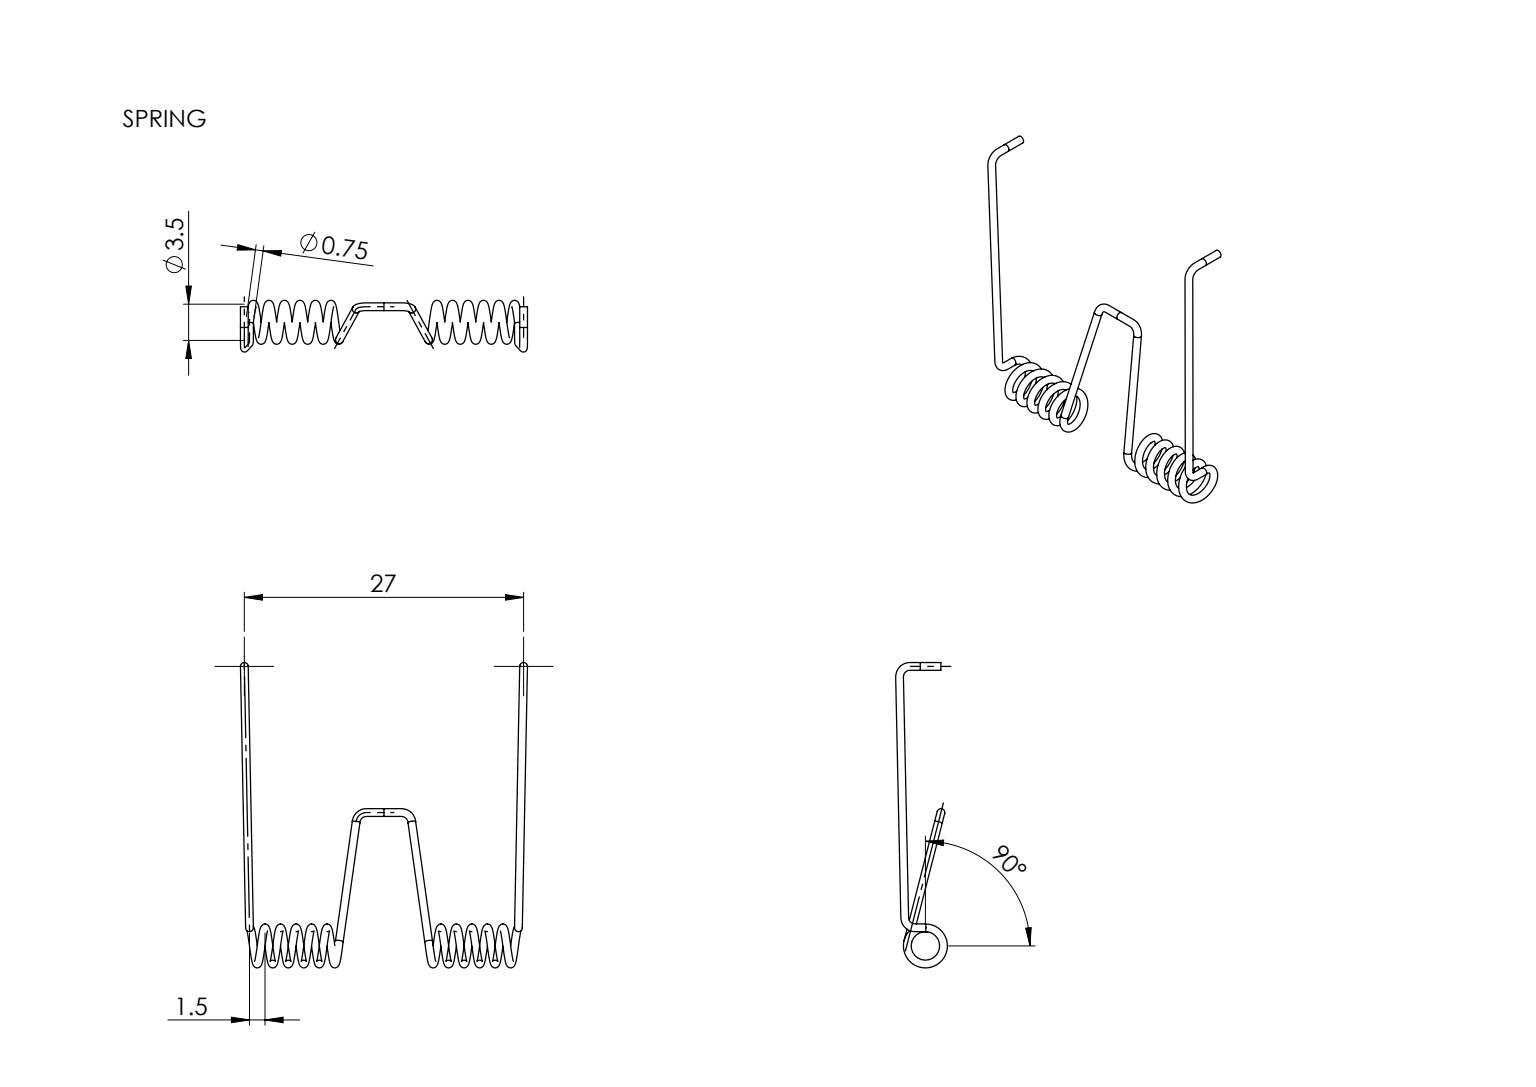
ISO-10303-21;
HEADER;
FILE_DESCRIPTION (('STEP AP214'),
    '1' );
FILE_NAME ('spring.step',
    '2026-10-04T16:38:04',
    ( '' ),
    ( '' ),
    'SwSTEP 2.0',
    'SolidWorks 2026',
    '' );
FILE_SCHEMA (( 'AUTOMOTIVE_DESIGN' ));
ENDSEC;

DATA;
#3=CARTESIAN_POINT ( 'NONE',  ( -13.45643611822145225, -15.38747602984844853, 4.825999963382285429 ) ) ;
#4=CARTESIAN_POINT ( 'NONE',  ( 8.871558582316794173, -20.24999999999999289, 3.449312527122348371 ) ) ;
#5=CARTESIAN_POINT ( 'NONE',  ( -12.62499963760179256, -21.00001830110826972, 4.442557003548452066 ) ) ;
#9=CARTESIAN_POINT ( 'NONE',  ( -8.309058582316795949, -23.80360840875935935, 1.768074502826626260 ) ) ;
#10=CARTESIAN_POINT ( 'NONE',  ( 8.496558582316794173, -22.05068747287764452, 1.749999999999998446 ) ) ;
#11=CARTESIAN_POINT ( 'NONE',  ( 4.097191417683177406, -22.46490103525075810, 4.479004561291653808 ) ) ;
#12=CARTESIAN_POINT ( 'NONE',  ( -6.621558582316794173, -23.74999999999999645, 3.550687472877651629 ) ) ;
#14=CARTESIAN_POINT ( 'NONE',  ( 13.82092246150448211, 3.019084305971233562, 5.221833296715730377 ) ) ;
#25=CARTESIAN_POINT ( 'NONE',  ( -1.548630333695928396, -9.114917468222230923, 2.372643865078341019 ) ) ;
#28=CARTESIAN_POINT ( 'NONE',  ( 2.506848361495492394, -9.459347215042898327, 1.711100304737409150 ) ) ;
#29=CARTESIAN_POINT ( 'NONE',  ( -13.10012427866737639, 3.743776072700027324, 6.001983176248468332 ) ) ;
#30=CARTESIAN_POINT ( 'NONE',  ( 9.715308582316794173, -23.77099543870833998, 2.825813738724734847 ) ) ;
#32=CARTESIAN_POINT ( 'NONE',  ( 13.15498530132288479, 5.764257716805535559, 4.666666666666618113 ) ) ;
#33=CARTESIAN_POINT ( 'NONE',  ( -1.797685059409938280, -9.880079706704160358, 1.626537830816663588 ) ) ;
#37=CARTESIAN_POINT ( 'NONE',  ( -13.85980676119184629, 4.232741440188380722, 5.965367510457697975 ) ) ;
#40=CARTESIAN_POINT ( 'NONE',  ( 5.972191417683178294, -24.47900456129165292, 2.413778621189595963 ) ) ;
#41=CARTESIAN_POINT ( 'NONE',  ( -6.534691417683177406, -20.97900456129164581, 3.136473910504570917 ) ) ;
#44=CARTESIAN_POINT ( 'NONE',  ( 13.90439735423812273, 5.734566389025032684, 4.166666666666765551 ) ) ;
#45=CARTESIAN_POINT ( 'NONE',  ( 13.11017182064853159, 4.251176942750957366, 5.979809059808775196 ) ) ;
#57=CARTESIAN_POINT ( 'NONE',  ( 2.097836924194969033, -11.64739567274323129, 2.830419876579102212 ) ) ;
#64=CARTESIAN_POINT ( 'NONE',  ( 11.77780858231679595, -21.02099543870833998, 3.035098964749253003 ) ) ;
#65=CARTESIAN_POINT ( 'NONE',  ( -13.08799567112409790, 3.881281391764801025, 5.254907606674271037 ) ) ;
#66=CARTESIAN_POINT ( 'NONE',  ( -5.309058582316795949, -22.74294823697954016, 2.828734674606448785 ) ) ;
#67=CARTESIAN_POINT ( 'NONE',  ( -12.25344141768317741, -21.94931252712233061, 1.749999999999998446 ) ) ;
#69=CARTESIAN_POINT ( 'NONE',  ( 13.09358652029869141, 4.163619275088517035, 5.207983256689002083 ) ) ;
#70=SURFACE_STYLE_USAGE ( .BOTH. , #17121 ) ;
#75=CARTESIAN_POINT ( 'NONE',  ( 13.37505392270939986, -20.99727690317663686, 4.612442573673130930 ) ) ;
#79=CARTESIAN_POINT ( 'NONE',  ( 10.19094141768317563, -23.27327832286946219, 4.701595411283453707 ) ) ;
#83=CARTESIAN_POINT ( 'NONE',  ( -2.583953725994688533, -9.847075946378776479, 2.560676788604062004 ) ) ;
#84=CARTESIAN_POINT ( 'NONE',  ( 2.702705060698113115, -10.69015907548275379, 2.777197378435510622 ) ) ;
#85=CARTESIAN_POINT ( 'NONE',  ( -10.65280858231679240, -21.22443879296942626, 5.229004561291660025 ) ) ;
#86=VECTOR ( 'NONE', #19310, 1000.000000000000114 ) ;
#88=CARTESIAN_POINT ( 'NONE',  ( 5.503441417683177406, -22.05068747287766229, 6.000000000000001776 ) ) ;
#90=CARTESIAN_POINT ( 'NONE',  ( -3.974842109207561425, -21.82955800590261575, 5.256404853634145447 ) ) ;
#92=CARTESIAN_POINT ( 'NONE',  ( 13.37155858231679595, -19.49999999999998934, 3.449312527122348371 ) ) ;
#94=CARTESIAN_POINT ( 'NONE',  ( -13.90439735423812273, 5.734566389025032684, 4.791666666666684726 ) ) ;
#97=CARTESIAN_POINT ( 'NONE',  ( 7.465308582316795061, -20.22900456129164937, 4.174186261275266929 ) ) ;
#105=CARTESIAN_POINT ( 'NONE',  ( -12.43405858231679595, -23.73192549717337130, 5.303608408759367343 ) ) ;
#106=CARTESIAN_POINT ( 'NONE',  ( 12.62499979224180180, -20.25001049178813162, 4.458178821399696012 ) ) ;
#108=CARTESIAN_POINT ( 'NONE',  ( 0.5631383031621635116, -9.114917468222230923, 1.622643865078341463 ) ) ;
#109=CARTESIAN_POINT ( 'NONE',  ( 12.62499999999998579, -20.24999999999999289, 3.666666666666653640 ) ) ;
#111=CARTESIAN_POINT ( 'NONE',  ( -13.37499999999998579, -20.24999999999999289, 3.146526952850934755 ) ) ;
#112=CARTESIAN_POINT ( 'NONE',  ( 7.840308582316794173, -22.67418626127525982, 5.270995438708342640 ) ) ;
#113=CARTESIAN_POINT ( 'NONE',  ( -13.89992416064626646, 5.508670112635706495, 5.888743936161951353 ) ) ;
#116=CARTESIAN_POINT ( 'NONE',  ( -10.74655858231679595, -21.94931252712234127, 6.000000000000001776 ) ) ;
#117=CARTESIAN_POINT ( 'NONE',  ( 4.840308582316793284, -22.67418626127525982, 5.270995438708342640 ) ) ;
#119=CARTESIAN_POINT ( 'NONE',  ( 8.503441417683177406, -22.05068747287766229, 4.499999999999999112 ) ) ;
#120=CARTESIAN_POINT ( 'NONE',  ( -9.815941417683177406, -20.79840458871654363, 4.773278322869464851 ) ) ;
#123=CARTESIAN_POINT ( 'NONE',  ( 13.80173896975277437, 2.050317972508536535, 5.200999963382010094 ) ) ;
#125=CARTESIAN_POINT ( 'NONE',  ( 2.693754455098655409, -10.04853567022903782, 2.237415670251142519 ) ) ;
#132=CARTESIAN_POINT ( 'NONE',  ( -2.076833265075072266, -8.407161531158021006, 2.383492984350220389 ) ) ;
#133=CARTESIAN_POINT ( 'NONE',  ( 0.2815691515810352930, -9.114917468222230923, 2.372643865078523984 ) ) ;
#135=CARTESIAN_POINT ( 'NONE',  ( -13.09532840572934376, 3.501584489333809724, 5.996774842915142401 ) ) ;
#138=CARTESIAN_POINT ( 'NONE',  ( 13.12175473207386922, 4.086113969730903683, 6.756475741440692850 ) ) ;
#139=CARTESIAN_POINT ( 'NONE',  ( -1.982945319006538032, -10.83166796549307520, 2.620924705558935308 ) ) ;
#141=CARTESIAN_POINT ( 'NONE',  ( -13.37499999998404299, -20.99999999996810729, 2.793053905886972998 ) ) ;
#143=CARTESIAN_POINT ( 'NONE',  ( 5.878441417683177406, -24.50000000000000000, 3.449312527122335048 ) ) ;
#144=CARTESIAN_POINT ( 'NONE',  ( -6.809058582316796837, -22.74294823697954016, 2.828734674606448785 ) ) ;
#146=CARTESIAN_POINT ( 'NONE',  ( 12.62608183053121458, -20.94536755816881168, 4.949360998036265613 ) ) ;
#147=CARTESIAN_POINT ( 'NONE',  ( 13.10557919622060652, 4.019249409169220577, 6.007898877577752650 ) ) ;
#158=CARTESIAN_POINT ( 'NONE',  ( 0.2815691515810352374, -9.864917468222230923, 1.622643865078524428 ) ) ;
#163=CARTESIAN_POINT ( 'NONE',  ( -11.12155858231679417, -23.74999999999999645, 3.550687472877651629 ) ) ;
#164=CARTESIAN_POINT ( 'NONE',  ( -13.09734501894798342, -20.62502179913553846, 3.486720336327766567 ) ) ;
#165=CARTESIAN_POINT ( 'NONE',  ( -13.08559773465513487, 3.760185600081874746, 5.252303440007609403 ) ) ;
#166=CARTESIAN_POINT ( 'NONE',  ( -10.84030858231679240, -22.67418626127525982, 5.270995438708342640 ) ) ;
#167=CARTESIAN_POINT ( 'NONE',  ( -8.784691417683177406, -23.77099543870834353, 4.174186261275252718 ) ) ;
#169=CARTESIAN_POINT ( 'NONE',  ( 13.37893135632597819, -19.30146650553847465, 4.738802066438188909 ) ) ;
#178=CARTESIAN_POINT ( 'NONE',  ( 9.628441417683177406, -20.24999999999999289, 3.550687472877664952 ) ) ;
#181=CARTESIAN_POINT ( 'NONE',  ( -1.710927537542899612, -9.866086492083725901, 2.372944093759576933 ) ) ;
#182=CARTESIAN_POINT ( 'NONE',  ( 2.659620708751979645, -10.38426118526329489, 2.698636689302993830 ) ) ;
#183=CARTESIAN_POINT ( 'NONE',  ( -11.87155858231679417, -20.24999999999999289, 3.449312527122348371 ) ) ;
#186=CARTESIAN_POINT ( 'NONE',  ( 7.190941417683176518, -23.27327832286946219, 4.701595411283453707 ) ) ;
#188=CARTESIAN_POINT ( 'NONE',  ( -6.253441417683176518, -21.94931252712233061, 1.749999999999998446 ) ) ;
#190=CARTESIAN_POINT ( 'NONE',  ( 11.30905858231679595, -23.80360840875935935, 1.768074502826626260 ) ) ;
#191=CARTESIAN_POINT ( 'NONE',  ( 12.64387510712649565, -19.29680709011273976, 5.506486987317513737 ) ) ;
#192=CARTESIAN_POINT ( 'NONE',  ( -12.62562019941893432, -20.21867992933967173, 4.757612834768309540 ) ) ;
#199=SHAPE_DEFINITION_REPRESENTATION ( #15847, #6045 ) ;
#203=CARTESIAN_POINT ( 'NONE',  ( -7.277808582316794173, -20.27099543870833642, 2.724438792969431589 ) ) ;
#206=CARTESIAN_POINT ( 'NONE',  ( 2.022757268986824730, -10.07035769906783784, 1.675405020440470238 ) ) ;
#207=CARTESIAN_POINT ( 'NONE',  ( 12.65410809543883985, -18.78004118034163739, 5.517608176248461227 ) ) ;
#209=CARTESIAN_POINT ( 'NONE',  ( -13.39169183355864590, -18.65706240528901105, 4.755687463382285429 ) ) ;
#210=CARTESIAN_POINT ( 'NONE',  ( 8.777808582316797725, -19.52099543870833642, 2.413778621189609286 ) ) ;
#211=CARTESIAN_POINT ( 'NONE',  ( -12.62500000000001954, -20.24999999999450040, 3.833333333368183382 ) ) ;
#213=CARTESIAN_POINT ( 'NONE',  ( 5.215308582316793284, -23.77099543870833998, 2.825813738724734847 ) ) ;
#214=CARTESIAN_POINT ( 'NONE',  ( 4.565941417683176518, -22.67126532539353789, 2.757051763020445634 ) ) ;
#215=CARTESIAN_POINT ( 'NONE',  ( -5.409691417683177406, -21.32581373872474373, 5.270995438708348857 ) ) ;
#218=CARTESIAN_POINT ( 'NONE',  ( 13.82811627091129836, 3.382371681020614584, 5.229645796715683304 ) ) ;
#224=CARTESIAN_POINT ( 'NONE',  ( -13.12529397354238192, 5.014845663890295846, 4.833333333333344584 ) ) ;
#225=CARTESIAN_POINT ( 'NONE',  ( -1.513434189748285918, -8.364917468222230923, 1.622643865078341907 ) ) ;
#229=CARTESIAN_POINT ( 'NONE',  ( -12.64323021897839006, -19.32937394158751943, 5.504219675487169283 ) ) ;
#232=CARTESIAN_POINT ( 'NONE',  ( 12.70700162295422864, -16.85891804079483691, 6.308954579156044851 ) ) ;
#233=CARTESIAN_POINT ( 'NONE',  ( -2.097836924194969033, -11.64739567274323129, 2.830419876579102212 ) ) ;
#236=CARTESIAN_POINT ( 'NONE',  ( -13.70116456325478893, -3.778689555664588973, 5.825679699621801433 ) ) ;
#238=CARTESIAN_POINT ( 'NONE',  ( 6.534691417683177406, -19.47900456129164581, 2.515153566944927199 ) ) ;
#239=CARTESIAN_POINT ( 'NONE',  ( -5.027808582316795949, -22.97900456129165647, 3.964901035250747885 ) ) ;
#241=CARTESIAN_POINT ( 'NONE',  ( 13.87372783958217681, 4.185755898898970706, 6.732634959205082481 ) ) ;
#242=CARTESIAN_POINT ( 'NONE',  ( 12.95145221759166354, -3.764163011652346569, 5.840524842913703552 ) ) ;
#249=DIRECTION ( 'NONE',  ( 0.000000000000000000, 0.2487476929738665354, 0.9685683172808094987 ) ) ;
#250=CARTESIAN_POINT ( 'NONE',  ( 1.337453470010121714, -9.864917468222230923, 1.622643865078341907 ) ) ;
#257=CARTESIAN_POINT ( 'NONE',  ( -10.84030858231679240, -22.67418626127525982, 5.270995438708342640 ) ) ;
#258=CARTESIAN_POINT ( 'NONE',  ( -1.548630333695928396, -9.114917468222230923, 2.372643865078341019 ) ) ;
#260=CARTESIAN_POINT ( 'NONE',  ( -12.62837453896009876, -19.32958578251692572, 4.742959489302074338 ) ) ;
#261=CARTESIAN_POINT ( 'NONE',  ( -6.059058582316795949, -21.25705176302045274, 4.171265325393551215 ) ) ;
#262=CARTESIAN_POINT ( 'NONE',  ( -4.284691417683176518, -23.77099543870834353, 4.174186261275252718 ) ) ;
#265=CARTESIAN_POINT ( 'NONE',  ( 13.80173896975277437, 2.050317972508536535, 5.200999963382010094 ) ) ;
#275=CARTESIAN_POINT ( 'NONE',  ( 9.815941417683177406, -20.79840458871654363, 4.773278322869464851 ) ) ;
#277=CARTESIAN_POINT ( 'NONE',  ( -1.853238653218509890, -9.965882697426144077, 2.398573752920997837 ) ) ;
#279=CARTESIAN_POINT ( 'NONE',  ( -9.340308582316794173, -22.67418626127525982, 5.270995438708342640 ) ) ;
#284=CARTESIAN_POINT ( 'NONE',  ( 10.56594141768317741, -23.20159541128344927, 2.226721677130534705 ) ) ;
#286=CARTESIAN_POINT ( 'NONE',  ( -11.59719141768317741, -22.46490103525075810, 4.479004561291653808 ) ) ;
#288=CARTESIAN_POINT ( 'NONE',  ( 11.68405858231679595, -20.26807450282662160, 1.696391591240633101 ) ) ;
#290=CARTESIAN_POINT ( 'NONE',  ( 12.64131715375063258, -19.42598373559290792, 5.491151580003103660 ) ) ;
#291=CARTESIAN_POINT ( 'NONE',  ( -13.15498530132288479, 5.764257716805535559, 4.791666666666684726 ) ) ;
#299=PRESENTATION_STYLE_ASSIGNMENT (( #17872 ) ) ;
#300=ORIENTED_EDGE ( 'NONE', *, *, #6043, .F. ) ;
#303=CARTESIAN_POINT ( 'NONE',  ( 12.87800906051949390, -19.89203723036131066, 3.516308674092069708 ) ) ;
#307=CARTESIAN_POINT ( 'NONE',  ( -6.809058582316794173, -23.27327832286945153, 2.298404588716537411 ) ) ;
#308=CARTESIAN_POINT ( 'NONE',  ( 13.12463908936614132, 4.981774012991869505, 5.264611377988129171 ) ) ;
#311=CARTESIAN_POINT ( 'NONE',  ( 12.62499999999998401, -20.24999999999998934, 2.439580858552613751 ) ) ;
#313=CARTESIAN_POINT ( 'NONE',  ( -13.53317008522746434, -11.51241069598931510, 4.909333296715523431 ) ) ;
#316=CARTESIAN_POINT ( 'NONE',  ( 7.559058582316795949, -20.19639159124062999, 5.231925497173373074 ) ) ;
#317=CARTESIAN_POINT ( 'NONE',  ( -13.15498530132288479, 5.764257716805535559, 3.666666666666500873 ) ) ;
#318=CARTESIAN_POINT ( 'NONE',  ( -10.00344141768317741, -22.05068747287766229, 6.000000000000001776 ) ) ;
#322=CARTESIAN_POINT ( 'NONE',  ( 10.93405858231679595, -22.67126532539354855, 4.242948236979545484 ) ) ;
#323=CARTESIAN_POINT ( 'NONE',  ( -6.722191417683176518, -20.27099543870833998, 4.275561207030583510 ) ) ;
#326=CARTESIAN_POINT ( 'NONE',  ( 13.37883250981221472, -20.05645825448334563, 5.102688967256983510 ) ) ;
#334=CARTESIAN_POINT ( 'NONE',  ( 13.66279757975024722, -5.716222222589476765, 5.784013032957989964 ) ) ;
#341=CARTESIAN_POINT ( 'NONE',  ( -13.10756170493883310, 4.119366099410778581, 6.001761809183453700 ) ) ;
#342=CARTESIAN_POINT ( 'NONE',  ( 5.309058582316794173, -23.27327832286945153, 2.298404588716537411 ) ) ;
#344=CARTESIAN_POINT ( 'NONE',  ( 12.65650603190776025, -18.65894538865861563, 5.520212342915047365 ) ) ;
#345=CARTESIAN_POINT ( 'NONE',  ( -0.2815691515810352374, -9.864917468222230923, 2.372643865078523540 ) ) ;
#347=CARTESIAN_POINT ( 'NONE',  ( -13.39902456816392906, -19.03675930772010361, 5.497554699623231400 ) ) ;
#349=CARTESIAN_POINT ( 'NONE',  ( 10.09719141768317741, -22.77556120703057729, 5.229004561291655584 ) ) ;
#350=CARTESIAN_POINT ( 'NONE',  ( -7.371558582316795949, -20.99999999999999645, 3.449312527122348371 ) ) ;
#352=CARTESIAN_POINT ( 'NONE',  ( 13.87486364728600208, 4.243114187942282456, 6.725269602253773016 ) ) ;
#353=CARTESIAN_POINT ( 'NONE',  ( 12.66849571425264287, -18.05346643024382303, 5.533233176248494978 ) ) ;
#364=CARTESIAN_POINT ( 'NONE',  ( 1.711347482507859397, -9.865394108634699677, 1.622766275858107621 ) ) ;
#371=CARTESIAN_POINT ( 'NONE',  ( -9.059058582316794173, -20.72672167713054137, 4.701595411283463477 ) ) ;
#373=CARTESIAN_POINT ( 'NONE',  ( -0.5631383031621635116, -9.114917468222230923, 2.372643865078341019 ) ) ;
#375=CARTESIAN_POINT ( 'NONE',  ( -12.62499994688180749, -19.50000268246798640, 4.473800639250938183 ) ) ;
#376=CARTESIAN_POINT ( 'NONE',  ( -10.37155858231679417, -20.24999999999999289, 3.449312527122348371 ) ) ;
#377=CARTESIAN_POINT ( 'NONE',  ( -7.284691417683176518, -23.77099543870834353, 4.174186261275252718 ) ) ;
#379=CARTESIAN_POINT ( 'NONE',  ( 13.37930517931174634, -19.28258844475809042, 4.742233558278135419 ) ) ;
#389=CARTESIAN_POINT ( 'NONE',  ( 6.909691417683177406, -21.32581373872474373, 5.270995438708348857 ) ) ;
#391=CARTESIAN_POINT ( 'NONE',  ( -1.707060460004204527, -9.864918773552613374, 2.372644200313257290 ) ) ;
#393=CARTESIAN_POINT ( 'NONE',  ( -7.840308582316794173, -22.67418626127525982, 5.270995438708342640 ) ) ;
#395=CARTESIAN_POINT ( 'NONE',  ( 8.690941417683177406, -23.27327832286946219, 4.701595411283453707 ) ) ;
#397=CARTESIAN_POINT ( 'NONE',  ( -10.47219141768317741, -22.97900456129165292, 3.035098964749240125 ) ) ;
#400=CARTESIAN_POINT ( 'NONE',  ( 9.621558582316795949, -24.50000000000000000, 3.550687472877651629 ) ) ;
#401=CARTESIAN_POINT ( 'NONE',  ( 13.09532840572934376, 3.501584489333809724, 5.996774842915142401 ) ) ;
#402=CARTESIAN_POINT ( 'NONE',  ( -13.15498530132288479, 5.764257716805535559, 4.333333333333380999 ) ) ;
#410=CARTESIAN_POINT ( 'NONE',  ( 13.24164500767265729, -19.96139048183125198, 3.467035629977988975 ) ) ;
#414=CARTESIAN_POINT ( 'NONE',  ( 13.05696142222617695, 1.564051822406025583, 5.955108176248398166 ) ) ;
#418=CARTESIAN_POINT ( 'NONE',  ( 13.15498501280115917, 5.764243146453090105, 5.045733045595949484 ) ) ;
#419=CARTESIAN_POINT ( 'NONE',  ( 4.315753587183824180, -21.65797192216093947, 4.831781436261117335 ) ) ;
#420=CARTESIAN_POINT ( 'NONE',  ( -13.37499979530394967, -20.25001033714808329, 4.458488164327452097 ) ) ;
#421=CARTESIAN_POINT ( 'NONE',  ( 9.715308582316795949, -24.52099543870834708, 2.515153566944913432 ) ) ;
#423=CARTESIAN_POINT ( 'NONE',  ( -13.14123030749026277, 5.069630528265579805, 6.418963484850015000 ) ) ;
#424=CARTESIAN_POINT ( 'NONE',  ( -12.44094141768317741, -20.19639159124061933, 1.768074502826635586 ) ) ;
#426=CARTESIAN_POINT ( 'NONE',  ( 3.944195004867014909, -21.61378581760806128, 5.207602947182413011 ) ) ;
#428=CARTESIAN_POINT ( 'NONE',  ( 10.84030858231679595, -22.36352608949544418, 4.520995438708343528 ) ) ;
#429=CARTESIAN_POINT ( 'NONE',  ( -7.284691417683176518, -23.77099543870834353, 4.174186261275251830 ) ) ;
#432=CARTESIAN_POINT ( 'NONE',  ( 13.84501469867711698, 4.235742283194553259, 4.791666666666684726 ) ) ;
#436=ADVANCED_FACE ( 'NONE', ( #18652 ), #4141, .F. ) ;
#439=CARTESIAN_POINT ( 'NONE',  ( 13.84983662433050178, 3.729249528687784920, 5.987138032956566214 ) ) ;
#441=CARTESIAN_POINT ( 'NONE',  ( 3.767139617958116471, -12.99583330722436791, 3.561955564372631500 ) ) ;
#444=CARTESIAN_POINT ( 'NONE',  ( -12.62746768552656285, -19.37538188090202596, 4.723115281690125400 ) ) ;
#445=CARTESIAN_POINT ( 'NONE',  ( 8.496558582316794173, -22.05068747287764452, 1.749999999999998446 ) ) ;
#447=CARTESIAN_POINT ( 'NONE',  ( 13.08573665985359824, 3.017201322601628100, 5.986358176248492313 ) ) ;
#449=CARTESIAN_POINT ( 'NONE',  ( -2.875042468481914248, -11.91375063635796039, 3.091440134965714126 ) ) ;
#450=CARTESIAN_POINT ( 'NONE',  ( 10.55905858231679595, -21.25705176302045274, 4.171265325393551215 ) ) ;
#451=CARTESIAN_POINT ( 'NONE',  ( 9.628441417683177406, -20.24999999999999289, 3.550687472877664952 ) ) ;
#453=CARTESIAN_POINT ( 'NONE',  ( -7.090308582316795061, -21.63647391050454871, 2.479004561291657804 ) ) ;
#455=CARTESIAN_POINT ( 'NONE',  ( 13.88045627189955233, 4.525541730927888473, 6.662882075361062029 ) ) ;
#456=CARTESIAN_POINT ( 'NONE',  ( 13.10372118337080849, 3.925419760224517329, 6.005889426248455010 ) ) ;
#468=CARTESIAN_POINT ( 'NONE',  ( 0.000000000000000000, -9.114917468222230923, 1.622643865078341019 ) ) ;
#472=CARTESIAN_POINT ( 'NONE',  ( 13.36732475835166234, -20.34061592879088920, 3.450098321863545703 ) ) ;
#473=CARTESIAN_POINT ( 'NONE',  ( -2.436080212393455735, -9.483920418190111334, 2.467411194204634839 ) ) ;
#474=CARTESIAN_POINT ( 'NONE',  ( -8.871558582316794173, -20.24999999999999289, 3.449312527122348371 ) ) ;
#475=CARTESIAN_POINT ( 'NONE',  ( -3.034277558025862298, -9.029550313327863620, 2.543334857076493094 ) ) ;
#477=CARTESIAN_POINT ( 'NONE',  ( -12.62506359033936754, -19.49678868786235597, 4.541393094775662220 ) ) ;
#478=CARTESIAN_POINT ( 'NONE',  ( -5.871558582316794173, -20.24999999999999289, 3.449312527122348371 ) ) ;
#479=CARTESIAN_POINT ( 'NONE',  ( -5.972191417683179182, -23.72900456129165292, 2.724438792969417822 ) ) ;
#481=CARTESIAN_POINT ( 'NONE',  ( 13.84485691484488257, 4.227774199669918964, 5.063753864839139140 ) ) ;
#488=CARTESIAN_POINT ( 'NONE',  ( 5.690941417683176518, -23.27327832286946219, 4.701595411283453707 ) ) ;
#492=EDGE_CURVE ( 'NONE', #1847, #19275, #12685, .T. ) ;
#494=CARTESIAN_POINT ( 'NONE',  ( 11.03469141768318273, -20.22900456129164581, 2.825813738724747726 ) ) ;
#496=CARTESIAN_POINT ( 'NONE',  ( -8.878441417683177406, -22.99999999999999645, 3.449312527122335048 ) ) ;
#497=CARTESIAN_POINT ( 'NONE',  ( -8.965308582316795949, -19.47900456129164937, 4.484846433055089676 ) ) ;
#499=CARTESIAN_POINT ( 'NONE',  ( 12.62499999998404121, -20.24999999996810729, 2.793053905886972998 ) ) ;
#500=CARTESIAN_POINT ( 'NONE',  ( -13.15469878640066526, 5.749788713235649773, 5.232478742873432509 ) ) ;
#507=CARTESIAN_POINT ( 'NONE',  ( 2.592143777221601386, -9.905122062175031772, 2.575584190728205325 ) ) ;
#512=CARTESIAN_POINT ( 'NONE',  ( 13.12529380813666435, 5.014837310896125722, 5.033295791462342628 ) ) ;
#515=CARTESIAN_POINT ( 'NONE',  ( 12.91308523408712183, -5.701695678577235249, 5.798858176249892082 ) ) ;
#517=CARTESIAN_POINT ( 'NONE',  ( 7.184058582316795949, -20.26807450282662160, 1.696391591240633101 ) ) ;
#518=CARTESIAN_POINT ( 'NONE',  ( -13.15498530132288479, 5.764257716805535559, 4.166666666666765551 ) ) ;
#519=CARTESIAN_POINT ( 'NONE',  ( -4.687312169500634340, -21.32903648725300272, 5.908812401261035241 ) ) ;
#524=CARTESIAN_POINT ( 'NONE',  ( 8.309058582316795949, -22.74294823697954016, 2.828734674606448785 ) ) ;
#529=CARTESIAN_POINT ( 'NONE',  ( 13.39542766346049518, -19.21840299524461315, 5.493648449623241170 ) ) ;
#536=CARTESIAN_POINT ( 'NONE',  ( 13.83544900551672185, 3.002674778589386140, 5.971513032956590195 ) ) ;
#539=CARTESIAN_POINT ( 'NONE',  ( 1.797604806073912709, -9.120796646272857799, 2.374153755450133740 ) ) ;
#540=CARTESIAN_POINT ( 'NONE',  ( 1.652577328807104839, -9.114908150887895744, 1.622641472200749835 ) ) ;
#541=CARTESIAN_POINT ( 'NONE',  ( -12.93692567357942202, -3.747753484270499591, 5.090845106672844622 ) ) ;
#542=CARTESIAN_POINT ( 'NONE',  ( 7.840308582316794173, -22.67418626127525982, 5.270995438708342640 ) ) ;
#544=CARTESIAN_POINT ( 'NONE',  ( 13.11514659413808737, 4.502403003978772134, 5.887634658581065494 ) ) ;
#546=CARTESIAN_POINT ( 'NONE',  ( -1.548630333695928396, -9.114917468222230923, 2.372643865078341019 ) ) ;
#547=CARTESIAN_POINT ( 'NONE',  ( 6.902808582316795949, -22.46490103525074034, 2.520995438708341307 ) ) ;
#549=CARTESIAN_POINT ( 'NONE',  ( 8.128441417683175629, -20.24999999999999289, 3.550687472877664952 ) ) ;
#550=CARTESIAN_POINT ( 'NONE',  ( -10.18405858231679595, -21.32873467460644079, 2.757051763020455404 ) ) ;
#552=CARTESIAN_POINT ( 'NONE',  ( 13.11345185444515415, 3.666818649476655700, 6.750360829155977349 ) ) ;
#554=CARTESIAN_POINT ( 'NONE',  ( 13.09123688038123490, 4.044962459253448550, 5.255034774807352704 ) ) ;
#563=CARTESIAN_POINT ( 'NONE',  ( 3.277163086644854229, -14.76879761173520578, 3.824673233536266537 ) ) ;
#564=LINE ( 'NONE', #11752, #7741 ) ;
#569=CARTESIAN_POINT ( 'NONE',  ( -9.246558582316794173, -21.94931252712234482, 5.250000000000000888 ) ) ;
#571=CARTESIAN_POINT ( 'NONE',  ( -3.451187703687236041, -10.75258211228477734, 2.985843844067104680 ) ) ;
#573=CARTESIAN_POINT ( 'NONE',  ( -13.09560269887985307, 4.265436293439658577, 4.973800642626965640 ) ) ;
#575=CARTESIAN_POINT ( 'NONE',  ( -5.409691417683178294, -21.32581373872474373, 5.270995438708348857 ) ) ;
#577=CARTESIAN_POINT ( 'NONE',  ( 13.39169183355864590, -18.65706240528901105, 4.755687463382285429 ) ) ;
#589=CARTESIAN_POINT ( 'NONE',  ( 1.728780693989796724, -8.364929292255887106, 2.372646901726390478 ) ) ;
#590=CARTESIAN_POINT ( 'NONE',  ( -5.965308582316793284, -20.22900456129164937, 4.174186261275266929 ) ) ;
#592=CARTESIAN_POINT ( 'NONE',  ( 12.66863463945108137, -18.79645070772368953, 6.267287912489321045 ) ) ;
#595=CARTESIAN_POINT ( 'NONE',  ( 4.284691417683176518, -23.77099543870834353, 4.174186261275252718 ) ) ;
#597=CARTESIAN_POINT ( 'NONE',  ( -9.628441417683177406, -20.99999999999999645, 3.550687472877664952 ) ) ;
#598=CARTESIAN_POINT ( 'NONE',  ( -6.434058582316796837, -23.73192549717337130, 5.303608408759367343 ) ) ;
#600=CARTESIAN_POINT ( 'NONE',  ( 12.79798428357658047, -11.51429367935891790, 5.673858176248284479 ) ) ;
#601=CARTESIAN_POINT ( 'NONE',  ( -13.11345185444515415, 3.666818649476655700, 6.750360829155977349 ) ) ;
#602=ORIENTED_EDGE ( 'NONE', *, *, #19126, .F. ) ;
#609=CARTESIAN_POINT ( 'NONE',  ( 12.79327455738548203, -19.93647458090189772, 3.527980527292456259 ) ) ;
#612=CARTESIAN_POINT ( 'NONE',  ( 0.000000000000000000, -9.114917468222230923, 1.622643865078341019 ) ) ;
#614=CARTESIAN_POINT ( 'NONE',  ( -1.960495238260606010, -8.383787449798761671, 1.627490053312942164 ) ) ;
#619=CARTESIAN_POINT ( 'NONE',  ( 9.527808582316795949, -24.47900456129166358, 4.586221378810390270 ) ) ;
#620=CARTESIAN_POINT ( 'NONE',  ( -13.12405442816082868, 4.202248622120948518, 6.747400073346936367 ) ) ;
#621=CARTESIAN_POINT ( 'NONE',  ( -7.472191417683177406, -24.47900456129165292, 2.413778621189595963 ) ) ;
#626=CARTESIAN_POINT ( 'NONE',  ( 6.996558582316795949, -22.05068747287764452, 2.499999999999999112 ) ) ;
#631=CARTESIAN_POINT ( 'NONE',  ( 13.49014615398506045, -14.43511922376608680, 5.596513032956658584 ) ) ;
#638=CARTESIAN_POINT ( 'NONE',  ( 13.37515323800563039, -20.24226148071262799, 4.627790572011877934 ) ) ;
#641=CARTESIAN_POINT ( 'NONE',  ( 0.000000000000000000, -8.364917468222230923, 2.372643865078341019 ) ) ;
#644=CARTESIAN_POINT ( 'NONE',  ( -12.62562661273123332, -19.46835605706984040, 4.628101975944573176 ) ) ;
#645=CARTESIAN_POINT ( 'NONE',  ( 4.840308582316793284, -22.67418626127525982, 5.270995438708342640 ) ) ;
#647=CARTESIAN_POINT ( 'NONE',  ( 12.91308523408712183, -5.701695678577235249, 5.798858176249892082 ) ) ;
#648=CARTESIAN_POINT ( 'NONE',  ( -1.668644041176298387, -9.864915931696323526, 2.372643470467795890 ) ) ;
#649=CARTESIAN_POINT ( 'NONE',  ( 10.74655858231679595, -21.94931252712234127, 4.499999999999999112 ) ) ;
#650=CARTESIAN_POINT ( 'NONE',  ( 11.87844141768317563, -23.74999999999999645, 3.449312527122335492 ) ) ;
#651=CARTESIAN_POINT ( 'NONE',  ( -7.934058582316792396, -23.20159541128345992, 4.773278322869455970 ) ) ;
#653=CARTESIAN_POINT ( 'NONE',  ( 13.12175473207386922, 4.086113969730903683, 6.756475741440692850 ) ) ;
#654=CARTESIAN_POINT ( 'NONE',  ( 12.62500797102436678, -19.49959746326937093, 4.516621614626514791 ) ) ;
#666=CARTESIAN_POINT ( 'NONE',  ( 1.772926875221950249, -9.883376166076789815, 2.377384427436886494 ) ) ;
#674=CARTESIAN_POINT ( 'NONE',  ( -6.809058582316794173, -23.27327832286945153, 2.298404588716537411 ) ) ;
#675=CARTESIAN_POINT ( 'NONE',  ( -3.502569552650398155, -9.961070227720959736, 2.032567780072621400 ) ) ;
#678=CARTESIAN_POINT ( 'NONE',  ( -13.37499999999998224, -19.49999999999998934, 4.166666666666637653 ) ) ;
#679=CARTESIAN_POINT ( 'NONE',  ( -4.840308582316793284, -22.67418626127525982, 5.270995438708342640 ) ) ;
#681=CARTESIAN_POINT ( 'NONE',  ( -11.40969141768317918, -21.63647391050456648, 4.520995438708348857 ) ) ;
#683=CARTESIAN_POINT ( 'NONE',  ( 13.39542766346049518, -19.21840299524461315, 5.493648449623241170 ) ) ;
#689=CARTESIAN_POINT ( 'NONE',  ( -13.37499999999998579, -20.24999999999999289, 3.666666666666653640 ) ) ;
#692=ORIENTED_EDGE ( 'NONE', *, *, #16527, .T. ) ;
#698=CARTESIAN_POINT ( 'NONE',  ( 3.173374397671306912, -9.279487642487616483, 2.607523756204581211 ) ) ;
#699=CARTESIAN_POINT ( 'NONE',  ( -7.371558582316794173, -20.24999999999999289, 3.449312527122348371 ) ) ;
#700=CARTESIAN_POINT ( 'NONE',  ( 12.62927505847832776, -20.78410954684871825, 5.373974324164845662 ) ) ;
#701=B_SPLINE_CURVE_WITH_KNOTS ( 'NONE', 3,
 ( #1316, #14061, #7896, #20471, #12592, #14258 ),
 .UNSPECIFIED., .F., .F.,
 ( 4, 2, 4 ),
 ( 0.5000000000000000000, 0.7500000000000000000, 1.000000000000000000 ),
 .UNSPECIFIED. ) ;
#703=CARTESIAN_POINT ( 'NONE',  ( 4.472191417683177406, -23.72900456129165292, 2.724438792969417822 ) ) ;
#705=CARTESIAN_POINT ( 'NONE',  ( -4.472191417683178294, -22.97900456129165292, 3.035098964749240125 ) ) ;
#706=CARTESIAN_POINT ( 'NONE',  ( -5.590308582316795949, -21.01515356694490322, 0.9790045612916562501 ) ) ;
#708=CARTESIAN_POINT ( 'NONE',  ( 12.62499999999998401, -19.49999999999998934, 3.666666666666654084 ) ) ;
#709=CARTESIAN_POINT ( 'NONE',  ( -13.09532840572934376, 3.501584489333809724, 5.996774842915142401 ) ) ;
#723=CARTESIAN_POINT ( 'NONE',  ( 13.08094078691552831, 2.775009739235173356, 5.981149842915306714 ) ) ;
#724=CARTESIAN_POINT ( 'NONE',  ( -3.486710468562268961, -9.848741751643258269, 2.003719583429115492 ) ) ;
#730=CARTESIAN_POINT ( 'NONE',  ( 10.00344141768317741, -22.05068747287766229, 6.000000000000001776 ) ) ;
#731=CARTESIAN_POINT ( 'NONE',  ( -12.63465172146706728, -19.76258806590802664, 5.372658420469845986 ) ) ;
#733=CARTESIAN_POINT ( 'NONE',  ( -5.315941417683176518, -20.26807450282663225, 5.303608408759377113 ) ) ;
#737=CARTESIAN_POINT ( 'NONE',  ( -13.77789853026076550, 0.09637577819625635367, 5.909013032956687006 ) ) ;
#738=CARTESIAN_POINT ( 'NONE',  ( 7.465308582316796837, -20.97900456129165647, 3.863526089495444626 ) ) ;
#742=CARTESIAN_POINT ( 'NONE',  ( 13.87444723674697755, 4.972085455720938185, 5.163895512850782410 ) ) ;
#749=CARTESIAN_POINT ( 'NONE',  ( 13.41820805991576826, -18.06799297425606454, 5.518388032956592859 ) ) ;
#751=CARTESIAN_POINT ( 'NONE',  ( 1.957016269584227031, -9.152392576945766578, 2.382268221639079364 ) ) ;
#753=CARTESIAN_POINT ( 'NONE',  ( -12.62499999999998224, -19.50000000000006040, 4.416666666666682062 ) ) ;
#755=CARTESIAN_POINT ( 'NONE',  ( 12.43405858231679417, -23.20159541128345992, 4.773278322869455970 ) ) ;
#756=CARTESIAN_POINT ( 'NONE',  ( -13.79242507427300879, 0.07996625081441015304, 6.658692769197546824 ) ) ;
#760=CARTESIAN_POINT ( 'NONE',  ( 8.215308582316795949, -23.02099543870833998, 3.136473910504556262 ) ) ;
#761=CARTESIAN_POINT ( 'NONE',  ( 8.878441417683177406, -23.74999999999999645, 3.449312527122335492 ) ) ;
#762=CARTESIAN_POINT ( 'NONE',  ( -11.30905858231679417, -23.27327832286945153, 2.298404588716537411 ) ) ;
#763=ORIENTED_EDGE ( 'NONE', *, *, #6414, .F. ) ;
#764=CARTESIAN_POINT ( 'NONE',  ( 12.66204031416134335, -19.12946413485185104, 6.260126454156002218 ) ) ;
#765=CARTESIAN_POINT ( 'NONE',  ( 13.08799567112409790, 3.881281391764801025, 5.254907606674271037 ) ) ;
#774=CARTESIAN_POINT ( 'NONE',  ( 1.824218240560544047, -9.921717538097572842, 2.387231257717697286 ) ) ;
#779=CARTESIAN_POINT ( 'NONE',  ( -4.934058582316793284, -23.20159541128345992, 4.773278322869455970 ) ) ;
#780=CARTESIAN_POINT ( 'NONE',  ( -0.9854920305337622199, -8.364917468222230923, 2.372643865078341019 ) ) ;
#782=CARTESIAN_POINT ( 'NONE',  ( -13.37500000000002132, -19.49999999999450040, 3.833333333368183382 ) ) ;
#783=CARTESIAN_POINT ( 'NONE',  ( -7.652808582316795061, -21.22443879296942626, 5.229004561291659137 ) ) ;
#785=CARTESIAN_POINT ( 'NONE',  ( 11.40280858231679595, -23.08622137881038938, 1.020995438708339309 ) ) ;
#786=CARTESIAN_POINT ( 'NONE',  ( -9.065941417683177406, -22.67126532539353789, 2.757051763020445634 ) ) ;
#788=CARTESIAN_POINT ( 'NONE',  ( 13.37597619100657198, -20.20070235416671167, 4.815535977982682070 ) ) ;
#802=CARTESIAN_POINT ( 'NONE',  ( 0.2815691515810352374, -8.364917468222230923, 2.372643865078523540 ) ) ;
#803=CARTESIAN_POINT ( 'NONE',  ( -8.496558582316794173, -22.05068747287764452, 1.749999999999998446 ) ) ;
#804=CARTESIAN_POINT ( 'NONE',  ( 12.62672826945118665, -20.91272239271162903, 5.058631648758789900 ) ) ;
#806=CARTESIAN_POINT ( 'NONE',  ( 11.59719141768317741, -22.46490103525075810, 4.479004561291653808 ) ) ;
#808=CARTESIAN_POINT ( 'NONE',  ( -4.097191417683177406, -22.46490103525075810, 4.479004561291653808 ) ) ;
#810=CARTESIAN_POINT ( 'NONE',  ( -4.717959273841179524, -21.63341328858655999, 5.993595146365859883 ) ) ;
#812=CARTESIAN_POINT ( 'NONE',  ( 13.11740841389447709, 4.616624901677048420, 5.813473370769506765 ) ) ;
#813=CARTESIAN_POINT ( 'NONE',  ( -13.08094078691552831, 2.775009739235173356, 5.981149842915306714 ) ) ;
#822=CARTESIAN_POINT ( 'NONE',  ( -2.693754455098655409, -10.04853567022903782, 2.237415670251142519 ) ) ;
#824=CARTESIAN_POINT ( 'NONE',  ( -3.506783328160878010, -9.991161114504492957, 2.040295720924476530 ) ) ;
#828=CARTESIAN_POINT ( 'NONE',  ( 6.340308582316796837, -22.98484643305508612, 6.020995438708344416 ) ) ;
#829=CARTESIAN_POINT ( 'NONE',  ( -13.12512971825177033, 5.006550771716304915, 5.133277049491872468 ) ) ;
#830=CARTESIAN_POINT ( 'NONE',  ( -8.972191417683177406, -24.47900456129165292, 2.413778621189595963 ) ) ;
#834=CARTESIAN_POINT ( 'NONE',  ( 12.80905858231679417, -23.27327832286945153, 2.298404588716537411 ) ) ;
#836=CARTESIAN_POINT ( 'NONE',  ( -13.39782821820594627, -19.84717498059871943, 6.143582220458365661 ) ) ;
#837=CARTESIAN_POINT ( 'NONE',  ( 12.99655858231679417, -22.05068747287764452, 1.749999999999998446 ) ) ;
#841=CARTESIAN_POINT ( 'NONE',  ( 13.77789853026076550, 0.09637577819625635367, 5.909013032956687006 ) ) ;
#851=CARTESIAN_POINT ( 'NONE',  ( 3.636036383999129207, -10.90885478516162976, 2.275977788322152584 ) ) ;
#852=CARTESIAN_POINT ( 'NONE',  ( -13.87470602645761808, 4.985154336109792972, 4.000000000000000000 ) ) ;
#853=CARTESIAN_POINT ( 'NONE',  ( -12.65396917024039958, -18.03705690286155772, 4.783553440007634272 ) ) ;
#857=CARTESIAN_POINT ( 'NONE',  ( -13.87470602645761986, 4.985154336109792972, 3.000000000000000000 ) ) ;
#860=CARTESIAN_POINT ( 'NONE',  ( 13.09030858231679417, -21.32581373872472597, 1.729004561291657582 ) ) ;
#861=CARTESIAN_POINT ( 'NONE',  ( 9.159691417683175629, -22.36352608949543352, 2.479004561291652031 ) ) ;
#862=CARTESIAN_POINT ( 'NONE',  ( -9.621558582316794173, -23.74999999999999645, 3.550687472877651629 ) ) ;
#864=CARTESIAN_POINT ( 'NONE',  ( 12.68302225826488616, -18.06987595762608478, 6.282912912489355683 ) ) ;
#865=CARTESIAN_POINT ( 'NONE',  ( 12.82182472306881671, -9.560351485048736109, 4.965845106672846399 ) ) ;
#875=CARTESIAN_POINT ( 'NONE',  ( 1.126276606324276619, -9.864917468222230923, 2.372643865078341019 ) ) ;
#878=CARTESIAN_POINT ( 'NONE',  ( 4.315753587183822404, -21.47141115243053378, 5.558207674221720573 ) ) ;
#879=CARTESIAN_POINT ( 'NONE',  ( -12.71530858231679417, -24.52099543870834708, 2.515153566944913432 ) ) ;
#880=CARTESIAN_POINT ( 'NONE',  ( -1.639793706121975614, -8.364901960018411131, 1.622639882261793343 ) ) ;
#882=CARTESIAN_POINT ( 'NONE',  ( -13.37523871602689596, -19.48794484064217514, 4.577160611493482634 ) ) ;
#883=CARTESIAN_POINT ( 'NONE',  ( -6.434058582316794173, -23.20159541128345992, 4.773278322869455970 ) ) ;
#884=CARTESIAN_POINT ( 'NONE',  ( 7.465308582316796837, -19.47900456129164937, 4.484846433055089676 ) ) ;
#885=CARTESIAN_POINT ( 'NONE',  ( -12.25344141768317741, -21.94931252712233061, 2.499999999999999112 ) ) ;
#887=CARTESIAN_POINT ( 'NONE',  ( 13.70116456325478893, -3.778689555664588973, 5.825679699621801433 ) ) ;
#899=CARTESIAN_POINT ( 'NONE',  ( 1.743623630681728542, -9.116095536440919744, 2.372946416531167557 ) ) ;
#901=CARTESIAN_POINT ( 'NONE',  ( 13.88684657106908205, 4.848251838987907014, 6.535242036940271504 ) ) ;
#904=CARTESIAN_POINT ( 'NONE',  ( 11.97219141768317918, -22.97900456129165292, 3.035098964749240125 ) ) ;
#905=CARTESIAN_POINT ( 'NONE',  ( -12.62503117662529739, -20.24842558042254836, 4.565011198945062354 ) ) ;
#906=CARTESIAN_POINT ( 'NONE',  ( -6.722191417683176518, -21.02099543870834353, 3.964901035250761208 ) ) ;
#907=CARTESIAN_POINT ( 'NONE',  ( -8.503441417683177406, -22.05068747287766229, 6.000000000000001776 ) ) ;
#909=CARTESIAN_POINT ( 'NONE',  ( 12.62933427970994238, -19.28111887465110996, 4.754790882998214840 ) ) ;
#910=CARTESIAN_POINT ( 'NONE',  ( -13.12500000000000178, 5.000000000000047962, 4.000000000000000000 ) ) ;
#916=ORIENTED_EDGE ( 'NONE', *, *, #5151, .T. ) ;
#921=CARTESIAN_POINT ( 'NONE',  ( -3.187906586576829682, -9.105473976199601083, 1.812833570429532859 ) ) ;
#928=CARTESIAN_POINT ( 'NONE',  ( 10.65969141768317741, -22.98484643305507191, 0.9790045612916508100 ) ) ;
#929=CARTESIAN_POINT ( 'NONE',  ( -13.12529397354238192, 5.014845663890295846, 4.833333333333344584 ) ) ;
#931=CARTESIAN_POINT ( 'NONE',  ( -5.597191417683177406, -23.08622137881040359, 5.979004561291654696 ) ) ;
#933=CARTESIAN_POINT ( 'NONE',  ( 10.74655858231679417, -21.94931252712234482, 5.250000000000000888 ) ) ;
#934=CARTESIAN_POINT ( 'NONE',  ( -13.87500000000000178, 5.000000000000047962, 4.000000000000000000 ) ) ;
#935=CARTESIAN_POINT ( 'NONE',  ( -13.43273460392801155, -18.08440250163749496, 6.268067769197452677 ) ) ;
#937=CARTESIAN_POINT ( 'NONE',  ( 12.62155858231679417, -23.74999999999999645, 3.550687472877651629 ) ) ;
#941=CARTESIAN_POINT ( 'NONE',  ( 13.81626551376501588, 2.033908445126689557, 5.950679699622869911 ) ) ;
#947=CARTESIAN_POINT ( 'NONE',  ( -11.59030858231679417, -21.32581373872472597, 1.729004561291657582 ) ) ;
#951=CARTESIAN_POINT ( 'NONE',  ( 3.002445346198714837, -11.66215945560911749, 2.276826493710632171 ) ) ;
#953=CARTESIAN_POINT ( 'NONE',  ( -13.37499999999998224, -19.49999999999998934, 4.166666666666637653 ) ) ;
#955=CARTESIAN_POINT ( 'NONE',  ( -13.37499999999998401, -20.99999999999998934, 2.439580858552613751 ) ) ;
#958=CARTESIAN_POINT ( 'NONE',  ( 5.684058582316795949, -21.32873467460644079, 2.757051763020455404 ) ) ;
#960=CARTESIAN_POINT ( 'NONE',  ( 11.97219141768317918, -22.97900456129165292, 3.035098964749240125 ) ) ;
#961=CARTESIAN_POINT ( 'NONE',  ( -4.687312169500634340, -21.70215802671379990, 4.455959925339818106 ) ) ;
#963=CARTESIAN_POINT ( 'NONE',  ( 13.09106898171683930, 4.036483576700608644, 5.256123545019964816 ) ) ;
#974=CARTESIAN_POINT ( 'NONE',  ( -2.875042468481914248, -11.91375063635796039, 3.091440134965714126 ) ) ;
#975=CARTESIAN_POINT ( 'NONE',  ( -13.84504075139246915, 3.487057945321567765, 5.981929699623240282 ) ) ;
#977=CARTESIAN_POINT ( 'NONE',  ( 1.513434189748285918, -9.864917468222230923, 2.372643865078341019 ) ) ;
#981=CARTESIAN_POINT ( 'NONE',  ( -8.777808582316797725, -19.52099543870833642, 2.413778621189609286 ) ) ;
#982=CARTESIAN_POINT ( 'NONE',  ( -2.512468814886674284, -13.43512376012158782, 2.539544162874482591 ) ) ;
#985=CARTESIAN_POINT ( 'NONE',  ( -13.37499999999998224, -19.49999999999998934, 4.291666666666699825 ) ) ;
#988=CARTESIAN_POINT ( 'NONE',  ( 10.09719141768317741, -23.08622137881040359, 5.979004561291654696 ) ) ;
#989=CARTESIAN_POINT ( 'NONE',  ( -10.56594141768317741, -22.67126532539353789, 2.757051763020445634 ) ) ;
#992=CARTESIAN_POINT ( 'NONE',  ( 13.40022353639839103, -18.97621141187856608, 5.498856782956575984 ) ) ;
#998=CARTESIAN_POINT ( 'NONE',  ( -13.84983662433050178, 3.729249528687784920, 5.987138032956566214 ) ) ;
#1004=CARTESIAN_POINT ( 'NONE',  ( 2.445888733774860935, -8.532121313016713060, 2.415585152653916712 ) ) ;
#1008=CARTESIAN_POINT ( 'NONE',  ( 12.62499999999998401, -20.99999999999998934, 2.439580858552613751 ) ) ;
#1011=CARTESIAN_POINT ( 'NONE',  ( 13.12529397354238192, 5.014845663890295846, 4.791666666666685614 ) ) ;
#1012=CARTESIAN_POINT ( 'NONE',  ( 11.87844141768317741, -22.99999999999999645, 3.449312527122335048 ) ) ;
#1013=CARTESIAN_POINT ( 'NONE',  ( -12.62562019941893432, -20.21867992933967173, 4.757612834768309540 ) ) ;
#1014=CARTESIAN_POINT ( 'NONE',  ( -11.68405858231679595, -21.32873467460644079, 2.757051763020455404 ) ) ;
#1016=CARTESIAN_POINT ( 'NONE',  ( -10.84719141768317741, -20.91377862118959285, 1.020995438708345082 ) ) ;
#1018=CARTESIAN_POINT ( 'NONE',  ( 12.65396917024039958, -18.03705690286155772, 4.783553440007634272 ) ) ;
#1019=CARTESIAN_POINT ( 'NONE',  ( -13.12529418130016445, 5.014856155665242454, 4.958178834604180629 ) ) ;
#1026=CARTESIAN_POINT ( 'NONE',  ( 2.203959450683124377, -9.262433282444222371, 2.410528873095051594 ) ) ;
#1034=CARTESIAN_POINT ( 'NONE',  ( -1.711347482507859397, -9.865394108634699677, 1.622766275858107621 ) ) ;
#1038=CARTESIAN_POINT ( 'NONE',  ( 11.40969141768317918, -21.01515356694492098, 6.020995438708349745 ) ) ;
#1039=CARTESIAN_POINT ( 'NONE',  ( -13.06655316810189227, 2.048434989138931961, 5.965524842914772030 ) ) ;
#1041=CARTESIAN_POINT ( 'NONE',  ( -3.974842109207560537, -21.73478823434188456, 6.006404853634143670 ) ) ;
#1045=CARTESIAN_POINT ( 'NONE',  ( 10.37155858231679417, -20.24999999999999289, 3.449312527122348371 ) ) ;
#1047=CARTESIAN_POINT ( 'NONE',  ( -13.48548920624593883, -15.42029508461213716, 6.325359435864005064 ) ) ;
#1049=EDGE_CURVE ( 'NONE', #9910, #11689, #11331, .T. ) ;
#1050=CARTESIAN_POINT ( 'NONE',  ( 11.40280858231679417, -22.77556120703056308, 1.770995438708339975 ) ) ;
#1054=CARTESIAN_POINT ( 'NONE',  ( 13.60059015675642513, -9.607697083824668027, 6.450359435862663027 ) ) ;
#1055=CARTESIAN_POINT ( 'NONE',  ( -2.786182376113650605, -10.12667130264514626, 1.882483419865550900 ) ) ;
#1059=EDGE_CURVE ( 'NONE', #17561, #14618, #6947, .T. ) ;
#1066=CARTESIAN_POINT ( 'NONE',  ( 2.589709240944451096, -9.559844081062008669, 1.736909907557668165 ) ) ;
#1068=CARTESIAN_POINT ( 'NONE',  ( -13.09001666039658573, 3.983341349998239966, 5.257104358157307367 ) ) ;
#1069=CARTESIAN_POINT ( 'NONE',  ( 10.27780858231679417, -20.27099543870833642, 2.724438792969431589 ) ) ;
#1070=CARTESIAN_POINT ( 'NONE',  ( -13.37499999999998224, -20.99999999999991829, 4.333333333333343695 ) ) ;
#1072=CARTESIAN_POINT ( 'NONE',  ( 10.18405858231679417, -20.79840458871652942, 2.226721677130544030 ) ) ;
#1075=CARTESIAN_POINT ( 'NONE',  ( 11.12844141768317741, -20.99999999999999645, 3.550687472877664952 ) ) ;
#1076=CARTESIAN_POINT ( 'NONE',  ( -12.05905858231679417, -20.72672167713054137, 4.701595411283463477 ) ) ;
#1077=EDGE_LOOP ( 'NONE', ( #18859, #14241, #20611, #6809, #18260 ) ) ;
#1078=CARTESIAN_POINT ( 'NONE',  ( 13.47561960997282071, -14.41870969638424071, 4.846833296715798767 ) ) ;
#1084=CARTESIAN_POINT ( 'NONE',  ( -12.62499979224180180, -20.25001049178813162, 4.458178821399696012 ) ) ;
#1086=CARTESIAN_POINT ( 'NONE',  ( -13.87367531042247748, 4.933103176334663331, 5.324010972534209074 ) ) ;
#1090=CARTESIAN_POINT ( 'NONE',  ( -12.62500000000001954, -20.25000000000274269, 4.083333333315724012 ) ) ;
#1093=CARTESIAN_POINT ( 'NONE',  ( -1.513434189748285696, -9.114917468222230923, 2.372643865078341019 ) ) ;
#1094=CARTESIAN_POINT ( 'NONE',  ( -11.77780858231679595, -19.52099543870833642, 2.413778621189609286 ) ) ;
#1095=CARTESIAN_POINT ( 'NONE',  ( -2.844469389063872811, -10.54053385813977606, 1.988770633557972012 ) ) ;
#1097=CARTESIAN_POINT ( 'NONE',  ( -13.37500000000002132, -20.25000000000274269, 4.083333333315724012 ) ) ;
#1100=CARTESIAN_POINT ( 'NONE',  ( 5.590308582316795949, -21.01515356694490322, 0.9790045612916562501 ) ) ;
#1101=CARTESIAN_POINT ( 'NONE',  ( -7.659691417683177406, -22.36352608949543352, 2.479004561291652031 ) ) ;
#1104=CARTESIAN_POINT ( 'NONE',  ( 13.54769662923970763, -11.52882022337116119, 5.659013032956382361 ) ) ;
#1112=CARTESIAN_POINT ( 'NONE',  ( -13.75871503850933841, -0.8723905552644914962, 5.888179699623941943 ) ) ;
#1119=CARTESIAN_POINT ( 'NONE',  ( 2.830107938415192148, -10.43856789473369950, 1.962583737180462418 ) ) ;
#1126=CARTESIAN_POINT ( 'NONE',  ( 8.128441417683177406, -20.99999999999999645, 3.550687472877664952 ) ) ;
#1127=CARTESIAN_POINT ( 'NONE',  ( -13.09532840572934376, 3.501584489333809724, 5.996774842915142401 ) ) ;
#1128=CARTESIAN_POINT ( 'NONE',  ( -8.871558582316795949, -20.99999999999999645, 3.449312527122348371 ) ) ;
#1129=CARTESIAN_POINT ( 'NONE',  ( -7.753441417683177406, -21.94931252712233061, 0.9999999999999978906 ) ) ;
#1131=CARTESIAN_POINT ( 'NONE',  ( 12.62506359033936754, -19.49678868786235597, 4.541393094775662220 ) ) ;
#1132=CARTESIAN_POINT ( 'NONE',  ( -12.83635126708105823, -9.576761012430582198, 5.715524842913705328 ) ) ;
#1136=CARTESIAN_POINT ( 'NONE',  ( 1.824218240560544047, -9.921717538097572842, 2.387231257717697286 ) ) ;
#1141=CARTESIAN_POINT ( 'NONE',  ( -2.049450250860079592, -10.15122911285664564, 1.696174415070213382 ) ) ;
#1146=CARTESIAN_POINT ( 'NONE',  ( 10.75344141768317741, -21.94931252712233061, 0.9999999999999978906 ) ) ;
#1147=CARTESIAN_POINT ( 'NONE',  ( -13.12119116326504908, 4.807653744879115010, 5.626470997801169105 ) ) ;
#1148=CARTESIAN_POINT ( 'NONE',  ( -10.65969141768318096, -22.67418626127524917, 1.729004561291651809 ) ) ;
#1150=CARTESIAN_POINT ( 'NONE',  ( 11.02780858231679595, -23.72900456129165647, 4.275561207030568411 ) ) ;
#1152=CARTESIAN_POINT ( 'NONE',  ( -13.87144757537903494, 4.070602556641903291, 6.741633940066556363 ) ) ;
#1153=CARTESIAN_POINT ( 'NONE',  ( 11.02780858231679595, -23.72900456129165647, 4.275561207030568411 ) ) ;
#1157=CARTESIAN_POINT ( 'NONE',  ( 13.44712222274167246, -17.35782775154002522, 6.283692769197384287 ) ) ;
#1163=CARTESIAN_POINT ( 'NONE',  ( 13.87470602645761986, 4.985154336109792972, 4.916666666666650087 ) ) ;
#1165=CARTESIAN_POINT ( 'NONE',  ( 2.532303758294933704, -8.551221675625164664, 1.670490507339845054 ) ) ;
#1168=CARTESIAN_POINT ( 'NONE',  ( -13.37499999999998224, -19.50000000000006040, 4.416666666666682062 ) ) ;
#1170=CARTESIAN_POINT ( 'NONE',  ( -13.37543017851028893, -20.97827598523083026, 4.780017688621249761 ) ) ;
#1173=CARTESIAN_POINT ( 'NONE',  ( 11.96530858231679595, -20.22900456129164937, 4.174186261275266929 ) ) ;
#1175=CARTESIAN_POINT ( 'NONE',  ( 11.31594141768317741, -21.32873467460645145, 4.242948236979555254 ) ) ;
#1176=CARTESIAN_POINT ( 'NONE',  ( -7.090308582316794173, -21.32581373872472597, 1.729004561291657582 ) ) ;
#1178=CARTESIAN_POINT ( 'NONE',  ( 13.38090111944825367, -19.20199346786276351, 4.743968713382380464 ) ) ;
#1183=CARTESIAN_POINT ( 'NONE',  ( -12.64931222250080545, -19.02223276370786209, 5.512399842915133519 ) ) ;
#1186=CARTESIAN_POINT ( 'NONE',  ( -13.86106797245302147, 4.296432608878145487, 5.947261916831099171 ) ) ;
#1187=EDGE_CURVE ( 'NONE', #11689, #18614, #8308, .T. ) ;
#1189=CARTESIAN_POINT ( 'NONE',  ( 2.693754455098655409, -10.14181605509423711, 1.874202551270839123 ) ) ;
#1193=CARTESIAN_POINT ( 'NONE',  ( -8.027808582316795949, -24.47900456129166358, 4.586221378810390270 ) ) ;
#1194=CARTESIAN_POINT ( 'NONE',  ( -0.2815691515810352930, -9.114917468222230923, 1.622643865078524206 ) ) ;
#1198=CARTESIAN_POINT ( 'NONE',  ( -13.84495141469777479, 4.232546442235974204, 5.040078719623224401 ) ) ;
#1201=CARTESIAN_POINT ( 'NONE',  ( 5.965308582316795949, -19.47900456129164937, 4.484846433055089676 ) ) ;
#1202=CARTESIAN_POINT ( 'NONE',  ( -4.659691417683177406, -22.36352608949543352, 2.479004561291652031 ) ) ;
#1204=CARTESIAN_POINT ( 'NONE',  ( 13.87470602645415063, 4.985154336109792972, 3.333333333332063830 ) ) ;
#1211=CARTESIAN_POINT ( 'NONE',  ( -13.85343352903393388, 3.910893216212274925, 5.991044282956552891 ) ) ;
#1216=EDGE_CURVE ( 'NONE', #11536, #7438, #16444, .T. ) ;
#1218=CARTESIAN_POINT ( 'NONE',  ( 3.342893013439646843, -9.383962644129466568, 1.884355023724047173 ) ) ;
#1224=CARTESIAN_POINT ( 'NONE',  ( 7.378441417683177406, -22.99999999999999645, 3.449312527122335048 ) ) ;
#1225=CARTESIAN_POINT ( 'NONE',  ( -13.12512971825177033, 5.006550771716304915, 5.133277049491872468 ) ) ;
#1226=CARTESIAN_POINT ( 'NONE',  ( -9.246558582316795949, -21.94931252712234127, 4.499999999999999112 ) ) ;
#1227=CARTESIAN_POINT ( 'NONE',  ( -10.37844141768317741, -24.50000000000000000, 3.449312527122335048 ) ) ;
#1229=CARTESIAN_POINT ( 'NONE',  ( 13.37499999999998224, -19.49999999999991473, 4.333333333333343695 ) ) ;
#1234=CARTESIAN_POINT ( 'NONE',  ( 1.904508877737772998, -9.138371295333994837, 2.378667276417936627 ) ) ;
#1241=CARTESIAN_POINT ( 'NONE',  ( -2.167793999318431197, -10.98794063836983703, 1.911058649813994315 ) ) ;
#1246=CARTESIAN_POINT ( 'NONE',  ( 5.690941417683177406, -23.80360840875937001, 5.231925497173365081 ) ) ;
#1248=CARTESIAN_POINT ( 'NONE',  ( -11.78469141768317563, -23.77099543870834353, 4.174186261275252718 ) ) ;
#1250=CARTESIAN_POINT ( 'NONE',  ( 9.527808582316792396, -23.72900456129165647, 4.275561207030568411 ) ) ;
#1252=CARTESIAN_POINT ( 'NONE',  ( -13.40787921250184311, -19.33959976865745389, 6.241060671539915283 ) ) ;
#1254=CARTESIAN_POINT ( 'NONE',  ( 5.965308582316795949, -20.97900456129165647, 3.863526089495444626 ) ) ;
#1258=CARTESIAN_POINT ( 'NONE',  ( 13.40653076352726103, -19.40769644187082932, 6.236886054669082746 ) ) ;
#1264=CARTESIAN_POINT ( 'NONE',  ( -9.996558582316794173, -22.05068747287764452, 1.749999999999998446 ) ) ;
#1265=CARTESIAN_POINT ( 'NONE',  ( 13.87470602645761808, 4.985154336109792972, 4.000000000000000000 ) ) ;
#1267=CARTESIAN_POINT ( 'NONE',  ( 1.619022621591187150, -9.114917468222230923, 1.622643865078341463 ) ) ;
#1269=CARTESIAN_POINT ( 'NONE',  ( -13.37514942709654164, -19.49245393162283690, 4.562067678168288509 ) ) ;
#1270=CARTESIAN_POINT ( 'NONE',  ( 7.184058582316794173, -20.79840458871652942, 2.226721677130544030 ) ) ;
#1271=CARTESIAN_POINT ( 'NONE',  ( -12.62499999999998224, -20.99999999999998934, 4.291666666666699825 ) ) ;
#1273=CARTESIAN_POINT ( 'NONE',  ( 5.496558582316795949, -22.05068747287764452, 2.499999999999999112 ) ) ;
#1274=CARTESIAN_POINT ( 'NONE',  ( 10.09719141768317741, -22.46490103525075810, 4.479004561291653808 ) ) ;
#1275=CARTESIAN_POINT ( 'NONE',  ( -12.06594141768317563, -23.20159541128344927, 2.226721677130534705 ) ) ;
#1277=CARTESIAN_POINT ( 'NONE',  ( 13.09556065010287362, 4.263312830196960057, 5.034075356110313315 ) ) ;
#1278=CARTESIAN_POINT ( 'NONE',  ( -2.781778019848414552, -10.09537774617444938, 1.874445651118397560 ) ) ;
#1285=CARTESIAN_POINT ( 'NONE',  ( -13.06655316810189227, 2.048434989138931961, 5.965524842914772030 ) ) ;
#1286=CARTESIAN_POINT ( 'NONE',  ( -1.513434189748285918, -8.364917468222230923, 2.372643865078341019 ) ) ;
#1287=CARTESIAN_POINT ( 'NONE',  ( -13.39107665282975645, -19.43812903209671461, 5.476542851584349947 ) ) ;
#1293=CARTESIAN_POINT ( 'NONE',  ( -13.37155858231679595, -19.49999999999998934, 3.449312527122348371 ) ) ;
#1294=CARTESIAN_POINT ( 'NONE',  ( -1.548630333695928618, -8.364917468222230923, 1.622643865078341907 ) ) ;
#1296=CARTESIAN_POINT ( 'NONE',  ( -13.39296152110871851, -19.34294318400601753, 5.489418334493660012 ) ) ;
#1298=CARTESIAN_POINT ( 'NONE',  ( 4.717959273841179524, -21.63341328858655999, 5.993595146365859883 ) ) ;
#1299=CARTESIAN_POINT ( 'NONE',  ( -12.62155858231679417, -22.99999999999999645, 3.550687472877652073 ) ) ;
#1301=CARTESIAN_POINT ( 'NONE',  ( 13.38172782443493602, -20.66024486603417643, 5.557997437521964734 ) ) ;
#1302=CARTESIAN_POINT ( 'NONE',  ( 12.62499999998404121, -20.24999999996810729, 2.793053905886972998 ) ) ;
#1311=CARTESIAN_POINT ( 'NONE',  ( -13.85723511636018301, 4.102873376188801657, 5.986996695041598926 ) ) ;
#1316=CARTESIAN_POINT ( 'NONE',  ( -3.944195004867014909, -21.61378581760806128, 5.207602947182413011 ) ) ;
#1319=VECTOR ( 'NONE', #14885, 1000.000000000000114 ) ;
#1320=CARTESIAN_POINT ( 'NONE',  ( 2.722060606927515725, -8.660968749821154944, 1.698675748411476283 ) ) ;
#1329=CARTESIAN_POINT ( 'NONE',  ( 6.253441417683175629, -21.94931252712233061, 2.499999999999999112 ) ) ;
#1330=CARTESIAN_POINT ( 'NONE',  ( -13.12463908936614132, 4.981774012991869505, 5.264611377988129171 ) ) ;
#1331=CARTESIAN_POINT ( 'NONE',  ( -11.87155858231679595, -20.99999999999999645, 3.449312527122348371 ) ) ;
#1332=CARTESIAN_POINT ( 'NONE',  ( -11.50344141768317563, -22.05068747287765873, 5.250000000000000888 ) ) ;
#1334=CARTESIAN_POINT ( 'NONE',  ( 13.09560260347216953, 4.265431475339161338, 5.020858537328734883 ) ) ;
#1340=CARTESIAN_POINT ( 'NONE',  ( 3.047379876266447685, -13.13734219723468755, 3.405682891496055742 ) ) ;
#1346=CARTESIAN_POINT ( 'NONE',  ( -1.872293763630120678, -10.04602735435188698, 2.419156501869924369 ) ) ;
#1350=CARTESIAN_POINT ( 'NONE',  ( 8.409691417683177406, -21.01515356694492098, 6.020995438708349745 ) ) ;
#1352=CARTESIAN_POINT ( 'NONE',  ( -8.784691417683177406, -23.77099543870834353, 4.174186261275252718 ) ) ;
#1354=CARTESIAN_POINT ( 'NONE',  ( 9.434058582316794173, -23.20159541128345992, 4.773278322869455970 ) ) ;
#1356=CARTESIAN_POINT ( 'NONE',  ( -12.62500028073152869, -20.99998582305707728, 4.544498183892649479 ) ) ;
#1359=CARTESIAN_POINT ( 'NONE',  ( 8.027808582316792396, -23.72900456129165647, 4.275561207030568411 ) ) ;
#1369=CARTESIAN_POINT ( 'NONE',  ( -9.152808582316794173, -21.22443879296942626, 5.229004561291659137 ) ) ;
#1370=CARTESIAN_POINT ( 'NONE',  ( 12.62562019941893432, -20.21867992933967173, 4.757612834768309540 ) ) ;
#1372=CARTESIAN_POINT ( 'NONE',  ( 2.121089610268797276, -8.411987239090384705, 1.634732322550447758 ) ) ;
#1377=CARTESIAN_POINT ( 'NONE',  ( -13.09080647246885576, 4.023226859705822278, 5.257958009367514229 ) ) ;
#1378=CARTESIAN_POINT ( 'NONE',  ( 9.152808582316794173, -21.22443879296942626, 5.229004561291659137 ) ) ;
#1379=CARTESIAN_POINT ( 'NONE',  ( -13.90411326029870409, 5.720219645086723759, 5.230514352905474063 ) ) ;
#1380=CARTESIAN_POINT ( 'NONE',  ( 3.944195004867014909, -21.61378581760806128, 5.207602947182413011 ) ) ;
#1381=CARTESIAN_POINT ( 'NONE',  ( 8.684058582316794173, -20.79840458871652942, 2.226721677130544030 ) ) ;
#1382=CARTESIAN_POINT ( 'NONE',  ( 12.80905858231679417, -22.74294823697954016, 2.828734674606448785 ) ) ;
#1383=CARTESIAN_POINT ( 'NONE',  ( -5.777808582316794173, -20.27099543870833642, 2.724438792969431589 ) ) ;
#1385=CARTESIAN_POINT ( 'NONE',  ( 13.45643611822145225, -15.38747602984844853, 4.825999963382285429 ) ) ;
#1386=CARTESIAN_POINT ( 'NONE',  ( -2.195822829018478473, -9.226849102155203042, 1.651390144731336163 ) ) ;
#1392=CARTESIAN_POINT ( 'NONE',  ( -0.2815691515810352930, -9.114917468222230923, 2.372643865078523984 ) ) ;
#1393=CARTESIAN_POINT ( 'NONE',  ( -13.38238173943565990, -19.87722215849730034, 5.285856107751903288 ) ) ;
#1397=CARTESIAN_POINT ( 'NONE',  ( 10.65280858231679240, -21.22443879296942626, 5.229004561291660025 ) ) ;
#1399=CARTESIAN_POINT ( 'NONE',  ( 13.10985494974158705, 3.485174961951963191, 6.746454579156001330 ) ) ;
#1401=CARTESIAN_POINT ( 'NONE',  ( -12.25344141768317741, -21.94931252712233061, 0.9999999999999978906 ) ) ;
#1402=CARTESIAN_POINT ( 'NONE',  ( -1.939860967060266672, -10.52577007527361808, 2.542364016426418516 ) ) ;
#1404=CARTESIAN_POINT ( 'NONE',  ( -13.84311479963346869, 4.139797381492562600, 5.195993353439945395 ) ) ;
#1406=CARTESIAN_POINT ( 'NONE',  ( 8.690941417683177406, -23.80360840875937001, 5.231925497173365081 ) ) ;
#1407=CARTESIAN_POINT ( 'NONE',  ( -6.065941417683177406, -22.67126532539353789, 2.757051763020445634 ) ) ;
#1410=CARTESIAN_POINT ( 'NONE',  ( 13.37526900345969771, -20.98641532528209908, 4.724331462949078464 ) ) ;
#1411=CARTESIAN_POINT ( 'NONE',  ( 12.62745083560477966, -20.12623280195927933, 5.001038150054709419 ) ) ;
#1415=CARTESIAN_POINT ( 'NONE',  ( -13.87066368810231154, 4.781016249162736820, 5.617237349937618696 ) ) ;
#1422=CARTESIAN_POINT ( 'NONE',  ( 3.502569552650398155, -9.961070227720959736, 2.032567780072621400 ) ) ;
#1428=CARTESIAN_POINT ( 'NONE',  ( -13.33466323279248122, -20.44601834413422026, 3.454345736197117045 ) ) ;
#1429=CARTESIAN_POINT ( 'NONE',  ( 7.565941417683177406, -22.67126532539353789, 2.757051763020445634 ) ) ;
#1430=CARTESIAN_POINT ( 'NONE',  ( -12.91308523408712183, -5.701695678577235249, 5.798858176249892082 ) ) ;
#1431=CARTESIAN_POINT ( 'NONE',  ( -7.559058582316795949, -21.25705176302045274, 4.171265325393551215 ) ) ;
#1433=CARTESIAN_POINT ( 'NONE',  ( -10.56594141768317741, -23.20159541128344927, 2.226721677130534705 ) ) ;
#1436=CARTESIAN_POINT ( 'NONE',  ( 13.37505992445764136, -19.49697381488866554, 4.539006848837218833 ) ) ;
#1439=EDGE_CURVE ( 'NONE', #13028, #8942, #18411, .T. ) ;
#1440=CARTESIAN_POINT ( 'NONE',  ( 12.62672070884157804, -20.24999999999983658, 3.550922209436377042 ) ) ;
#1442=CARTESIAN_POINT ( 'NONE',  ( 1.707060460004204527, -9.864918773552613374, 2.372644200313257290 ) ) ;
#1444=CARTESIAN_POINT ( 'NONE',  ( 9.722191417683177406, -20.27099543870833998, 4.275561207030583510 ) ) ;
#1447=CARTESIAN_POINT ( 'NONE',  ( -1.896776615114361908, -10.21987218505477024, 2.463803327293850209 ) ) ;
#1452=CARTESIAN_POINT ( 'NONE',  ( 5.315941417683176518, -20.26807450282663225, 5.303608408759377113 ) ) ;
#1453=CARTESIAN_POINT ( 'NONE',  ( -7.847191417683176518, -21.22443879296941915, 1.770995438708345748 ) ) ;
#1455=CARTESIAN_POINT ( 'NONE',  ( 8.871558582316794173, -20.24999999999999289, 3.449312527122348371 ) ) ;
#1457=CARTESIAN_POINT ( 'NONE',  ( -12.62500000000002132, -20.99999999999450395, 3.833333333368183382 ) ) ;
#1459=CARTESIAN_POINT ( 'NONE',  ( 6.340308582316793284, -22.67418626127525982, 5.270995438708342640 ) ) ;
#1464=ADVANCED_FACE ( 'NONE', ( #12881 ), #14233, .T. ) ;
#1467=CARTESIAN_POINT ( 'NONE',  ( -6.246558582316794173, -21.94931252712234482, 5.250000000000000888 ) ) ;
#1470=CARTESIAN_POINT ( 'NONE',  ( 1.407845757905374695, -9.864917468222230923, 1.622643865078341907 ) ) ;
#1474=CARTESIAN_POINT ( 'NONE',  ( -13.74418849449709512, -0.8559810278826442964, 5.138499963383082125 ) ) ;
#1476=CARTESIAN_POINT ( 'NONE',  ( 4.717959273841178636, -21.72818306014730183, 5.243595146365860771 ) ) ;
#1477=CARTESIAN_POINT ( 'NONE',  ( -13.90434039801927568, 5.731690099970989216, 5.115558489342345361 ) ) ;
#1478=CARTESIAN_POINT ( 'NONE',  ( 7.746558582316794173, -21.94931252712234482, 5.250000000000000888 ) ) ;
#1479=CARTESIAN_POINT ( 'NONE',  ( 5.503441417683177406, -22.05068747287766229, 4.499999999999999112 ) ) ;
#1480=CARTESIAN_POINT ( 'NONE',  ( -12.34719141768317741, -21.22443879296941915, 1.770995438708345748 ) ) ;
#1481=B_SPLINE_CURVE_WITH_KNOTS ( 'NONE', 3,
 ( #3169, #1591, #1494, #12672, #18967, #4623, #11016, #14344, #7874, #4731, #28, #6415, #12780, #17808, #14766, #6919, #5352, #10263, #5459, #540, #8399, #19494, #9951, #16336, #19804, #2010, #11831, #5243, #10065, #11523 ),
 .UNSPECIFIED., .F., .F.,
 ( 4, 2, 2, 2, 2, 2, 2, 2, 2, 2, 2, 2, 2, 2, 4 ),
 ( 0.6080100341812841869, 0.6200887121040892236, 0.6309950902025724950, 0.6419014683010558775, 0.6637142244980225314, 0.7073397368919559502, 0.7509652492858893691, 0.7727780054828560230, 0.7836843835813394055, 0.7945907616798226769, 0.8074288390748337596, 0.8202669164698448423, 0.8459430712598670077, 0.8972953808399113385, 1.000000000000000000 ),
 .UNSPECIFIED. ) ;
#1483=CARTESIAN_POINT ( 'NONE',  ( 13.38569699238614952, -18.95980188449660986, 4.749177046715717054 ) ) ;
#1484=CARTESIAN_POINT ( 'NONE',  ( -1.126276606324276619, -9.114917468222230923, 1.622643865078341463 ) ) ;
#1490=CARTESIAN_POINT ( 'NONE',  ( -4.066879903460562495, -13.96783368734915776, 3.061584679647603391 ) ) ;
#1494=CARTESIAN_POINT ( 'NONE',  ( 2.777355782919915139, -10.06396397089670458, 1.866377966073868411 ) ) ;
#1497=CARTESIAN_POINT ( 'NONE',  ( 12.62500016093973620, -20.24999187254239175, 4.532396751752561848 ) ) ;
#1498=CARTESIAN_POINT ( 'NONE',  ( -11.40969141768317918, -21.01515356694492098, 6.020995438708349745 ) ) ;
#1499=CARTESIAN_POINT ( 'NONE',  ( -1.707060460004204527, -9.864918773552613374, 2.372644200313257290 ) ) ;
#1501=CARTESIAN_POINT ( 'NONE',  ( -13.82092246150448211, 3.019084305971233562, 5.221833296715730377 ) ) ;
#1503=CARTESIAN_POINT ( 'NONE',  ( 4.847191417683177406, -20.91377862118959285, 1.020995438708345082 ) ) ;
#1504=CARTESIAN_POINT ( 'NONE',  ( -10.93405858231679595, -22.67126532539354855, 4.242948236979545484 ) ) ;
#1506=CARTESIAN_POINT ( 'NONE',  ( 13.87470602645761986, 4.985154336109792972, 4.583333333333296622 ) ) ;
#1507=CARTESIAN_POINT ( 'NONE',  ( 12.64131715375063258, -19.42598373559290792, 5.491151580003103660 ) ) ;
#1519=CARTESIAN_POINT ( 'NONE',  ( 0.2815691515810352374, -8.364917468222230923, 1.622643865078524428 ) ) ;
#1522=CARTESIAN_POINT ( 'NONE',  ( 2.693754455098655409, -10.04853567022903782, 2.237415670251142519 ) ) ;
#1524=CARTESIAN_POINT ( 'NONE',  ( -13.09030858231679417, -21.32581373872472597, 1.729004561291657582 ) ) ;
#1525=CARTESIAN_POINT ( 'NONE',  ( -2.367358971471363649, -9.400572650371021410, 2.446005822389718087 ) ) ;
#1527=CARTESIAN_POINT ( 'NONE',  ( 8.972191417683177406, -22.97900456129165292, 3.035098964749240125 ) ) ;
#1528=CARTESIAN_POINT ( 'NONE',  ( -13.12529397354238192, 5.014845663890295846, 4.333333333333382775 ) ) ;
#1529=CARTESIAN_POINT ( 'NONE',  ( -12.71530858231679240, -23.77099543870833998, 2.825813738724734847 ) ) ;
#1530=CARTESIAN_POINT ( 'NONE',  ( -5.503441417683177406, -22.05068747287766229, 6.000000000000001776 ) ) ;
#1532=CARTESIAN_POINT ( 'NONE',  ( 12.89855869007488209, -5.685286151195387383, 5.049178440009032265 ) ) ;
#1543=CARTESIAN_POINT ( 'NONE',  ( 0.000000000000000000, -9.864917468222230923, 2.372643865078341019 ) ) ;
#1545=CARTESIAN_POINT ( 'NONE',  ( -10.09030858231679417, -21.32581373872472952, 1.729004561291657138 ) ) ;
#1546=CARTESIAN_POINT ( 'NONE',  ( 7.565941417683177406, -23.73192549717336064, 1.696391591240623331 ) ) ;
#1548=CARTESIAN_POINT ( 'NONE',  ( -11.31594141768317741, -20.79840458871654363, 4.773278322869464851 ) ) ;
#1550=CARTESIAN_POINT ( 'NONE',  ( 5.402808582316794173, -22.77556120703056308, 1.770995438708339975 ) ) ;
#1552=CARTESIAN_POINT ( 'NONE',  ( -13.04271272860988340, 0.09449279482665236263, 6.673537912489449830 ) ) ;
#1555=CARTESIAN_POINT ( 'NONE',  ( 8.496558582316794173, -22.05068747287764452, 1.749999999999998446 ) ) ;
#1556=CARTESIAN_POINT ( 'NONE',  ( 13.12500000000000000, 5.004982103124741677, 3.999999999999983569 ) ) ;
#1561=B_SPLINE_CURVE_WITH_KNOTS ( 'NONE', 3,
 ( #16574, #2154, #15119, #689, #16679, #8536, #8748, #2251, #13441, #7179, #13640, #19945, #14907, #8850, #5602, #8638, #15009, #11974, #19845, #18264, #5497, #4033, #15218, #10419, #13232, #16378, #10310, #8443, #19630, #9357, #9254, #18475, #15525, #4453, #14058, #5813, #4549, #2877, #15624, #16991, #5712, #6125, #16889, #12391, #7488, #1112, #13850, #20049, #2669, #12083, #4136, #10728, #15734, #20153, #998, #10518, #7388, #1211, #10837, #17201, #7690, #1311, #9056, #10932, #20466, #2559, #8945, #1415, #7797, #15318, #9157, #12494, #13751, #5911, #7586, #12183, #18573, #4236, #10617, #15427, #2780, #20252, #18888, #12282 ),
 .UNSPECIFIED., .F., .F.,
 ( 4, 2, 2, 2, 2, 2, 2, 2, 2, 2, 2, 2, 2, 2, 2, 2, 2, 2, 2, 2, 2, 2, 2, 2, 2, 2, 2, 2, 2, 2, 2, 2, 2, 2, 2, 2, 2, 2, 2, 2, 2, 4 ),
 ( 0.03313147696908362583, 0.03481082764294501225, 0.05122453910963482154, 0.05943139484297972619, 0.06353482270965217504, 0.06763825057632462390, 0.07081696859385247511, 0.07399568661138032633, 0.08035312264643602875, 0.09306799471654744749, 0.1057828667866588385, 0.1121403028217145548, 0.1153190208392423921, 0.1184977388567702433, 0.1214804596100246686, 0.1244631803632790662, 0.1304286218697878474, 0.1423595048828054654, 0.1662212709088405904, 0.2139448029609110069, 0.3093918670650517844, 0.5002859952733332838, 0.6911801234816148387, 0.7866271875857555607, 0.8343507196378260327, 0.8582124856638612131, 0.8701433686768788034, 0.8761088101833875985, 0.8790915309366421626, 0.8820742516898965047, 0.8853411830926055659, 0.8886081144953145161, 0.8951419773007326386, 0.9082097029115688835, 0.9212774285224051285, 0.9278112913278232510, 0.9310782227305320902, 0.9343451541332412624, 0.9384485819999136558, 0.9425520098665861601, 0.9507588655999309468, 0.9671725770666207422 ),
 .UNSPECIFIED. ) ;
#1564=CARTESIAN_POINT ( 'NONE',  ( -13.09030858231679417, -21.01515356694490322, 0.9790045612916562501 ) ) ;
#1568=CARTESIAN_POINT ( 'NONE',  ( 2.110348196723525138, -10.58007678474401914, 1.806311064303893099 ) ) ;
#1572=CARTESIAN_POINT ( 'NONE',  ( -13.84500676459759383, 4.235341612176667603, 5.016097456370799179 ) ) ;
#1573=CARTESIAN_POINT ( 'NONE',  ( 7.934058582316792396, -23.20159541128345992, 4.773278322869455970 ) ) ;
#1574=CARTESIAN_POINT ( 'NONE',  ( -12.62499999999998224, -20.99999999999991829, 4.333333333333343695 ) ) ;
#1576=CARTESIAN_POINT ( 'NONE',  ( -6.996558582316795949, -22.05068747287764452, 0.9999999999999978906 ) ) ;
#1577=CARTESIAN_POINT ( 'NONE',  ( 9.152808582316794173, -21.22443879296942626, 5.229004561291659137 ) ) ;
#1578=CARTESIAN_POINT ( 'NONE',  ( 6.815941417683177406, -21.32873467460645145, 4.242948236979555254 ) ) ;
#1579=CARTESIAN_POINT ( 'NONE',  ( -6.434058582316794173, -23.20159541128345992, 4.773278322869455970 ) ) ;
#1581=CARTESIAN_POINT ( 'NONE',  ( 13.84074239313819277, 4.019990853478630832, 5.241358430878110930 ) ) ;
#1588=CARTESIAN_POINT ( 'NONE',  ( -13.11017182064853159, 4.251176942750957366, 5.979809059808775196 ) ) ;
#1589=CARTESIAN_POINT ( 'NONE',  ( -3.528325504133930313, -10.14411005961392398, 2.079576065490765124 ) ) ;
#1591=CARTESIAN_POINT ( 'NONE',  ( 2.781778019848414552, -10.09537774617444938, 1.874445651118397560 ) ) ;
#1592=CARTESIAN_POINT ( 'NONE',  ( -12.64691428603184242, -19.14332855539073464, 5.509795676248469221 ) ) ;
#1593=CARTESIAN_POINT ( 'NONE',  ( 10.46530858231679417, -20.22900456129164937, 4.174186261275266929 ) ) ;
#1595=CARTESIAN_POINT ( 'NONE',  ( 13.08107971211413378, 2.032025461757085427, 6.715204579155630960 ) ) ;
#1597=CARTESIAN_POINT ( 'NONE',  ( -1.407845757905374695, -9.864917468222230923, 1.622643865078341907 ) ) ;
#1599=CARTESIAN_POINT ( 'NONE',  ( -13.40022353639839103, -18.97621141187856608, 5.498856782956575984 ) ) ;
#1602=CARTESIAN_POINT ( 'NONE',  ( 7.940941417683175629, -20.19639159124061933, 1.768074502826635586 ) ) ;
#1603=CARTESIAN_POINT ( 'NONE',  ( -4.565941417683176518, -22.67126532539353789, 2.757051763020445634 ) ) ;
#1605=CARTESIAN_POINT ( 'NONE',  ( 13.87144757537903494, 4.070602556641903291, 6.741633940066556363 ) ) ;
#1606=CARTESIAN_POINT ( 'NONE',  ( 12.64323021897839006, -19.32937394158751943, 5.504219675487169283 ) ) ;
#1611=EDGE_CURVE ( 'NONE', #1939, #8942, #1481, .T. ) ;
#1617=CARTESIAN_POINT ( 'NONE',  ( 2.513306525444908512, -9.622685169956881168, 2.503048754562789746 ) ) ;
#1619=CARTESIAN_POINT ( 'NONE',  ( 0.000000000000000000, -9.864917468222230923, 1.622643865078341241 ) ) ;
#1625=CARTESIAN_POINT ( 'NONE',  ( -11.59030858231679417, -21.32581373872472597, 1.729004561291657582 ) ) ;
#1626=CARTESIAN_POINT ( 'NONE',  ( -2.875042468481914248, -11.91375063635796039, 3.091440134965714126 ) ) ;
#1628=CARTESIAN_POINT ( 'NONE',  ( 10.37155858231679595, -20.99999999999999645, 3.449312527122348371 ) ) ;
#1629=CARTESIAN_POINT ( 'NONE',  ( -12.63238774201960268, -19.12691902800888499, 4.760115940007608515 ) ) ;
#1630=CARTESIAN_POINT ( 'NONE',  ( -7.090308582316795061, -21.63647391050454871, 2.479004561291657804 ) ) ;
#1631=CARTESIAN_POINT ( 'NONE',  ( -5.128441417683177406, -19.49999999999998934, 3.550687472877664952 ) ) ;
#1634=CARTESIAN_POINT ( 'NONE',  ( 13.09560264575884503, 4.265433610975056133, 3.333333333333364568 ) ) ;
#1640=CARTESIAN_POINT ( 'NONE',  ( 13.41175265982446696, -19.14399067886409256, 6.245281310864100988 ) ) ;
#1643=B_SPLINE_CURVE_WITH_KNOTS ( 'NONE', 3,
 ( #10027, #11390, #5213, #8561, #19460, #1975, #11797, #5010, #14929, #11691, #8360, #18088, #410, #3850, #6996, #18186, #10230, #303, #16596, #609, #17974, #6793, #16406, #17776, #2081, #2274, #3443, #9822, #8466, #16207, #6690, #1873 ),
 .UNSPECIFIED., .F., .F.,
 ( 4, 2, 2, 2, 1, 2, 2, 2, 2, 2, 2, 2, 1, 2, 2, 2, 4 ),
 ( 0.5000677049534336671, 0.5625592418342705292, 0.5938050102746865733, 0.6094278944948945398, 0.6172393366049978569, 0.6211450576600495710, 0.6250507787151011740, 0.6875423155959299315, 0.7500338524767586890, 0.8125253893575872244, 0.8437711577980016031, 0.8593940420182086815, 0.8672054841283111104, 0.8711112051833602710, 0.8750169262384093205, 0.9375084631192046603, 1.000000000000000000 ),
 .UNSPECIFIED. ) ;
#1644=AXIS2_PLACEMENT_3D ( 'NONE', #12595, #17830, #249 ) ;
#1646=CARTESIAN_POINT ( 'NONE',  ( 10.94094141768317741, -20.72672167713052715, 2.298404588716546293 ) ) ;
#1648=AXIS2_PLACEMENT_3D ( 'NONE', #20610, #9197, #5956 ) ;
#1649=CARTESIAN_POINT ( 'NONE',  ( -2.875042468481914248, -11.91375063635796039, 3.091440134965714126 ) ) ;
#1651=CARTESIAN_POINT ( 'NONE',  ( -11.21530858231679417, -23.77099543870833998, 2.825813738724734847 ) ) ;
#1653=CARTESIAN_POINT ( 'NONE',  ( 6.159691417683175629, -22.98484643305507191, 0.9790045612916508100 ) ) ;
#1655=CARTESIAN_POINT ( 'NONE',  ( -4.190941417683176518, -23.27327832286946219, 4.701595411283453707 ) ) ;
#1657=CARTESIAN_POINT ( 'NONE',  ( 7.184058582316794173, -20.79840458871652942, 2.226721677130544030 ) ) ;
#1659=CARTESIAN_POINT ( 'NONE',  ( -13.07148796623841847, 1.547642295024179493, 6.704787912489258872 ) ) ;
#1661=CARTESIAN_POINT ( 'NONE',  ( 6.621558582316794173, -23.74999999999999645, 3.550687472877651629 ) ) ;
#1665=PRODUCT ( 'spring', 'spring', '', ( #14521 ) ) ;
#1668=ORIENTED_EDGE ( 'NONE', *, *, #11266, .F. ) ;
#1671=CARTESIAN_POINT ( 'NONE',  ( -12.62155858231679417, -24.50000000000000000, 3.550687472877651629 ) ) ;
#1674=CARTESIAN_POINT ( 'NONE',  ( 2.327620134574780231, -13.27885108724501251, 3.249410218619480872 ) ) ;
#1677=CARTESIAN_POINT ( 'NONE',  ( -13.37499999998404121, -20.24999999996810729, 2.793053905886972998 ) ) ;
#1678=CARTESIAN_POINT ( 'NONE',  ( 8.402808582316794173, -22.77556120703056308, 1.770995438708339975 ) ) ;
#1679=CARTESIAN_POINT ( 'NONE',  ( -12.69740987707854707, -17.34330120752609616, 6.298537912489285517 ) ) ;
#1680=STYLED_ITEM ( 'NONE', ( #6457 ), #11472 ) ;
#1683=CARTESIAN_POINT ( 'NONE',  ( 4.068047865639286442, -21.69070144236915354, 4.840187030888444042 ) ) ;
#1684=CARTESIAN_POINT ( 'NONE',  ( -10.37155858231679595, -19.49999999999998934, 3.449312527122348371 ) ) ;
#1685=CARTESIAN_POINT ( 'NONE',  ( 6.715308582316794173, -23.77099543870833998, 2.825813738724734847 ) ) ;
#1686=CARTESIAN_POINT ( 'NONE',  ( 5.409691417683178294, -21.63647391050456648, 4.520995438708348857 ) ) ;
#1687=CARTESIAN_POINT ( 'NONE',  ( -6.815941417683176518, -20.79840458871654363, 4.773278322869464851 ) ) ;
#1691=CARTESIAN_POINT ( 'NONE',  ( 13.37499999999998224, -20.24999999999991829, 4.333333333333343695 ) ) ;
#1702=CARTESIAN_POINT ( 'NONE',  ( -1.743623630681728542, -9.116095536440919744, 2.372946416531167557 ) ) ;
#1705=CARTESIAN_POINT ( 'NONE',  ( -12.62515553039088090, -20.24214571525854467, 4.629702272822510345 ) ) ;
#1708=CARTESIAN_POINT ( 'NONE',  ( 12.62499999999998579, -20.24999999999999289, 3.146526952850934755 ) ) ;
#1710=CARTESIAN_POINT ( 'NONE',  ( -1.772926875221950249, -9.883376166076789815, 2.377384427436886494 ) ) ;
#1712=CARTESIAN_POINT ( 'NONE',  ( -13.85788212999909419, 4.135547564954428879, 5.982801014393342776 ) ) ;
#1715=CARTESIAN_POINT ( 'NONE',  ( 5.315941417683176518, -20.26807450282663225, 5.303608408759377113 ) ) ;
#1716=CARTESIAN_POINT ( 'NONE',  ( -10.46530858231679595, -20.97900456129165647, 3.863526089495444626 ) ) ;
#1719=CARTESIAN_POINT ( 'NONE',  ( 13.86316420010827777, 3.652292105464413297, 6.735515685864076119 ) ) ;
#1720=CARTESIAN_POINT ( 'NONE',  ( 12.79798428357658047, -11.51429367935891790, 5.673858176248284479 ) ) ;
#1729=CARTESIAN_POINT ( 'NONE',  ( 2.011668220304084542, -11.03559989230542193, 2.673298498313999794 ) ) ;
#1735=CARTESIAN_POINT ( 'NONE',  ( -2.693754455098655409, -9.955255285363838524, 2.600628789231445470 ) ) ;
#1737=CARTESIAN_POINT ( 'NONE',  ( -2.817596665886821672, -11.50588678273290988, 2.986692549455723267 ) ) ;
#1738=CARTESIAN_POINT ( 'NONE',  ( 9.527808582316795949, -22.97900456129165647, 3.964901035250747885 ) ) ;
#1739=CARTESIAN_POINT ( 'NONE',  ( -13.09173631808601002, 4.070184063342107805, 5.250510817581989009 ) ) ;
#1740=CARTESIAN_POINT ( 'NONE',  ( -12.90280858231679773, -22.77556120703056308, 1.770995438708339975 ) ) ;
#1741=CARTESIAN_POINT ( 'NONE',  ( -10.28469141768318096, -23.77099543870834353, 4.174186261275252718 ) ) ;
#1743=CARTESIAN_POINT ( 'NONE',  ( 13.84439157666246878, 4.204274621457510186, 5.123803251657143676 ) ) ;
#1753=CARTESIAN_POINT ( 'NONE',  ( 8.690941417683177406, -23.27327832286946219, 4.701595411283453707 ) ) ;
#1755=CARTESIAN_POINT ( 'NONE',  ( -1.407845757905374695, -9.864917468222230923, 2.372643865078341019 ) ) ;
#1757=CARTESIAN_POINT ( 'NONE',  ( -12.62155858231679417, -23.74999999999999645, 3.550687472877651629 ) ) ;
#1759=CARTESIAN_POINT ( 'NONE',  ( 6.347191417683176518, -21.22443879296941915, 1.770995438708345748 ) ) ;
#1761=CARTESIAN_POINT ( 'NONE',  ( -11.40969141768317918, -21.63647391050456648, 4.520995438708348857 ) ) ;
#1763=CARTESIAN_POINT ( 'NONE',  ( 11.12155858231679595, -24.50000000000000000, 3.550687472877651629 ) ) ;
#1764=CARTESIAN_POINT ( 'NONE',  ( 12.62524871736568954, -20.23743977303344010, 4.661898514667671023 ) ) ;
#1765=CARTESIAN_POINT ( 'NONE',  ( -13.14782865898149034, 5.402847278557675104, 6.092770214907355708 ) ) ;
#1775=CARTESIAN_POINT ( 'NONE',  ( -5.402808582316794173, -22.77556120703056308, 1.770995438708339975 ) ) ;
#1778=CARTESIAN_POINT ( 'NONE',  ( 2.124709647372160060, -10.68204274815009924, 1.832497960681391147 ) ) ;
#1779=CARTESIAN_POINT ( 'NONE',  ( 12.62500000000001954, -20.24999999999450040, 3.833333333368183382 ) ) ;
#1781=CARTESIAN_POINT ( 'NONE',  ( -13.84501474873290938, 4.235744811019327649, 4.974109985360144037 ) ) ;
#1782=CARTESIAN_POINT ( 'NONE',  ( 9.434058582316795949, -23.73192549717337130, 5.303608408759367343 ) ) ;
#1783=CARTESIAN_POINT ( 'NONE',  ( -13.15469878640066526, 5.749788713235649773, 5.232478742873432509 ) ) ;
#1786=CARTESIAN_POINT ( 'NONE',  ( 6.902808582316793284, -22.77556120703056308, 1.770995438708339975 ) ) ;
#1787=CARTESIAN_POINT ( 'NONE',  ( 8.972191417683177406, -22.97900456129165292, 3.035098964749240125 ) ) ;
#1788=CARTESIAN_POINT ( 'NONE',  ( -4.753441417683176518, -21.94931252712233061, 1.749999999999998446 ) ) ;
#1791=CARTESIAN_POINT ( 'NONE',  ( 13.37499979530394967, -20.25001033714808329, 4.458488164327452097 ) ) ;
#1793=CARTESIAN_POINT ( 'NONE',  ( 0.000000000000000000, 0.000000000000000000, 0.000000000000000000 ) ) ;
#1800=CARTESIAN_POINT ( 'NONE',  ( -0.5631383031621635116, -8.364917468222230923, 1.622643865078341907 ) ) ;
#1804=CARTESIAN_POINT ( 'NONE',  ( -12.64751377014909828, -19.11305460747000495, 5.510446717915143289 ) ) ;
#1808=CARTESIAN_POINT ( 'NONE',  ( 13.15498530132288479, 5.764257716805535559, 4.791666666666684726 ) ) ;
#1809=CARTESIAN_POINT ( 'NONE',  ( -2.041623931606483033, -10.12028065167953272, 1.688226231982305370 ) ) ;
#1811=CARTESIAN_POINT ( 'NONE',  ( -13.49014615398506045, -14.43511922376608680, 5.596513032956658584 ) ) ;
#1813=CARTESIAN_POINT ( 'NONE',  ( 7.659691417683177406, -22.98484643305507191, 0.9790045612916508100 ) ) ;
#1814=CARTESIAN_POINT ( 'NONE',  ( -5.684058582316795949, -21.32873467460644079, 2.757051763020455404 ) ) ;
#1816=CARTESIAN_POINT ( 'NONE',  ( 13.90439735423812273, 5.734566389025032684, 2.999999999999999556 ) ) ;
#1817=CARTESIAN_POINT ( 'NONE',  ( 13.10431844137356627, 3.955581289335645234, 6.006545679920360925 ) ) ;
#1827=CARTESIAN_POINT ( 'NONE',  ( 1.982945319006538032, -10.83166796549307520, 2.620924705558935308 ) ) ;
#1833=CARTESIAN_POINT ( 'NONE',  ( -10.93405858231679417, -23.20159541128345992, 4.773278322869455970 ) ) ;
#1834=CARTESIAN_POINT ( 'NONE',  ( -12.62672070884157804, -20.24999999999991473, 3.550922209436377042 ) ) ;
#1837=CARTESIAN_POINT ( 'NONE',  ( -12.62599452815238443, -19.44977632830967806, 4.656396506304353977 ) ) ;
#1838=CARTESIAN_POINT ( 'NONE',  ( -11.96530858231679595, -20.22900456129164937, 4.174186261275266929 ) ) ;
#1839=CARTESIAN_POINT ( 'NONE',  ( -8.222191417683175629, -20.27099543870833998, 4.275561207030583510 ) ) ;
#1841=CARTESIAN_POINT ( 'NONE',  ( 13.79214722387705905, 1.565934805775630601, 5.190583296715636230 ) ) ;
#1847=VERTEX_POINT ( 'NONE', #852 ) ;
#1852=CARTESIAN_POINT ( 'NONE',  ( 11.59719141768317563, -22.77556120703057729, 5.229004561291656472 ) ) ;
#1854=CARTESIAN_POINT ( 'NONE',  ( -3.047379876266447685, -13.13734219723468755, 3.405682891496055742 ) ) ;
#1855=CARTESIAN_POINT ( 'NONE',  ( 2.436080212393455735, -9.483920418190111334, 2.467411194204634839 ) ) ;
#1856=CARTESIAN_POINT ( 'NONE',  ( -11.68405858231679417, -20.79840458871652942, 2.226721677130544030 ) ) ;
#1858=CARTESIAN_POINT ( 'NONE',  ( 8.222191417683175629, -20.27099543870833998, 4.275561207030583510 ) ) ;
#1861=CARTESIAN_POINT ( 'NONE',  ( -10.28469141768317741, -23.02099543870834353, 3.863526089495429972 ) ) ;
#1862=ORIENTED_EDGE ( 'NONE', *, *, #19649, .F. ) ;
#1863=CARTESIAN_POINT ( 'NONE',  ( 8.871558582316795949, -19.49999999999998934, 3.449312527122348371 ) ) ;
#1864=CARTESIAN_POINT ( 'NONE',  ( 12.62500000000001954, -20.24999999999450040, 3.833333333368183382 ) ) ;
#1865=CARTESIAN_POINT ( 'NONE',  ( -13.15498530132288479, 5.764257716805535559, 4.166666666666765551 ) ) ;
#1873=CARTESIAN_POINT ( 'NONE',  ( 12.62672070884157804, -20.24999999999983658, 3.550922209436377042 ) ) ;
#1876=CARTESIAN_POINT ( 'NONE',  ( -11.68405858231679595, -20.26807450282662160, 1.696391591240633101 ) ) ;
#1877=CARTESIAN_POINT ( 'NONE',  ( 13.09892531043291086, 3.683228176858501790, 6.000681092915118420 ) ) ;
#1881=CARTESIAN_POINT ( 'NONE',  ( 12.64571531779736979, -19.20387645123237164, 5.508493592915143289 ) ) ;
#1883=CARTESIAN_POINT ( 'NONE',  ( -13.40368151590352497, -18.05158344687463412, 4.768708296715732153 ) ) ;
#1884=CARTESIAN_POINT ( 'NONE',  ( 7.746558582316795949, -21.94931252712234127, 6.000000000000001776 ) ) ;
#1885=CARTESIAN_POINT ( 'NONE',  ( -13.15498501280115917, 5.764243146453090105, 5.045733045595949484 ) ) ;
#1887=CARTESIAN_POINT ( 'NONE',  ( -10.19094141768317741, -23.80360840875937001, 5.231925497173365081 ) ) ;
#1890=CARTESIAN_POINT ( 'NONE',  ( 10.55905858231679595, -21.25705176302045274, 4.171265325393551215 ) ) ;
#1891=CARTESIAN_POINT ( 'NONE',  ( -7.847191417683176518, -21.22443879296941915, 1.770995438708345748 ) ) ;
#1894=CARTESIAN_POINT ( 'NONE',  ( 13.37499999998404121, -20.24999999996810729, 2.793053905886972998 ) ) ;
#1903=CARTESIAN_POINT ( 'NONE',  ( -12.79798428357658047, -11.51429367935891790, 5.673858176248284479 ) ) ;
#1904=CARTESIAN_POINT ( 'NONE',  ( 9.059058582316794173, -20.72672167713054137, 4.701595411283463477 ) ) ;
#1906=CARTESIAN_POINT ( 'NONE',  ( 12.62745083560477966, -20.12623280195927933, 5.001038150054709419 ) ) ;
#1911=CARTESIAN_POINT ( 'NONE',  ( -13.86693669322925260, 4.592803008081209448, 5.801483467520450077 ) ) ;
#1914=CARTESIAN_POINT ( 'NONE',  ( 9.253441417683177406, -21.94931252712233061, 1.749999999999998446 ) ) ;
#1915=CARTESIAN_POINT ( 'NONE',  ( -8.965308582316795949, -20.97900456129165647, 3.863526089495444626 ) ) ;
#1917=CARTESIAN_POINT ( 'NONE',  ( 13.90439735423812273, 5.734566389025032684, 4.916666666666649199 ) ) ;
#1918=CARTESIAN_POINT ( 'NONE',  ( 13.12503131243110843, 5.001581277770153378, 5.166347330538456184 ) ) ;
#1919=CARTESIAN_POINT ( 'NONE',  ( -13.19540963423371949, -19.91531415481216882, 3.473342506385693085 ) ) ;
#1920=EDGE_LOOP ( 'NONE', ( #602, #17525, #19374, #11232, #9716 ) ) ;
#1921=ORIENTED_EDGE ( 'NONE', *, *, #12222, .T. ) ;
#1926=CARTESIAN_POINT ( 'NONE',  ( 1.862510824048270619, -9.990417728039201251, 2.404874838918925395 ) ) ;
#1932=CARTESIAN_POINT ( 'NONE',  ( -13.37155858231679417, -20.24999999999999289, 3.449312527122348371 ) ) ;
#1933=CARTESIAN_POINT ( 'NONE',  ( -3.379380450443691952, -10.24275229525297348, 2.854909362179569587 ) ) ;
#1935=CARTESIAN_POINT ( 'NONE',  ( -12.62966097655984754, -19.26462068372267566, 4.756751955311774083 ) ) ;
#1936=CARTESIAN_POINT ( 'NONE',  ( -6.527808582316795949, -22.97900456129165647, 3.964901035250747885 ) ) ;
#1938=CARTESIAN_POINT ( 'NONE',  ( -8.597191417683177406, -22.77556120703057729, 5.229004561291655584 ) ) ;
#1939=VERTEX_POINT ( 'NONE', #10579 ) ;
#1940=CARTESIAN_POINT ( 'NONE',  ( 13.84501469867711698, 4.235742283194553259, 4.791666666666684726 ) ) ;
#1944=PLANE ( 'NONE',  #19092 ) ;
#1952=CARTESIAN_POINT ( 'NONE',  ( 6.159691417683176518, -22.67418626127524917, 1.729004561291651587 ) ) ;
#1954=CARTESIAN_POINT ( 'NONE',  ( -2.534747216115884161, -9.671180236796224960, 2.515503256513427210 ) ) ;
#1955=CARTESIAN_POINT ( 'NONE',  ( 1.904508877737772998, -9.138371295333994837, 2.378667276417936627 ) ) ;
#1956=CARTESIAN_POINT ( 'NONE',  ( -5.684058582316794173, -20.79840458871652942, 2.226721677130544030 ) ) ;
#1959=CARTESIAN_POINT ( 'NONE',  ( 6.253441417683176518, -21.94931252712233061, 1.749999999999998446 ) ) ;
#1961=CARTESIAN_POINT ( 'NONE',  ( -10.65969141768317741, -22.36352608949543352, 2.479004561291652031 ) ) ;
#1964=CARTESIAN_POINT ( 'NONE',  ( 9.527808582316795949, -24.47900456129166358, 4.586221378810390270 ) ) ;
#1965=CARTESIAN_POINT ( 'NONE',  ( 13.06655316810189227, 2.048434989138931961, 5.965524842914772030 ) ) ;
#1966=CARTESIAN_POINT ( 'NONE',  ( -13.11824772738305356, 3.909010232842670796, 6.755569162489314827 ) ) ;
#1975=CARTESIAN_POINT ( 'NONE',  ( 13.30678549240874275, -20.03395411350983935, 3.458247869257524254 ) ) ;
#1981=CARTESIAN_POINT ( 'NONE',  ( 12.62500000000001954, -20.25000000000274269, 4.083333333315724012 ) ) ;
#1983=CARTESIAN_POINT ( 'NONE',  ( -13.37515323800563039, -20.24226148071262799, 4.627790572011877934 ) ) ;
#1985=CARTESIAN_POINT ( 'NONE',  ( 11.40280858231679595, -23.08622137881038938, 1.020995438708339309 ) ) ;
#1986=CARTESIAN_POINT ( 'NONE',  ( -12.92761177809936513, -5.718105205959081339, 6.548537912490751900 ) ) ;
#1987=CARTESIAN_POINT ( 'NONE',  ( -4.840308582316795061, -22.98484643305508612, 6.020995438708344416 ) ) ;
#1993=CARTESIAN_POINT ( 'NONE',  ( 9.434058582316795949, -22.67126532539354855, 4.242948236979545484 ) ) ;
#1994=CARTESIAN_POINT ( 'NONE',  ( -9.253441417683177406, -21.94931252712233061, 1.749999999999998446 ) ) ;
#1997=CARTESIAN_POINT ( 'NONE',  ( 13.38800411018677572, -19.59329243556743805, 5.436267741224407146 ) ) ;
#2004=CARTESIAN_POINT ( 'NONE',  ( 13.84264281492353987, 3.365962153638767607, 5.979325532956542233 ) ) ;
#2008=CARTESIAN_POINT ( 'NONE',  ( 1.337453470010121714, -8.364917468222230923, 2.372643865078341019 ) ) ;
#2010=CARTESIAN_POINT ( 'NONE',  ( 1.126276606324276619, -9.114917468222230923, 1.622643865078341463 ) ) ;
#2011=CARTESIAN_POINT ( 'NONE',  ( -13.10431844137356627, 3.955581289335645234, 6.006545679920360925 ) ) ;
#2012=CARTESIAN_POINT ( 'NONE',  ( 8.309058582316792396, -23.27327832286945153, 2.298404588716537411 ) ) ;
#2014=CARTESIAN_POINT ( 'NONE',  ( 12.63249216759192350, -19.87164553660301536, 5.297612231341934041 ) ) ;
#2015=CARTESIAN_POINT ( 'NONE',  ( -2.602174906157317835, -9.976397331638239052, 2.593889103792902606 ) ) ;
#2018=CARTESIAN_POINT ( 'NONE',  ( 7.753441417683176518, -21.94931252712233061, 1.749999999999998446 ) ) ;
#2019=CARTESIAN_POINT ( 'NONE',  ( -8.590308582316797725, -21.63647391050454871, 2.479004561291657804 ) ) ;
#2021=CARTESIAN_POINT ( 'NONE',  ( 13.90439735423812273, 5.734566389025032684, 4.833333333333343695 ) ) ;
#2022=CARTESIAN_POINT ( 'NONE',  ( 12.65051119073526564, -18.96168486786632457, 5.513701926248478102 ) ) ;
#2032=CARTESIAN_POINT ( 'NONE',  ( 2.340131407102140848, -12.21153219924485889, 2.225301406344140531 ) ) ;
#2036=( GEOMETRIC_REPRESENTATION_CONTEXT ( 3 ) GLOBAL_UNCERTAINTY_ASSIGNED_CONTEXT ( ( #2529 ) ) GLOBAL_UNIT_ASSIGNED_CONTEXT ( ( #17942, #5282, #9892 ) ) REPRESENTATION_CONTEXT ( 'NONE', 'WORKASPACE' ) );
#2038=CARTESIAN_POINT ( 'NONE',  ( 13.25854700851012424, -20.52162993467030461, 3.464734827531053440 ) ) ;
#2039=CARTESIAN_POINT ( 'NONE',  ( -2.534747216115884161, -9.671180236796224960, 2.515503256513427210 ) ) ;
#2040=CARTESIAN_POINT ( 'NONE',  ( -7.277808582316794173, -20.27099543870833642, 2.724438792969431589 ) ) ;
#2043=CARTESIAN_POINT ( 'NONE',  ( 0.000000000000000000, -8.364917468222230923, 2.372643865078341019 ) ) ;
#2046=CARTESIAN_POINT ( 'NONE',  ( -12.62500797102436678, -19.49959746326937093, 4.516621614626514791 ) ) ;
#2047=CARTESIAN_POINT ( 'NONE',  ( -6.809058582316794173, -23.27327832286945153, 2.298404588716537411 ) ) ;
#2048=CARTESIAN_POINT ( 'NONE',  ( -6.815941417683176518, -20.79840458871654363, 4.773278322869464851 ) ) ;
#2050=CARTESIAN_POINT ( 'NONE',  ( 13.39888564296547635, -18.29377503024027263, 4.763499963382565205 ) ) ;
#2059=CARTESIAN_POINT ( 'NONE',  ( 5.878441417683177406, -23.74999999999999645, 3.449312527122335492 ) ) ;
#2067=CARTESIAN_POINT ( 'NONE',  ( 11.87844141768317563, -23.74999999999999645, 3.449312527122335492 ) ) ;
#2069=CARTESIAN_POINT ( 'NONE',  ( -5.690941417683176518, -23.27327832286946219, 4.701595411283453707 ) ) ;
#2071=CARTESIAN_POINT ( 'NONE',  ( -7.371558582316795949, -19.49999999999998934, 3.449312527122348371 ) ) ;
#2073=CARTESIAN_POINT ( 'NONE',  ( 12.63249216759192350, -19.87164553660301536, 5.297612231341934041 ) ) ;
#2074=CARTESIAN_POINT ( 'NONE',  ( -12.62500000000001954, -20.25000000000274269, 4.083333333315724012 ) ) ;
#2081=CARTESIAN_POINT ( 'NONE',  ( 12.74155597218489078, -19.97827208673946231, 3.535251045670558145 ) ) ;
#2088=CARTESIAN_POINT ( 'NONE',  ( 12.62745083560477966, -20.12623280195927933, 5.001038150054709419 ) ) ;
#2090=CARTESIAN_POINT ( 'NONE',  ( 7.277808582316795061, -19.52099543870833642, 2.413778621189609286 ) ) ;
#2092=CARTESIAN_POINT ( 'NONE',  ( -13.10026320386584153, 3.000791795219782454, 6.736037912489353019 ) ) ;
#2093=CARTESIAN_POINT ( 'NONE',  ( -10.47219141768317741, -24.47900456129165292, 2.413778621189595963 ) ) ;
#2097=CARTESIAN_POINT ( 'NONE',  ( 9.621558582316795949, -22.99999999999999645, 3.550687472877652073 ) ) ;
#2098=CARTESIAN_POINT ( 'NONE',  ( -4.003441417683176518, -22.05068747287765873, 5.250000000000000888 ) ) ;
#2101=CARTESIAN_POINT ( 'NONE',  ( 13.39359219590679295, -19.31109410670777038, 5.491647114909025795 ) ) ;
#2107=CARTESIAN_POINT ( 'NONE',  ( 13.38921792038197900, -19.53199502070850357, 5.456033026503027017 ) ) ;
#2111=CARTESIAN_POINT ( 'NONE',  ( 2.910499702382182807, -8.879427762644468203, 2.504780387061739333 ) ) ;
#2114=CARTESIAN_POINT ( 'NONE',  ( -12.82182472306881671, -9.560351485048736109, 4.965845106672846399 ) ) ;
#2115=CARTESIAN_POINT ( 'NONE',  ( 6.246558582316794173, -21.94931252712234482, 5.250000000000000888 ) ) ;
#2117=CARTESIAN_POINT ( 'NONE',  ( 13.10756170493883310, 4.119366099410778581, 6.001761809183453700 ) ) ;
#2118=CARTESIAN_POINT ( 'NONE',  ( -2.559937518207947793, -9.746075135043517079, 2.534737762559237773 ) ) ;
#2119=CARTESIAN_POINT ( 'NONE',  ( 7.090308582316795061, -21.63647391050454871, 2.479004561291657804 ) ) ;
#2120=CARTESIAN_POINT ( 'NONE',  ( 12.06594141768317563, -23.20159541128344927, 2.226721677130534705 ) ) ;
#2122=CARTESIAN_POINT ( 'NONE',  ( -6.246558582316795949, -21.94931252712234127, 4.499999999999999112 ) ) ;
#2124=CARTESIAN_POINT ( 'NONE',  ( 13.10026320386584153, 3.000791795219782454, 6.736037912489353019 ) ) ;
#2125=CARTESIAN_POINT ( 'NONE',  ( 12.62515856830665584, -19.49199230051052822, 4.565864671500353467 ) ) ;
#2126=CARTESIAN_POINT ( 'NONE',  ( -12.66618699081223198, -20.05307589586896455, 3.545538277555074114 ) ) ;
#2128=ORIENTED_EDGE ( 'NONE', *, *, #1216, .F. ) ;
#2135=CARTESIAN_POINT ( 'NONE',  ( 1.707060460004204527, -9.864918773552613374, 2.372644200313257290 ) ) ;
#2140=CARTESIAN_POINT ( 'NONE',  ( -8.027808582316792396, -23.72900456129165647, 4.275561207030568411 ) ) ;
#2141=CARTESIAN_POINT ( 'NONE',  ( -2.445888733774860935, -8.532121313016713060, 2.415585152653916712 ) ) ;
#2143=CARTESIAN_POINT ( 'NONE',  ( -13.38090111944825367, -19.20199346786276351, 4.743968713382380464 ) ) ;
#2144=CARTESIAN_POINT ( 'NONE',  ( -5.215308582316793284, -23.77099543870833998, 2.825813738724734847 ) ) ;
#2146=CARTESIAN_POINT ( 'NONE',  ( -10.09719141768317741, -22.77556120703057729, 5.229004561291655584 ) ) ;
#2148=CARTESIAN_POINT ( 'NONE',  ( 13.84501469867711698, 4.235742283194553259, 4.166666666666765551 ) ) ;
#2154=CARTESIAN_POINT ( 'NONE',  ( -13.37499999999995026, -20.24999999999991829, 3.465895369911768054 ) ) ;
#2156=CARTESIAN_POINT ( 'NONE',  ( 3.974842109207561425, -21.82955800590261930, 5.256404853634145447 ) ) ;
#2159=CARTESIAN_POINT ( 'NONE',  ( 2.817596665886821672, -11.50588678273290988, 2.986692549455723267 ) ) ;
#2161=CARTESIAN_POINT ( 'NONE',  ( 12.62500028073152869, -20.99998582305707728, 4.544498183892649479 ) ) ;
#2163=CARTESIAN_POINT ( 'NONE',  ( 10.65969141768318096, -22.67418626127524917, 1.729004561291651809 ) ) ;
#2165=CARTESIAN_POINT ( 'NONE',  ( -5.315941417683176518, -21.32873467460645145, 4.242948236979555254 ) ) ;
#2166=CARTESIAN_POINT ( 'NONE',  ( -11.12155858231679595, -24.50000000000000000, 3.550687472877651629 ) ) ;
#2168=CARTESIAN_POINT ( 'NONE',  ( 12.62500000000001954, -20.25000000000274269, 4.083333333315724012 ) ) ;
#2169=CARTESIAN_POINT ( 'NONE',  ( -13.11465082267961968, 3.727366545318180791, 6.751662912489328150 ) ) ;
#2177=AXIS2_PLACEMENT_3D ( 'NONE', #14012, #18844, #20307 ) ;
#2181=CARTESIAN_POINT ( 'NONE',  ( 13.11740841389447709, 4.616624901677048420, 5.813473370769506765 ) ) ;
#2182=CARTESIAN_POINT ( 'NONE',  ( -1.126276606324276619, -8.364917468222230923, 1.622643865078341907 ) ) ;
#2185=CARTESIAN_POINT ( 'NONE',  ( 12.72125031657057015, -15.38935901321805133, 5.590524842915047365 ) ) ;
#2187=CARTESIAN_POINT ( 'NONE',  ( 11.12155858231679595, -24.50000000000000000, 3.550687472877651629 ) ) ;
#2188=CARTESIAN_POINT ( 'NONE',  ( -12.96597876160390683, -3.780572539034193102, 6.590204579154564257 ) ) ;
#2189=CARTESIAN_POINT ( 'NONE',  ( -4.472191417683178294, -24.47900456129165292, 2.413778621189595963 ) ) ;
#2194=CARTESIAN_POINT ( 'NONE',  ( 6.809058582316796837, -22.74294823697954016, 2.828734674606448785 ) ) ;
#2198=CARTESIAN_POINT ( 'NONE',  ( 13.85980676119184629, 4.232741440188380722, 5.965367510457697975 ) ) ;
#2207=CARTESIAN_POINT ( 'NONE',  ( 13.38450946332969771, -19.76977210184853462, 5.359796180098093998 ) ) ;
#2209=CARTESIAN_POINT ( 'NONE',  ( 0.5631383031621635116, -8.364917468222230923, 2.372643865078341019 ) ) ;
#2211=CARTESIAN_POINT ( 'NONE',  ( -13.12529380813666435, 5.014837310896125722, 5.033295791462342628 ) ) ;
#2212=CARTESIAN_POINT ( 'NONE',  ( 6.621558582316794173, -23.74999999999999645, 3.550687472877651629 ) ) ;
#2214=CARTESIAN_POINT ( 'NONE',  ( 12.63465172146706728, -19.76258806590802664, 5.372658420469845986 ) ) ;
#2215=CARTESIAN_POINT ( 'NONE',  ( -3.162271481458107658, -13.95306990448253437, 3.615178062515473911 ) ) ;
#2216=CARTESIAN_POINT ( 'NONE',  ( 11.30905858231679595, -22.74294823697954016, 2.828734674606448785 ) ) ;
#2218=CARTESIAN_POINT ( 'NONE',  ( 9.440941417683177406, -20.72672167713052715, 2.298404588716546293 ) ) ;
#2219=CARTESIAN_POINT ( 'NONE',  ( -11.12155858231679417, -23.74999999999999645, 3.550687472877651629 ) ) ;
#2221=CARTESIAN_POINT ( 'NONE',  ( 12.65346245025441263, -19.56264626215117275, 6.228892365149262922 ) ) ;
#2222=CARTESIAN_POINT ( 'NONE',  ( 12.62499999999998224, -19.49999999999991473, 4.333333333333343695 ) ) ;
#2225=EDGE_LOOP ( 'NONE', ( #1668, #20220, #7372, #9771, #20404 ) ) ;
#2231=CARTESIAN_POINT ( 'NONE',  ( 2.583953725994688533, -9.847075946378776479, 2.560676788604062004 ) ) ;
#2236=CARTESIAN_POINT ( 'NONE',  ( -6.621558582316794173, -23.74999999999999645, 3.550687472877651629 ) ) ;
#2237=CARTESIAN_POINT ( 'NONE',  ( -2.910499702382182807, -8.879427762644468203, 2.504780387061739333 ) ) ;
#2239=CARTESIAN_POINT ( 'NONE',  ( -13.09556065010287362, 4.263312830196960057, 5.034075356110313315 ) ) ;
#2240=CARTESIAN_POINT ( 'NONE',  ( -9.340308582316794173, -22.67418626127525982, 5.270995438708342640 ) ) ;
#2242=CARTESIAN_POINT ( 'NONE',  ( -8.034691417683175629, -20.22900456129164581, 2.825813738724747726 ) ) ;
#2245=CARTESIAN_POINT ( 'NONE',  ( 13.75871503850933841, -0.8723905552644914962, 5.888179699623941943 ) ) ;
#2246=FACE_OUTER_BOUND ( 'NONE', #1920, .T. ) ;
#2251=CARTESIAN_POINT ( 'NONE',  ( -13.37499999999998224, -20.24999999999998934, 4.291666666666698937 ) ) ;
#2253=CARTESIAN_POINT ( 'NONE',  ( 7.378441417683176518, -23.74999999999999645, 3.449312527122335492 ) ) ;
#2257=CARTESIAN_POINT ( 'NONE',  ( 3.549867680106858714, -10.29705900472337632, 2.118856410057032402 ) ) ;
#2258=CARTESIAN_POINT ( 'NONE',  ( -8.402808582316792396, -22.77556120703056308, 1.770995438708340197 ) ) ;
#2259=CARTESIAN_POINT ( 'NONE',  ( 13.90439706815434739, 5.734551941788608609, 5.045486763335835789 ) ) ;
#2261=CARTESIAN_POINT ( 'NONE',  ( 5.784691417683179182, -23.77099543870834353, 4.174186261275252718 ) ) ;
#2262=CARTESIAN_POINT ( 'NONE',  ( -12.64571531779736979, -19.20387645123237164, 5.508493592915143289 ) ) ;
#2263=CARTESIAN_POINT ( 'NONE',  ( -6.159691417683175629, -22.36352608949543352, 2.479004561291652031 ) ) ;
#2264=CARTESIAN_POINT ( 'NONE',  ( -8.684058582316795949, -20.26807450282662160, 1.696391591240633101 ) ) ;
#2266=CARTESIAN_POINT ( 'NONE',  ( 13.12424783836753228, 4.962015837561366993, 5.328858059679200565 ) ) ;
#2267=CARTESIAN_POINT ( 'NONE',  ( -12.64387510712649565, -19.29680709011273976, 5.506486987317513737 ) ) ;
#2274=CARTESIAN_POINT ( 'NONE',  ( 12.73854111515253607, -19.98117175391610090, 3.535666685490541639 ) ) ;
#2276=FACE_OUTER_BOUND ( 'NONE', #13922, .T. ) ;
#2278=CARTESIAN_POINT ( 'NONE',  ( 12.95145221759166354, -3.764163011652346569, 5.840524842913703552 ) ) ;
#2280=CARTESIAN_POINT ( 'NONE',  ( -2.916276642307554123, -11.05036367517186058, 2.119705115445599475 ) ) ;
#2285=CARTESIAN_POINT ( 'NONE',  ( 11.31594141768317741, -20.26807450282663225, 5.303608408759377113 ) ) ;
#2286=CARTESIAN_POINT ( 'NONE',  ( -13.12526104302547836, 5.013182672784613381, 5.066812735559260261 ) ) ;
#2287=CARTESIAN_POINT ( 'NONE',  ( -7.003441417683177406, -22.05068747287766229, 6.000000000000001776 ) ) ;
#2288=VERTEX_POINT ( 'NONE', #6896 ) ;
#2289=CARTESIAN_POINT ( 'NONE',  ( 10.84030858231679240, -22.67418626127525982, 5.270995438708342640 ) ) ;
#2291=CARTESIAN_POINT ( 'NONE',  ( -13.87470602645761986, 4.985154336109792972, 4.666666666666619889 ) ) ;
#2293=CARTESIAN_POINT ( 'NONE',  ( 8.121558582316795949, -22.99999999999999645, 3.550687472877652073 ) ) ;
#2298=CARTESIAN_POINT ( 'NONE',  ( 13.86470821076586368, 4.480264643675554659, 5.874551681240599343 ) ) ;
#2304=CARTESIAN_POINT ( 'NONE',  ( 13.37561105820882013, -20.21914156045197686, 4.753815841436231260 ) ) ;
#2308=CARTESIAN_POINT ( 'NONE',  ( 3.379380450443691952, -10.24275229525297348, 2.854909362179569587 ) ) ;
#2312=CARTESIAN_POINT ( 'NONE',  ( -12.62500004114794372, -19.49999792202770621, 4.520295319612473328 ) ) ;
#2314=CARTESIAN_POINT ( 'NONE',  ( 13.10624331898488037, 4.052787608736739600, 6.006964772046813117 ) ) ;
#2315=CARTESIAN_POINT ( 'NONE',  ( -2.513306525444908512, -9.622685169956881168, 2.503048754562789746 ) ) ;
#2317=CARTESIAN_POINT ( 'NONE',  ( 8.777808582316797725, -21.02099543870833998, 3.035098964749253003 ) ) ;
#2319=CARTESIAN_POINT ( 'NONE',  ( 7.565941417683176518, -23.20159541128344927, 2.226721677130534705 ) ) ;
#2320=CARTESIAN_POINT ( 'NONE',  ( -7.840308582316794173, -22.67418626127525982, 5.270995438708342640 ) ) ;
#2322=CARTESIAN_POINT ( 'NONE',  ( 12.69740987707854707, -17.34330120752609616, 6.298537912489285517 ) ) ;
#2323=CARTESIAN_POINT ( 'NONE',  ( 12.99447614883396973, -0.8414544838704021146, 5.153345106674984244 ) ) ;
#2326=UNCERTAINTY_MEASURE_WITH_UNIT (LENGTH_MEASURE( 1.000000000000000082E-05 ), #12848, 'distance_accuracy_value', 'NONE');
#2335=CARTESIAN_POINT ( 'NONE',  ( 2.602174906157317835, -9.976397331638239052, 2.593889103792902606 ) ) ;
#2340=CARTESIAN_POINT ( 'NONE',  ( -5.309058582316794173, -23.27327832286945153, 2.298404588716537411 ) ) ;
#2341=CARTESIAN_POINT ( 'NONE',  ( -3.882031223148668886, -13.81156101447257889, 3.771450735391772557 ) ) ;
#2343=CARTESIAN_POINT ( 'NONE',  ( -13.37559048950600626, -19.47018027994350220, 4.620717101209816491 ) ) ;
#2344=CARTESIAN_POINT ( 'NONE',  ( -9.809058582316794173, -23.27327832286945153, 2.298404588716537411 ) ) ;
#2346=CARTESIAN_POINT ( 'NONE',  ( 8.027808582316795949, -24.47900456129166358, 4.586221378810390270 ) ) ;
#2347=CARTESIAN_POINT ( 'NONE',  ( -8.503441417683177406, -22.05068747287766229, 4.499999999999999112 ) ) ;
#2349=CARTESIAN_POINT ( 'NONE',  ( 13.83544900551672185, 3.002674778589386140, 5.971513032956590195 ) ) ;
#2350=DIRECTION ( 'NONE',  ( 1.000000000000000000, 0.000000000000000000, 0.000000000000000000 ) ) ;
#2360=DIRECTION ( 'NONE',  ( 0.000000000000000000, 0.2487476929738665354, 0.9685683172808094987 ) ) ;
#2366=CARTESIAN_POINT ( 'NONE',  ( 1.884282074604925583, -8.375506800461993251, 2.375363417140690547 ) ) ;
#2369=CARTESIAN_POINT ( 'NONE',  ( 12.62499999999998401, -20.99999999999999645, 3.146526952850934755 ) ) ;
#2371=CARTESIAN_POINT ( 'NONE',  ( 5.409691417683178294, -21.32581373872474373, 5.270995438708348857 ) ) ;
#2373=CARTESIAN_POINT ( 'NONE',  ( -7.847191417683175629, -21.53509896474923835, 2.520995438708346192 ) ) ;
#2374=CARTESIAN_POINT ( 'NONE',  ( -12.15969141768317918, -22.98484643305507191, 0.9790045612916508100 ) ) ;
#2376=CARTESIAN_POINT ( 'NONE',  ( 12.63478567848856571, -19.00582323632600890, 4.762720106674273701 ) ) ;
#2377=CARTESIAN_POINT ( 'NONE',  ( -13.10821839766814279, 4.152529082241303904, 5.997503362667785609 ) ) ;
#2382=B_SPLINE_CURVE_WITH_KNOTS ( 'NONE', 3,
 ( #3343, #3238, #8058, #9312, #12753, #11095, #3041, #19356, #106, #6492, #10988, #4596, #17780, #1370, #3142, #9722, #15887, #7942, #18941, #7751, #20522, #9419, #6175, #14312, #19156, #4811, #11190, #17565, #9610, #3447, #16599, #5527, #18092, #7000, #14738, #19464, #11800, #16210, #3649, #8669, #3854, #13261, #2278, #8469, #5216, #414, #13063, #723, #19770, #5119, #9825, #1877, #10135, #19657, #6892, #15039, #3757, #11898, #14838, #16507, #17978, #8260, #14625, #10031, #2181, #13367, #5429, #6796, #308, #17879, #18189, #5322, #512, #11694, #10233, #7107, #13164, #19563, #6693, #11499, #8564, #13471 ),
 .UNSPECIFIED., .F., .F.,
 ( 4, 2, 2, 2, 2, 2, 2, 2, 2, 2, 2, 2, 2, 2, 2, 2, 2, 2, 2, 2, 2, 2, 2, 2, 2, 2, 2, 2, 2, 2, 2, 2, 2, 2, 2, 2, 2, 2, 2, 2, 4 ),
 ( 0.03648247254878290990, 0.05122453910963482848, 0.05943139484297973313, 0.06353482270965218892, 0.06763825057632463778, 0.07081696859385248899, 0.07399568661138034020, 0.08035312264643605651, 0.09306799471654747524, 0.1057828667866588801, 0.1121403028217145964, 0.1153190208392424337, 0.1184977388567702850, 0.1214804596100246964, 0.1244631803632790940, 0.1304286218697879030, 0.1423595048828055210, 0.1662212709088407014, 0.2139448029609111179, 0.3093918670650518954, 0.5002859952733336169, 0.6911801234816151718, 0.7866271875857560048, 0.8343507196378263657, 0.8582124856638615462, 0.8701433686768791365, 0.8761088101833880426, 0.8790915309366424957, 0.8820742516898969487, 0.8853411830926060100, 0.8886081144953148492, 0.8951419773007329717, 0.9082097029115692166, 0.9212774285224054616, 0.9278112913278236951, 0.9310782227305326453, 0.9343451541332417065, 0.9384485819999140999, 0.9425520098665866042, 0.9507588655999313909, 0.9671725770666211863 ),
 .UNSPECIFIED. ) ;
#2389=CARTESIAN_POINT ( 'NONE',  ( -2.808565762442263303, -10.28561894962424716, 1.923303392614186924 ) ) ;
#2395=CARTESIAN_POINT ( 'NONE',  ( 4.840308582316795061, -22.98484643305508612, 6.020995438708344416 ) ) ;
#2396=CARTESIAN_POINT ( 'NONE',  ( -13.05696142222617695, 1.564051822406025583, 5.955108176248398166 ) ) ;
#2397=CARTESIAN_POINT ( 'NONE',  ( -7.284691417683176518, -24.52099543870834708, 4.484846433055073689 ) ) ;
#2399=CARTESIAN_POINT ( 'NONE',  ( 10.55905858231679595, -20.72672167713054137, 4.701595411283463477 ) ) ;
#2401=CARTESIAN_POINT ( 'NONE',  ( -13.40322194933353828, -19.57479155865495457, 6.214283636730510096 ) ) ;
#2402=EDGE_CURVE ( 'NONE', #19322, #8256, #5179, .T. ) ;
#2403=CARTESIAN_POINT ( 'NONE',  ( 5.684058582316795949, -21.32873467460644079, 2.757051763020455404 ) ) ;
#2407=CARTESIAN_POINT ( 'NONE',  ( 13.40022353639839103, -18.97621141187856608, 5.498856782956575984 ) ) ;
#2414=CARTESIAN_POINT ( 'NONE',  ( 13.37500015856764435, -20.24999199233421265, 4.532157119432948633 ) ) ;
#2416=CARTESIAN_POINT ( 'NONE',  ( 1.407845757905374695, -8.364917468222230923, 2.372643865078341019 ) ) ;
#2418=CARTESIAN_POINT ( 'NONE',  ( -12.62506359033936754, -19.49678868786235597, 4.541393094775662220 ) ) ;
#2420=CARTESIAN_POINT ( 'NONE',  ( 11.40280858231679417, -22.77556120703056308, 1.770995438708339975 ) ) ;
#2421=CARTESIAN_POINT ( 'NONE',  ( -13.38172782443493602, -20.66024486603417643, 5.557997437521964734 ) ) ;
#2424=CARTESIAN_POINT ( 'NONE',  ( 4.717959273841179524, -21.82295283170803302, 4.493595146365858994 ) ) ;
#2425=CARTESIAN_POINT ( 'NONE',  ( 11.03469141768317741, -20.97900456129164581, 3.136473910504570917 ) ) ;
#2426=CARTESIAN_POINT ( 'NONE',  ( -13.37155858231679417, -20.24999999999999289, 3.449312527122348371 ) ) ;
#2428=CARTESIAN_POINT ( 'NONE',  ( 12.73577686058281344, -15.40576854059989920, 6.340204579155907183 ) ) ;
#2429=CARTESIAN_POINT ( 'NONE',  ( 12.62500000000002132, -19.49999999999450040, 3.833333333368183382 ) ) ;
#2439=CARTESIAN_POINT ( 'NONE',  ( 1.957016269584227031, -9.152392576945766578, 2.382268221639079364 ) ) ;
#2443=CARTESIAN_POINT ( 'NONE',  ( -7.652808582316795061, -21.22443879296942626, 5.229004561291659137 ) ) ;
#2444=CARTESIAN_POINT ( 'NONE',  ( -1.513434189748285918, -8.364917468222230923, 1.622643865078341907 ) ) ;
#2446=CARTESIAN_POINT ( 'NONE',  ( -13.37499999999998401, -19.49999999999998934, 3.666666666666654084 ) ) ;
#2447=CARTESIAN_POINT ( 'NONE',  ( -5.402808582316794173, -22.77556120703056308, 1.770995438708339975 ) ) ;
#2448=CARTESIAN_POINT ( 'NONE',  ( 8.402808582316797725, -23.08622137881038938, 1.020995438708339309 ) ) ;
#2449=CARTESIAN_POINT ( 'NONE',  ( -10.28469141768317741, -23.02099543870834353, 3.863526089495429972 ) ) ;
#2451=CARTESIAN_POINT ( 'NONE',  ( 13.85788212999909419, 4.135547564954428879, 5.982801014393342776 ) ) ;
#2465=CARTESIAN_POINT ( 'NONE',  ( 3.636036383999129207, -10.90885478516162976, 2.275977788322152584 ) ) ;
#2468=CARTESIAN_POINT ( 'NONE',  ( 13.90434039801927568, 5.731690099970989216, 5.115558489342345361 ) ) ;
#2470=CARTESIAN_POINT ( 'NONE',  ( 11.03469141768317741, -20.97900456129164581, 3.136473910504570917 ) ) ;
#2472=CARTESIAN_POINT ( 'NONE',  ( -7.753441417683177406, -21.94931252712233061, 2.499999999999999112 ) ) ;
#2473=CARTESIAN_POINT ( 'NONE',  ( -8.597191417683177406, -23.08622137881040359, 5.979004561291654696 ) ) ;
#2475=CARTESIAN_POINT ( 'NONE',  ( 13.12529397354238192, 5.014845663890295846, 4.666666666666619889 ) ) ;
#2476=CARTESIAN_POINT ( 'NONE',  ( -12.74043380832193684, -14.42059267975384529, 5.611358176248560703 ) ) ;
#2486=CARTESIAN_POINT ( 'NONE',  ( -2.747777887823422471, -9.906471667804277459, 1.825930796414880763 ) ) ;
#2489=DIRECTION ( 'NONE',  ( -1.000000000000000000, 0.000000000000000000, 0.000000000000000000 ) ) ;
#2490=CARTESIAN_POINT ( 'NONE',  ( 5.215308582316795949, -24.52099543870834708, 2.515153566944913432 ) ) ;
#2491=CARTESIAN_POINT ( 'NONE',  ( -13.08573665985359824, 3.017201322601628100, 5.986358176248492313 ) ) ;
#2492=CARTESIAN_POINT ( 'NONE',  ( -4.284691417683177406, -24.52099543870834708, 4.484846433055073689 ) ) ;
#2496=CARTESIAN_POINT ( 'NONE',  ( -13.89730118381875279, 5.376209782841177898, 6.083536567043803522 ) ) ;
#2497=CARTESIAN_POINT ( 'NONE',  ( 5.871558582316795949, -20.99999999999999645, 3.449312527122348371 ) ) ;
#2503=CARTESIAN_POINT ( 'NONE',  ( 13.87467358130843387, 4.983515856073828409, 5.065827972856573602 ) ) ;
#2511=CARTESIAN_POINT ( 'NONE',  ( 13.86470821076586368, 4.480264643675554659, 5.874551681240599343 ) ) ;
#2514=CARTESIAN_POINT ( 'NONE',  ( 3.347120161770001268, -14.10934257735911146, 2.905312006771028077 ) ) ;
#2517=CARTESIAN_POINT ( 'NONE',  ( -12.62499999999998401, -19.49999999999998934, 3.666666666666654084 ) ) ;
#2519=CARTESIAN_POINT ( 'NONE',  ( -13.41355111217617413, -19.05316883510194614, 6.247234435864091218 ) ) ;
#2521=CARTESIAN_POINT ( 'NONE',  ( 12.05905858231679417, -20.72672167713054137, 4.701595411283463477 ) ) ;
#2522=CARTESIAN_POINT ( 'NONE',  ( 4.097191417683176518, -22.77556120703057729, 5.229004561291655584 ) ) ;
#2523=CARTESIAN_POINT ( 'NONE',  ( -10.55905858231679595, -20.72672167713054137, 4.701595411283463477 ) ) ;
#2525=CARTESIAN_POINT ( 'NONE',  ( 13.04271272860988340, 0.09449279482665236263, 6.673537912489449830 ) ) ;
#2526=CARTESIAN_POINT ( 'NONE',  ( 13.09001666039658573, 3.983341349998239966, 5.257104358157307367 ) ) ;
#2529=UNCERTAINTY_MEASURE_WITH_UNIT (LENGTH_MEASURE( 1.000000000000000082E-05 ), #17942, 'distance_accuracy_value', 'NONE');
#2530=ORIENTED_EDGE ( 'NONE', *, *, #20355, .F. ) ;
#2533=CARTESIAN_POINT ( 'NONE',  ( -12.74043380832193684, -14.42059267975384529, 5.611358176248560703 ) ) ;
#2535=CARTESIAN_POINT ( 'NONE',  ( -13.41341218697771609, -18.31018455762212227, 5.513179699623425023 ) ) ;
#2538=CARTESIAN_POINT ( 'NONE',  ( 2.579281110863027582, -9.822567596814183233, 2.554382554832406615 ) ) ;
#2541=( BOUNDED_CURVE ( )  B_SPLINE_CURVE ( 3, ( #18318, #3674, #14860, #5346 ),
 .UNSPECIFIED., .F., .F. ) 
 B_SPLINE_CURVE_WITH_KNOTS ( ( 4, 4 ),
 ( 1.468430546537837468E-05, 0.001172421487176120289 ),
 .UNSPECIFIED. ) 
 CURVE ( )  GEOMETRIC_REPRESENTATION_ITEM ( )  RATIONAL_B_SPLINE_CURVE ( ( 0.9619191252709937690, 0.3335846922424353656, 0.3462783171521043313, 1.000000000000000222 ) ) 
 REPRESENTATION_ITEM ( '' )  );
#2542=CARTESIAN_POINT ( 'NONE',  ( -1.337453470010121714, -9.114917468222230923, 2.372643865078341019 ) ) ;
#2543=CARTESIAN_POINT ( 'NONE',  ( -9.434058582316795949, -23.73192549717337130, 5.303608408759367343 ) ) ;
#2544=CARTESIAN_POINT ( 'NONE',  ( -2.708677329869237482, -9.785633270066144362, 1.794897081886200230 ) ) ;
#2547=CARTESIAN_POINT ( 'NONE',  ( -13.37593719518949698, -19.45267164293252193, 4.647380496992003174 ) ) ;
#2549=CARTESIAN_POINT ( 'NONE',  ( 12.53469141768317741, -19.47900456129164581, 2.515153566944927199 ) ) ;
#2550=CARTESIAN_POINT ( 'NONE',  ( -10.37844141768317741, -22.99999999999999645, 3.449312527122335048 ) ) ;
#2553=CARTESIAN_POINT ( 'NONE',  ( 13.37499999998404121, -20.24999999996810729, 2.793053905886972998 ) ) ;
#2559=CARTESIAN_POINT ( 'NONE',  ( -13.86470821076586368, 4.480264643675554659, 5.874551681240599343 ) ) ;
#2565=CARTESIAN_POINT ( 'NONE',  ( 0.5631383031621635116, -8.364917468222230923, 2.372643865078341019 ) ) ;
#2568=CARTESIAN_POINT ( 'NONE',  ( 13.89992416064626646, 5.508670112635706495, 5.888743936161951353 ) ) ;
#2571=CARTESIAN_POINT ( 'NONE',  ( 13.12529397354238192, 5.014845663890295846, 4.833333333333344584 ) ) ;
#2572=CARTESIAN_POINT ( 'NONE',  ( 9.440941417683177406, -21.25705176302044208, 2.828734674606458555 ) ) ;
#2574=CARTESIAN_POINT ( 'NONE',  ( -7.659691417683177406, -22.36352608949543352, 2.479004561291652031 ) ) ;
#2575=CARTESIAN_POINT ( 'NONE',  ( -4.746558582316795061, -21.94931252712234127, 6.000000000000001776 ) ) ;
#2578=CARTESIAN_POINT ( 'NONE',  ( 12.62525331949183105, -19.48720736566255951, 4.581880915780448760 ) ) ;
#2579=CARTESIAN_POINT ( 'NONE',  ( -12.64571531779736979, -19.20387645123237164, 5.508493592915143289 ) ) ;
#2582=ADVANCED_FACE ( 'NONE', ( #5637 ), #18295, .T. ) ;
#2586=CARTESIAN_POINT ( 'NONE',  ( 2.534747216115884161, -9.671180236796224960, 2.515503256513427210 ) ) ;
#2591=CARTESIAN_POINT ( 'NONE',  ( -1.859341899742023463, -9.902476528685241419, 1.632289782122827271 ) ) ;
#2597=CARTESIAN_POINT ( 'NONE',  ( 5.402808582316795949, -23.08622137881038938, 1.020995438708339309 ) ) ;
#2598=CARTESIAN_POINT ( 'NONE',  ( -12.79798428357658047, -11.51429367935891790, 5.673858176248284479 ) ) ;
#2599=CARTESIAN_POINT ( 'NONE',  ( -5.222191417683177406, -19.52099543870834353, 4.586221378810406257 ) ) ;
#2601=CARTESIAN_POINT ( 'NONE',  ( 11.40280858231679417, -22.77556120703056308, 1.770995438708339975 ) ) ;
#2603=CARTESIAN_POINT ( 'NONE',  ( -13.41115317570721110, -19.17426462678482579, 6.244630269197427808 ) ) ;
#2604=CARTESIAN_POINT ( 'NONE',  ( 5.590308582316795949, -21.63647391050454871, 2.479004561291657804 ) ) ;
#2608=CARTESIAN_POINT ( 'NONE',  ( 13.50467269799730374, -14.45152875114793467, 6.346192769197517514 ) ) ;
#2615=CARTESIAN_POINT ( 'NONE',  ( -12.62155858231679417, -23.74999999999999645, 3.550687472877651629 ) ) ;
#2618=CARTESIAN_POINT ( 'NONE',  ( 2.739050625766161762, -9.875938058683834342, 1.818089155622620412 ) ) ;
#2622=CARTESIAN_POINT ( 'NONE',  ( -13.37505992445764136, -19.49697381488866554, 4.539006848837218833 ) ) ;
#2626=CARTESIAN_POINT ( 'NONE',  ( -13.37505392270939986, -20.99727690317663686, 4.612442573673130930 ) ) ;
#2630=CARTESIAN_POINT ( 'NONE',  ( 10.27780858231679417, -20.27099543870833642, 2.724438792969431589 ) ) ;
#2632=CARTESIAN_POINT ( 'NONE',  ( 11.50344141768317741, -22.05068747287766229, 4.499999999999999112 ) ) ;
#2633=CARTESIAN_POINT ( 'NONE',  ( -8.684058582316794173, -20.79840458871652942, 2.226721677130544030 ) ) ;
#2635=CARTESIAN_POINT ( 'NONE',  ( 13.37499999999998401, -19.49999999999998934, 3.146526952850934755 ) ) ;
#2642=CARTESIAN_POINT ( 'NONE',  ( -13.08094078691552831, 2.775009739235173356, 5.981149842915306714 ) ) ;
#2644=CARTESIAN_POINT ( 'NONE',  ( -2.616536356806028696, -10.07836329504444706, 2.620076000170431296 ) ) ;
#2645=CARTESIAN_POINT ( 'NONE',  ( -13.39482594849551944, -19.24878960097397140, 5.493002502378098839 ) ) ;
#2646=DIRECTION ( 'NONE',  ( 0.000000000000000000, 0.000000000000000000, 1.000000000000000000 ) ) ;
#2651=CARTESIAN_POINT ( 'NONE',  ( -4.746558582316793284, -21.94931252712234482, 5.250000000000000888 ) ) ;
#2653=CARTESIAN_POINT ( 'NONE',  ( -3.059891148793807414, -12.07002330923453570, 2.381574079220715401 ) ) ;
#2655=CARTESIAN_POINT ( 'NONE',  ( -13.84501469867711698, 4.235742283194553259, 4.833333333333343695 ) ) ;
#2657=CARTESIAN_POINT ( 'NONE',  ( 6.809058582316796837, -23.80360840875935935, 1.768074502826626260 ) ) ;
#2658=CARTESIAN_POINT ( 'NONE',  ( -10.09719141768317741, -22.46490103525075810, 4.479004561291653808 ) ) ;
#2661=CARTESIAN_POINT ( 'NONE',  ( 13.37499999999998401, -20.24999999999998934, 2.439580858552613751 ) ) ;
#2662=CYLINDRICAL_SURFACE ( 'NONE', #12380, 0.3750000000000003331 ) ;
#2669=CARTESIAN_POINT ( 'NONE',  ( -13.81626551376501588, 2.033908445126689557, 5.950679699622869911 ) ) ;
#2675=( BOUNDED_CURVE ( )  B_SPLINE_CURVE ( 3, ( #14300, #12944, #1556, #11588 ),
 .UNSPECIFIED., .F., .F. ) 
 B_SPLINE_CURVE_WITH_KNOTS ( ( 4, 4 ),
 ( 0.000000000000000000, 1.468430546537837468E-05 ),
 .UNSPECIFIED. ) 
 CURVE ( )  GEOMETRIC_REPRESENTATION_ITEM ( )  RATIONAL_B_SPLINE_CURVE ( ( 1.000000000000000000, 0.9870550161812301493, 0.9743613912715626268, 0.9619191252709974327 ) ) 
 REPRESENTATION_ITEM ( '' )  );
#2677=CARTESIAN_POINT ( 'NONE',  ( 2.787023586469211001, -10.13267000451481614, 1.884023048047904103 ) ) ;
#2683=CARTESIAN_POINT ( 'NONE',  ( 13.12529397354238192, 5.014845663890295846, 4.333333333333382775 ) ) ;
#2684=CARTESIAN_POINT ( 'NONE',  ( 12.06594141768317741, -22.67126532539353789, 2.757051763020445634 ) ) ;
#2685=CARTESIAN_POINT ( 'NONE',  ( -12.63465172146706728, -19.76258806590802664, 5.372658420469845986 ) ) ;
#2686=CARTESIAN_POINT ( 'NONE',  ( -11.59030858231679595, -21.63647391050454871, 2.479004561291657804 ) ) ;
#2687=CARTESIAN_POINT ( 'NONE',  ( -4.934058582316795061, -23.73192549717337130, 5.303608408759367343 ) ) ;
#2689=CARTESIAN_POINT ( 'NONE',  ( 13.12529397353891270, 5.014845663890295846, 3.333333333333220239 ) ) ;
#2690=CARTESIAN_POINT ( 'NONE',  ( -13.12529397354238192, 5.014845663890295846, 3.000000000000000000 ) ) ;
#2696=CARTESIAN_POINT ( 'NONE',  ( 2.731427961995660958, -10.89409100229510052, 2.829571171190552015 ) ) ;
#2699=EDGE_CURVE ( 'NONE', #8463, #13542, #4343, .T. ) ;
#2704=CARTESIAN_POINT ( 'NONE',  ( -2.442511739767545098, -14.09457879449248807, 3.458905389639174821 ) ) ;
#2709=CARTESIAN_POINT ( 'NONE',  ( 4.687312169500634340, -21.32903648725300272, 5.908812401261035241 ) ) ;
#2710=CARTESIAN_POINT ( 'NONE',  ( -12.63943061533661982, -19.52125392549825733, 5.470334935344855154 ) ) ;
#2711=CARTESIAN_POINT ( 'NONE',  ( -3.944195004867014909, -21.42722504787766624, 5.934029185143018914 ) ) ;
#2717=CARTESIAN_POINT ( 'NONE',  ( -13.40957725085194241, -19.25384883197511243, 6.242932005802575901 ) ) ;
#2718=CARTESIAN_POINT ( 'NONE',  ( 13.18405858231679417, -20.79840458871652942, 2.226721677130544030 ) ) ;
#2722=CARTESIAN_POINT ( 'NONE',  ( 13.39169349927020569, -20.15697828685464188, 6.009339318877812808 ) ) ;
#2726=CARTESIAN_POINT ( 'NONE',  ( -4.315753587183824180, -21.56469153729574018, 5.194994555241421175 ) ) ;
#2728=CARTESIAN_POINT ( 'NONE',  ( -11.68405858231679417, -20.79840458871652942, 2.226721677130544030 ) ) ;
#2734=CARTESIAN_POINT ( 'NONE',  ( 2.309828811027716977, -9.292785183284841821, 1.668323847571005603 ) ) ;
#2737=CARTESIAN_POINT ( 'NONE',  ( -13.37559048950600626, -19.47018027994350220, 4.620717101209816491 ) ) ;
#2739=CARTESIAN_POINT ( 'NONE',  ( -13.37500027835944039, -20.99998594284889464, 4.544258551573043370 ) ) ;
#2741=CARTESIAN_POINT ( 'NONE',  ( 6.621558582316796837, -22.99999999999999645, 3.550687472877652073 ) ) ;
#2743=CARTESIAN_POINT ( 'NONE',  ( 11.40969141768317918, -21.63647391050456648, 4.520995438708348857 ) ) ;
#2744=CARTESIAN_POINT ( 'NONE',  ( -11.59719141768317563, -22.77556120703057729, 5.229004561291656472 ) ) ;
#2746=CARTESIAN_POINT ( 'NONE',  ( 13.37499994994395891, -19.50000252782794519, 4.474109982178703149 ) ) ;
#2750=VERTEX_POINT ( 'NONE', #11345 ) ;
#2754=CARTESIAN_POINT ( 'NONE',  ( -12.62888984277510218, -20.05356293986039873, 5.111704976569332537 ) ) ;
#2756=CARTESIAN_POINT ( 'NONE',  ( -13.85723511636018301, 4.102873376188801657, 5.986996695041598926 ) ) ;
#2763=CARTESIAN_POINT ( 'NONE',  ( -13.18405858231679595, -20.26807450282662160, 1.696391591240633101 ) ) ;
#2764=CARTESIAN_POINT ( 'NONE',  ( -1.126276606324276619, -9.114917468222230923, 1.622643865078341463 ) ) ;
#2766=CARTESIAN_POINT ( 'NONE',  ( -13.39107665282975645, -19.43812903209671461, 5.476542851584349947 ) ) ;
#2768=CARTESIAN_POINT ( 'NONE',  ( 6.715308582316796837, -24.52099543870834708, 2.515153566944913432 ) ) ;
#2769=CARTESIAN_POINT ( 'NONE',  ( -3.974842109207561425, -21.82955800590261575, 5.256404853634145447 ) ) ;
#2771=CARTESIAN_POINT ( 'NONE',  ( 13.50467269799730374, -14.45152875114793467, 6.346192769197517514 ) ) ;
#2772=CARTESIAN_POINT ( 'NONE',  ( 12.62499979224180180, -20.25001049178813162, 4.458178821399696012 ) ) ;
#2780=CARTESIAN_POINT ( 'NONE',  ( -13.87470602645761986, 4.985154336109792972, 4.583333333333296622 ) ) ;
#2787=CARTESIAN_POINT ( 'NONE',  ( 3.002445346198714837, -11.66215945560911749, 2.276826493710632171 ) ) ;
#2790=AXIS2_PLACEMENT_3D ( 'NONE', #2726, #15374, #10785 ) ;
#2791=EDGE_CURVE ( 'NONE', #4418, #11657, #15708, .T. ) ;
#2795=CARTESIAN_POINT ( 'NONE',  ( 5.878441417683177406, -22.99999999999999645, 3.449312527122335048 ) ) ;
#2796=CARTESIAN_POINT ( 'NONE',  ( -13.05696142222617695, 1.564051822406025583, 5.955108176248398166 ) ) ;
#2797=CARTESIAN_POINT ( 'NONE',  ( -9.621558582316795949, -22.99999999999999645, 3.550687472877652073 ) ) ;
#2798=CARTESIAN_POINT ( 'NONE',  ( -10.09719141768317741, -23.08622137881040359, 5.979004561291654696 ) ) ;
#2800=CARTESIAN_POINT ( 'NONE',  ( 13.09533517714100093, 4.251926445620864747, 5.084080158857392284 ) ) ;
#2804=ORIENTED_EDGE ( 'NONE', *, *, #20615, .F. ) ;
#2805=CARTESIAN_POINT ( 'NONE',  ( 1.882415164465650825, -10.11790622164856224, 2.437616430916333510 ) ) ;
#2809=CARTESIAN_POINT ( 'NONE',  ( -2.011668220304084542, -11.03559989230542193, 2.673298498313999794 ) ) ;
#2814=CARTESIAN_POINT ( 'NONE',  ( 8.878441417683177406, -24.50000000000000000, 3.449312527122335048 ) ) ;
#2816=CARTESIAN_POINT ( 'NONE',  ( -10.19094141768317563, -23.27327832286946219, 4.701595411283453707 ) ) ;
#2819=CARTESIAN_POINT ( 'NONE',  ( 5.684058582316794173, -20.79840458871652942, 2.226721677130544030 ) ) ;
#2821=CARTESIAN_POINT ( 'NONE',  ( -13.41175265982446696, -19.14399067886409256, 6.245281310864100988 ) ) ;
#2823=CARTESIAN_POINT ( 'NONE',  ( 9.621558582316794173, -23.74999999999999645, 3.550687472877651629 ) ) ;
#2827=CARTESIAN_POINT ( 'NONE',  ( 13.37500000000002132, -20.99999999999450395, 3.833333333368183382 ) ) ;
#2833=CARTESIAN_POINT ( 'NONE',  ( -10.55905858231679595, -20.72672167713054137, 4.701595411283463477 ) ) ;
#2836=CARTESIAN_POINT ( 'NONE',  ( 2.747777887823422471, -9.906471667804277459, 1.825930796414880763 ) ) ;
#2838=CARTESIAN_POINT ( 'NONE',  ( -13.09559422631463654, 4.265008428887424152, 5.017082219073495608 ) ) ;
#2839=CARTESIAN_POINT ( 'NONE',  ( -13.40432071140796744, -19.51930407389869515, 6.223619713037471968 ) ) ;
#2842=CARTESIAN_POINT ( 'NONE',  ( 5.965308582316795949, -20.97900456129165647, 3.863526089495444626 ) ) ;
#2844=CARTESIAN_POINT ( 'NONE',  ( 5.597191417683179182, -22.77556120703057729, 5.229004561291655584 ) ) ;
#2845=CARTESIAN_POINT ( 'NONE',  ( -10.47219141768317741, -23.72900456129164937, 2.724438792969417378 ) ) ;
#2848=CARTESIAN_POINT ( 'NONE',  ( 13.37500000000002132, -19.50000000000273559, 4.083333333315724012 ) ) ;
#2850=CARTESIAN_POINT ( 'NONE',  ( -1.720709671993384093, -9.114925383610804843, 1.622645897908254753 ) ) ;
#2854=CARTESIAN_POINT ( 'NONE',  ( -12.62599079447150885, -20.19996487918709249, 4.820256282269618886 ) ) ;
#2856=CARTESIAN_POINT ( 'NONE',  ( -13.87444723674697755, 4.972085455720938185, 5.163895512850782410 ) ) ;
#2857=DIRECTION ( 'NONE',  ( -1.000000000000000000, -0.000000000000000000, -0.000000000000000000 ) ) ;
#2863=CARTESIAN_POINT ( 'NONE',  ( -10.27780858231679595, -19.52099543870833642, 2.413778621189609286 ) ) ;
#2864=CARTESIAN_POINT ( 'NONE',  ( -2.808565762442263303, -10.28561894962424716, 1.923303392614186924 ) ) ;
#2866=CARTESIAN_POINT ( 'NONE',  ( -13.83770801678722329, 3.866754847752558621, 5.240062463382368030 ) ) ;
#2868=CARTESIAN_POINT ( 'NONE',  ( 11.31594141768317741, -20.26807450282663225, 5.303608408759377113 ) ) ;
#2869=CARTESIAN_POINT ( 'NONE',  ( -6.628441417683177406, -20.99999999999999645, 3.550687472877664952 ) ) ;
#2871=CARTESIAN_POINT ( 'NONE',  ( 13.87470602645761986, 4.985154336109792972, 3.000000000000000000 ) ) ;
#2873=ORIENTED_EDGE ( 'NONE', *, *, #6043, .T. ) ;
#2877=CARTESIAN_POINT ( 'NONE',  ( -13.43259567872942917, -17.34141822415733714, 5.534013032956523581 ) ) ;
#2882=CARTESIAN_POINT ( 'NONE',  ( 2.702705060698113115, -10.69015907548275379, 2.777197378435510622 ) ) ;
#2884=CARTESIAN_POINT ( 'NONE',  ( 3.347120161770001268, -14.10934257735911146, 2.905312006771028077 ) ) ;
#2886=CARTESIAN_POINT ( 'NONE',  ( 13.12512971825177033, 5.006550771716304915, 5.133277049491872468 ) ) ;
#2892=CARTESIAN_POINT ( 'NONE',  ( 8.690941417683177406, -22.74294823697955081, 4.171265325393542334 ) ) ;
#2893=CARTESIAN_POINT ( 'NONE',  ( -12.64931222250080545, -19.02223276370786209, 5.512399842915133519 ) ) ;
#2894=CARTESIAN_POINT ( 'NONE',  ( -11.49655858231679595, -22.05068747287764452, 2.499999999999999112 ) ) ;
#2895=CARTESIAN_POINT ( 'NONE',  ( -12.06594141768317563, -23.20159541128344927, 2.226721677130534705 ) ) ;
#2898=CARTESIAN_POINT ( 'NONE',  ( 13.37593719518949698, -19.45267164293252193, 4.647380496992003174 ) ) ;
#2903=CARTESIAN_POINT ( 'NONE',  ( 1.797604806073912709, -9.120796646272857799, 2.374153755450133740 ) ) ;
#2910=CARTESIAN_POINT ( 'NONE',  ( -1.882415164465650825, -10.11790622164856224, 2.437616430916333510 ) ) ;
#2914=CARTESIAN_POINT ( 'NONE',  ( 4.659691417683177406, -22.98484643305507191, 0.9790045612916508100 ) ) ;
#2916=CARTESIAN_POINT ( 'NONE',  ( -10.75344141768317741, -21.94931252712233061, 1.749999999999998446 ) ) ;
#2918=CARTESIAN_POINT ( 'NONE',  ( 6.902808582316793284, -22.77556120703056308, 1.770995438708339975 ) ) ;
#2920=CARTESIAN_POINT ( 'NONE',  ( -12.65346245025441263, -19.56264626215117275, 6.228892365149262922 ) ) ;
#2922=CARTESIAN_POINT ( 'NONE',  ( 7.559058582316794173, -20.72672167713054137, 4.701595411283463477 ) ) ;
#2925=CARTESIAN_POINT ( 'NONE',  ( 13.85956729540471066, 3.470648417939721231, 6.731609435864099211 ) ) ;
#2931=CARTESIAN_POINT ( 'NONE',  ( -9.809058582316794173, -23.27327832286945153, 2.298404588716537411 ) ) ;
#2932=CARTESIAN_POINT ( 'NONE',  ( 13.87406079471522347, 4.952570133121557028, 5.260711232101737522 ) ) ;
#2934=CARTESIAN_POINT ( 'NONE',  ( 3.521144778809589315, -10.09312707791070096, 2.066482617302010105 ) ) ;
#2936=CARTESIAN_POINT ( 'NONE',  ( -13.37893135632597819, -19.30146650553847465, 4.738802066438188909 ) ) ;
#2937=CARTESIAN_POINT ( 'NONE',  ( 9.059058582316794173, -20.72672167713054137, 4.701595411283463477 ) ) ;
#2938=CARTESIAN_POINT ( 'NONE',  ( -13.90439735423812273, 5.734566389025032684, 3.666666666666500873 ) ) ;
#2940=CARTESIAN_POINT ( 'NONE',  ( 9.527808582316792396, -23.72900456129165647, 4.275561207030568411 ) ) ;
#2941=CARTESIAN_POINT ( 'NONE',  ( 6.628441417683177406, -20.99999999999999645, 3.550687472877664952 ) ) ;
#2942=CARTESIAN_POINT ( 'NONE',  ( -7.184058582316794173, -20.79840458871652942, 2.226721677130544030 ) ) ;
#2945=CARTESIAN_POINT ( 'NONE',  ( 13.09560264576187905, 4.265433610975056133, 4.583333333333295734 ) ) ;
#2951=EDGE_CURVE ( 'NONE', #13563, #8562, #3701, .T. ) ;
#2952=CARTESIAN_POINT ( 'NONE',  ( -12.63465172146706728, -19.76258806590802664, 5.372658420469845986 ) ) ;
#2954=CARTESIAN_POINT ( 'NONE',  ( -3.302240162463773832, -9.695145533921818881, 2.714273006325518711 ) ) ;
#2955=CARTESIAN_POINT ( 'NONE',  ( -13.85223456079946303, 3.850345320370711644, 5.989742199623227847 ) ) ;
#2963=CARTESIAN_POINT ( 'NONE',  ( 12.62499999999998224, -20.25000000000006395, 4.416666666666681174 ) ) ;
#2965=CARTESIAN_POINT ( 'NONE',  ( -6.059058582316795949, -20.19639159124062999, 5.231925497173373074 ) ) ;
#2966=CARTESIAN_POINT ( 'NONE',  ( -0.2815691515810352374, -9.864917468222230923, 1.622643865078524428 ) ) ;
#2968=CARTESIAN_POINT ( 'NONE',  ( -13.37499999999998401, -20.24999999999998934, 2.439580858552613751 ) ) ;
#2970=CARTESIAN_POINT ( 'NONE',  ( 5.496558582316795949, -22.05068747287764452, 0.9999999999999978906 ) ) ;
#2971=CARTESIAN_POINT ( 'NONE',  ( -4.378441417683176518, -22.99999999999999645, 3.449312527122335048 ) ) ;
#2973=CARTESIAN_POINT ( 'NONE',  ( 13.41475008041063433, -18.99262093926051520, 6.248536519197435801 ) ) ;
#2984=CARTESIAN_POINT ( 'NONE',  ( 0.5631383031621635116, -9.114917468222230923, 2.372643865078341019 ) ) ;
#2987=CARTESIAN_POINT ( 'NONE',  ( 2.616536356806028696, -10.07836329504444706, 2.620076000170431296 ) ) ;
#2990=CARTESIAN_POINT ( 'NONE',  ( 1.337453470010121714, -8.364917468222230923, 1.622643865078341907 ) ) ;
#2997=CARTESIAN_POINT ( 'NONE',  ( 4.753441417683176518, -21.94931252712233061, 2.499999999999999112 ) ) ;
#2998=CARTESIAN_POINT ( 'NONE',  ( -13.08573665985359824, 3.017201322601628100, 5.986358176248492313 ) ) ;
#3000=CARTESIAN_POINT ( 'NONE',  ( -10.37155858231679595, -20.99999999999999645, 3.449312527122348371 ) ) ;
#3001=CARTESIAN_POINT ( 'NONE',  ( -12.62844141768317741, -20.24999999999999289, 3.550687472877664952 ) ) ;
#3003=CARTESIAN_POINT ( 'NONE',  ( 13.09494140422671471, 4.232040913449062636, 5.131376921800749003 ) ) ;
#3006=CARTESIAN_POINT ( 'NONE',  ( 2.601332995093193379, -9.970398767539743190, 2.592349323443654097 ) ) ;
#3008=CARTESIAN_POINT ( 'NONE',  ( 2.702705060698113115, -10.69015907548275379, 2.777197378435510622 ) ) ;
#3014=CARTESIAN_POINT ( 'NONE',  ( 8.128441417683175629, -20.24999999999999289, 3.550687472877664952 ) ) ;
#3017=CARTESIAN_POINT ( 'NONE',  ( -1.865667289525601680, -9.999006358835732300, 2.407080570882605297 ) ) ;
#3022=CARTESIAN_POINT ( 'NONE',  ( 9.253441417683177406, -21.94931252712233061, 0.9999999999999978906 ) ) ;
#3024=CARTESIAN_POINT ( 'NONE',  ( -10.84719141768317563, -21.22443879296941915, 1.770995438708345748 ) ) ;
#3026=CARTESIAN_POINT ( 'NONE',  ( 9.809058582316794173, -23.27327832286945153, 2.298404588716537411 ) ) ;
#3028=CARTESIAN_POINT ( 'NONE',  ( -13.90439706815434739, 5.734551941788608609, 5.045486763335835789 ) ) ;
#3031=CARTESIAN_POINT ( 'NONE',  ( 6.434058582316794173, -23.20159541128345992, 4.773278322869455970 ) ) ;
#3036=B_SPLINE_CURVE_WITH_KNOTS ( 'NONE', 3,
 ( #1834, #9477, #15746, #13019, #4968, #164, #20675, #1428, #6547, #4865 ),
 .UNSPECIFIED., .F., .F.,
 ( 4, 2, 2, 2, 4 ),
 ( 0.000000000000000000, 0.0002944886444448786226, 0.0005889772888897572452, 0.0008834659333346358678, 0.001177954577779514490 ),
 .UNSPECIFIED. ) ;
#3040=CARTESIAN_POINT ( 'NONE',  ( -8.684058582316794173, -20.79840458871652942, 2.226721677130544030 ) ) ;
#3041=CARTESIAN_POINT ( 'NONE',  ( 12.62499999999998224, -20.24999999999991829, 4.333333333333343695 ) ) ;
#3042=( GEOMETRIC_REPRESENTATION_CONTEXT ( 3 ) GLOBAL_UNCERTAINTY_ASSIGNED_CONTEXT ( ( #2326 ) ) GLOBAL_UNIT_ASSIGNED_CONTEXT ( ( #12848, #16301, #17560 ) ) REPRESENTATION_CONTEXT ( 'NONE', 'WORKASPACE' ) );
#3045=CARTESIAN_POINT ( 'NONE',  ( 0.9854920305337622199, -9.864917468222230923, 1.622643865078341907 ) ) ;
#3050=CARTESIAN_POINT ( 'NONE',  ( -13.84051394328565365, 4.008454135954084840, 5.243107695145536873 ) ) ;
#3051=CARTESIAN_POINT ( 'NONE',  ( 5.121558582316794173, -23.74999999999999645, 3.550687472877651629 ) ) ;
#3052=CARTESIAN_POINT ( 'NONE',  ( -12.62499999999998401, -20.99999999999999645, 3.146526952850934755 ) ) ;
#3056=CARTESIAN_POINT ( 'NONE',  ( 4.659691417683177406, -22.36352608949543352, 2.479004561291652031 ) ) ;
#3057=CARTESIAN_POINT ( 'NONE',  ( -7.371558582316794173, -20.24999999999999289, 3.449312527122348371 ) ) ;
#3059=CARTESIAN_POINT ( 'NONE',  ( 13.37930517931174634, -19.28258844475809042, 4.742233558278135419 ) ) ;
#3060=CARTESIAN_POINT ( 'NONE',  ( -1.652577328807104839, -9.114908150887895744, 1.622641472200749835 ) ) ;
#3066=CARTESIAN_POINT ( 'NONE',  ( -1.787053415088318609, -8.367039355952382351, 2.373188808236395886 ) ) ;
#3070=CARTESIAN_POINT ( 'NONE',  ( 10.37155858231679417, -20.24999999999999289, 3.449312527122348371 ) ) ;
#3072=CARTESIAN_POINT ( 'NONE',  ( 12.68302225826488616, -18.06987595762608478, 6.282912912489355683 ) ) ;
#3074=CARTESIAN_POINT ( 'NONE',  ( -4.717959273841179524, -21.63341328858655999, 5.993595146365859883 ) ) ;
#3075=CARTESIAN_POINT ( 'NONE',  ( -1.710927537542899612, -9.866086492083725901, 2.372944093759576933 ) ) ;
#3077=CARTESIAN_POINT ( 'NONE',  ( -13.84439157666246878, 4.204274621457510186, 5.123803251657143676 ) ) ;
#3080=CARTESIAN_POINT ( 'NONE',  ( 3.944195004867014909, -21.42722504787766624, 5.934029185143018914 ) ) ;
#3081=CARTESIAN_POINT ( 'NONE',  ( -11.40280858231679595, -22.46490103525074034, 2.520995438708341307 ) ) ;
#3083=CARTESIAN_POINT ( 'NONE',  ( 13.87444723674697755, 4.972085455720938185, 5.163895512850782410 ) ) ;
#3084=CARTESIAN_POINT ( 'NONE',  ( 12.63819864697926754, -19.58346832754827105, 5.450273968536036406 ) ) ;
#3095=CARTESIAN_POINT ( 'NONE',  ( 1.513434189748285918, -8.364917468222230923, 1.622643865078341907 ) ) ;
#3101=CARTESIAN_POINT ( 'NONE',  ( 6.065941417683177406, -22.67126532539353789, 2.757051763020445634 ) ) ;
#3102=CARTESIAN_POINT ( 'NONE',  ( -13.10557919622060652, 4.019249409169220577, 6.007898877577752650 ) ) ;
#3103=CARTESIAN_POINT ( 'NONE',  ( -9.996558582316795949, -22.05068747287764452, 2.499999999999999112 ) ) ;
#3106=CARTESIAN_POINT ( 'NONE',  ( -10.47219141768317563, -23.72900456129165292, 2.724438792969417822 ) ) ;
#3108=CARTESIAN_POINT ( 'NONE',  ( 13.09206359972826661, 4.086711786274932479, 5.245812454509717782 ) ) ;
#3117=CARTESIAN_POINT ( 'NONE',  ( 8.972191417683177406, -23.72900456129164937, 2.724438792969417378 ) ) ;
#3120=CARTESIAN_POINT ( 'NONE',  ( -2.436080212393455735, -9.483920418190111334, 2.467411194204634839 ) ) ;
#3124=CARTESIAN_POINT ( 'NONE',  ( 7.378441417683177406, -24.50000000000000000, 3.449312527122335048 ) ) ;
#3126=CARTESIAN_POINT ( 'NONE',  ( -8.503441417683177406, -22.05068747287765873, 5.250000000000000888 ) ) ;
#3129=CARTESIAN_POINT ( 'NONE',  ( 5.496558582316794173, -22.05068747287764452, 1.749999999999998446 ) ) ;
#3130=CARTESIAN_POINT ( 'NONE',  ( -13.90326467458556969, 5.677366066573198644, 5.457668599364335904 ) ) ;
#3132=CARTESIAN_POINT ( 'NONE',  ( 4.717959273841178636, -21.72818306014730183, 5.243595146365860771 ) ) ;
#3136=SURFACE_STYLE_FILL_AREA ( #11087 ) ;
#3141=CARTESIAN_POINT ( 'NONE',  ( -5.777808582316794173, -20.27099543870833642, 2.724438792969431589 ) ) ;
#3142=CARTESIAN_POINT ( 'NONE',  ( 12.62599079447150885, -20.19996487918709249, 4.820256282269618886 ) ) ;
#3145=CARTESIAN_POINT ( 'NONE',  ( 0.000000000000000000, -9.864917468222230923, 1.622643865078341241 ) ) ;
#3147=CARTESIAN_POINT ( 'NONE',  ( -13.84501469867365131, 4.235742283194553259, 3.333333333332063386 ) ) ;
#3148=CARTESIAN_POINT ( 'NONE',  ( 9.527808582316792396, -23.72900456129165647, 4.275561207030568411 ) ) ;
#3149=CARTESIAN_POINT ( 'NONE',  ( -12.62500000000002132, -21.00000000000274269, 4.083333333315724012 ) ) ;
#3153=CARTESIAN_POINT ( 'NONE',  ( -5.965308582316795949, -19.47900456129164937, 4.484846433055089676 ) ) ;
#3155=CARTESIAN_POINT ( 'NONE',  ( 5.784691417683178294, -23.02099543870834353, 3.863526089495429972 ) ) ;
#3156=CARTESIAN_POINT ( 'NONE',  ( -4.687312169500632564, -21.51559725698341197, 5.182386163300427562 ) ) ;
#3158=CARTESIAN_POINT ( 'NONE',  ( 13.84311479963346869, 4.139797381492562600, 5.195993353439945395 ) ) ;
#3161=PRODUCT_DEFINITION_CONTEXT ( 'detailed design', #17226, 'design' ) ;
#3166=CARTESIAN_POINT ( 'NONE',  ( -13.12529397354238192, 5.014845663890295846, 4.333333333333374782 ) ) ;
#3167=CARTESIAN_POINT ( 'NONE',  ( -1.407845757905374695, -8.364917468222230923, 2.372643865078341019 ) ) ;
#3169=CARTESIAN_POINT ( 'NONE',  ( 2.786182376113650605, -10.12667130264514626, 1.882483419865550900 ) ) ;
#3170=CARTESIAN_POINT ( 'NONE',  ( -12.72125031657057015, -15.38935901321805133, 5.590524842915047365 ) ) ;
#3171=CARTESIAN_POINT ( 'NONE',  ( 13.37327929115833669, -20.24999999707183207, 3.449077790995325632 ) ) ;
#3173=CARTESIAN_POINT ( 'NONE',  ( 12.67103257592000176, -18.67535491604046172, 6.269892079155907183 ) ) ;
#3174=CARTESIAN_POINT ( 'NONE',  ( -1.925499516411631973, -10.42380411186744382, 2.516177120048874283 ) ) ;
#3176=CARTESIAN_POINT ( 'NONE',  ( -13.37499999999998401, -20.99999999999998934, 2.439580858552613751 ) ) ;
#3178=CARTESIAN_POINT ( 'NONE',  ( 7.378441417683177406, -24.50000000000000000, 3.449312527122335048 ) ) ;
#3179=CARTESIAN_POINT ( 'NONE',  ( -12.52780858231679773, -22.97900456129165647, 3.964901035250747885 ) ) ;
#3181=CARTESIAN_POINT ( 'NONE',  ( 13.43273460392801155, -18.08440250163749496, 6.268067769197452677 ) ) ;
#3194=CARTESIAN_POINT ( 'NONE',  ( 1.619022621591186928, -9.864917468222230923, 1.622643865078341907 ) ) ;
#3199=CARTESIAN_POINT ( 'NONE',  ( -11.77780858231679417, -20.27099543870833642, 2.724438792969431589 ) ) ;
#3200=CARTESIAN_POINT ( 'NONE',  ( -2.583953725994688533, -9.847075946378776479, 2.560676788604062004 ) ) ;
#3201=VECTOR ( 'NONE', #20273, 1000.000000000000000 ) ;
#3202=CARTESIAN_POINT ( 'NONE',  ( 6.628441417683177406, -20.99999999999999645, 3.550687472877664952 ) ) ;
#3203=CARTESIAN_POINT ( 'NONE',  ( -13.12529397353891270, 5.014845663890295846, 3.333333333333220239 ) ) ;
#3204=CARTESIAN_POINT ( 'NONE',  ( -11.49655858231679417, -22.05068747287764452, 1.749999999999998446 ) ) ;
#3205=CARTESIAN_POINT ( 'NONE',  ( -6.347191417683176518, -20.91377862118959285, 1.020995438708345082 ) ) ;
#3207=CARTESIAN_POINT ( 'NONE',  ( 13.09553549038190567, 4.262042264285192950, 5.042530537310905281 ) ) ;
#3217=CARTESIAN_POINT ( 'NONE',  ( -1.791727654783324741, -9.894249715907907472, 2.380176972254574697 ) ) ;
#3219=CARTESIAN_POINT ( 'NONE',  ( -12.34030858231679240, -22.67418626127525982, 5.270995438708342640 ) ) ;
#3223=CARTESIAN_POINT ( 'NONE',  ( 7.847191417683175629, -20.91377862118959285, 1.020995438708345082 ) ) ;
#3224=CARTESIAN_POINT ( 'NONE',  ( -12.34719141768317741, -21.53509896474923835, 2.520995438708346192 ) ) ;
#3226=CARTESIAN_POINT ( 'NONE',  ( 5.309058582316794173, -23.27327832286945153, 2.298404588716537411 ) ) ;
#3228=CARTESIAN_POINT ( 'NONE',  ( -12.65816212372154403, -19.32531275206247301, 6.255900543948403225 ) ) ;
#3230=CARTESIAN_POINT ( 'NONE',  ( 8.590308582316794173, -21.32581373872472597, 1.729004561291657582 ) ) ;
#3237=CARTESIAN_POINT ( 'NONE',  ( -5.121558582316794173, -23.74999999999999645, 3.550687472877651629 ) ) ;
#3238=CARTESIAN_POINT ( 'NONE',  ( 12.62499999999999289, -20.24999999999899103, 3.700614806296627979 ) ) ;
#3241=CARTESIAN_POINT ( 'NONE',  ( 1.548630333695928618, -9.864917468222230923, 1.622643865078341907 ) ) ;
#3243=CARTESIAN_POINT ( 'NONE',  ( -13.84501469867711698, 4.235742283194553259, 4.666666666666618113 ) ) ;
#3244=CARTESIAN_POINT ( 'NONE',  ( 6.621558582316794173, -23.74999999999999645, 3.550687472877651629 ) ) ;
#3245=CARTESIAN_POINT ( 'NONE',  ( -13.90439735423812273, 5.734566389025032684, 4.333333333333380999 ) ) ;
#3247=CARTESIAN_POINT ( 'NONE',  ( -8.121558582316795949, -24.50000000000000000, 3.550687472877651629 ) ) ;
#3248=CARTESIAN_POINT ( 'NONE',  ( 9.059058582316794173, -20.72672167713054137, 4.701595411283463477 ) ) ;
#3251=CARTESIAN_POINT ( 'NONE',  ( 7.940941417683175629, -21.25705176302044208, 2.828734674606458555 ) ) ;
#3252=CARTESIAN_POINT ( 'NONE',  ( -9.159691417683177406, -22.67418626127524917, 1.729004561291651587 ) ) ;
#3254=CARTESIAN_POINT ( 'NONE',  ( 13.84501469867711698, 4.235742283194553259, 2.999999999999999556 ) ) ;
#3264=CARTESIAN_POINT ( 'NONE',  ( -1.126276606324276619, -9.114917468222230923, 2.372643865078341019 ) ) ;
#3267=CARTESIAN_POINT ( 'NONE',  ( -13.11514659413808737, 4.502403003978772134, 5.887634658581065494 ) ) ;
#3270=CARTESIAN_POINT ( 'NONE',  ( 13.15498530132288479, 5.764257716805535559, 2.999999999999999556 ) ) ;
#3271=CARTESIAN_POINT ( 'NONE',  ( -1.665360951492234287, -9.864914341757378580, 1.622643062139706993 ) ) ;
#3273=CARTESIAN_POINT ( 'NONE',  ( -13.87470602645761986, 4.985154336109792972, 4.791666666666685614 ) ) ;
#3275=CARTESIAN_POINT ( 'NONE',  ( 4.659691417683177406, -22.98484643305507191, 0.9790045612916508100 ) ) ;
#3276=CARTESIAN_POINT ( 'NONE',  ( -4.840308582316795061, -22.36352608949544418, 4.520995438708343528 ) ) ;
#3278=CARTESIAN_POINT ( 'NONE',  ( 13.71569110726703045, -3.795099083046435506, 6.575359435862661250 ) ) ;
#3279=CARTESIAN_POINT ( 'NONE',  ( 13.10624331898488037, 4.052787608736739600, 6.006964772046813117 ) ) ;
#3288=CARTESIAN_POINT ( 'NONE',  ( 2.124709647372160060, -10.68204274815009924, 1.832497960681391147 ) ) ;
#3293=CARTESIAN_POINT ( 'NONE',  ( -12.43405858231679417, -23.20159541128345992, 4.773278322869455970 ) ) ;
#3294=CARTESIAN_POINT ( 'NONE',  ( -2.203959450683124377, -9.262433282444222371, 2.410528873095051594 ) ) ;
#3297=CARTESIAN_POINT ( 'NONE',  ( 9.434058582316795949, -22.67126532539354855, 4.242948236979545484 ) ) ;
#3298=CARTESIAN_POINT ( 'NONE',  ( -13.07121011584135672, 3.033610849983475521, 5.236678440007632496 ) ) ;
#3299=CARTESIAN_POINT ( 'NONE',  ( -11.68405858231679417, -20.79840458871652942, 2.226721677130544030 ) ) ;
#3301=CARTESIAN_POINT ( 'NONE',  ( -12.34719141768317563, -21.22443879296941915, 1.770995438708345748 ) ) ;
#3304=CARTESIAN_POINT ( 'NONE',  ( 13.83770801678722329, 3.866754847752558621, 5.240062463382368030 ) ) ;
#3313=ORIENTED_EDGE ( 'NONE', *, *, #19126, .T. ) ;
#3314=CARTESIAN_POINT ( 'NONE',  ( 10.28469141768317741, -23.77099543870834353, 4.174186261275251830 ) ) ;
#3317=CARTESIAN_POINT ( 'NONE',  ( -1.126276606324276619, -9.114917468222230923, 2.372643865078341019 ) ) ;
#3318=CARTESIAN_POINT ( 'NONE',  ( 2.616536356806028696, -10.07836329504444706, 2.620076000170431296 ) ) ;
#3319=CARTESIAN_POINT ( 'NONE',  ( -13.09030858231679417, -21.32581373872472952, 1.729004561291657138 ) ) ;
#3321=CARTESIAN_POINT ( 'NONE',  ( 7.003441417683177406, -22.05068747287765873, 5.250000000000000888 ) ) ;
#3323=CARTESIAN_POINT ( 'NONE',  ( -11.03469141768317741, -20.97900456129164581, 3.136473910504570917 ) ) ;
#3325=CARTESIAN_POINT ( 'NONE',  ( 7.934058582316796837, -23.73192549717337130, 5.303608408759367343 ) ) ;
#3327=CARTESIAN_POINT ( 'NONE',  ( -12.62543384439201510, -20.97809085820452424, 4.782403934559678937 ) ) ;
#3330=CARTESIAN_POINT ( 'NONE',  ( 5.684058582316794173, -20.79840458871652942, 2.226721677130544030 ) ) ;
#3337=AXIS2_PLACEMENT_3D ( 'NONE', #15356, #16825, #2489 ) ;
#3342=CARTESIAN_POINT ( 'NONE',  ( -5.215308582316793284, -23.77099543870833998, 2.825813738724734847 ) ) ;
#3343=CARTESIAN_POINT ( 'NONE',  ( 12.62672070884157804, -20.24999999999983658, 3.550922209436377042 ) ) ;
#3346=CARTESIAN_POINT ( 'NONE',  ( 0.9854920305337621089, -9.114917468222230923, 1.622643865078341463 ) ) ;
#3347=CARTESIAN_POINT ( 'NONE',  ( 12.64751377014909828, -19.11305460747000495, 5.510446717915143289 ) ) ;
#3349=CARTESIAN_POINT ( 'NONE',  ( -13.82092246150448211, 3.019084305971233562, 5.221833296715730377 ) ) ;
#3350=CARTESIAN_POINT ( 'NONE',  ( 11.49655858231679595, -22.05068747287764452, 0.9999999999999978906 ) ) ;
#3351=CARTESIAN_POINT ( 'NONE',  ( -13.90439735423812273, 5.734566389025032684, 2.999999999999999556 ) ) ;
#3354=CARTESIAN_POINT ( 'NONE',  ( 6.434058582316794173, -23.20159541128345992, 4.773278322869455970 ) ) ;
#3356=CARTESIAN_POINT ( 'NONE',  ( 7.190941417683177406, -22.74294823697955081, 4.171265325393542334 ) ) ;
#3357=CARTESIAN_POINT ( 'NONE',  ( -8.409691417683177406, -21.32581373872474373, 5.270995438708348857 ) ) ;
#3360=CARTESIAN_POINT ( 'NONE',  ( 13.84485691484488257, 4.227774199669918964, 5.063753864839139140 ) ) ;
#3370=CARTESIAN_POINT ( 'NONE',  ( -13.12424783836753228, 4.962015837561366993, 5.328858059679200565 ) ) ;
#3371=CARTESIAN_POINT ( 'NONE',  ( -3.451187703687236041, -10.75258211228477734, 2.985843844067104680 ) ) ;
#3374=CARTESIAN_POINT ( 'NONE',  ( -12.64131715375063258, -19.42598373559290792, 5.491151580003103660 ) ) ;
#3375=CARTESIAN_POINT ( 'NONE',  ( 12.05905858231679417, -20.72672167713054137, 4.701595411283463477 ) ) ;
#3377=CARTESIAN_POINT ( 'NONE',  ( 12.69740987707854707, -17.34330120752609616, 6.298537912489285517 ) ) ;
#3378=CARTESIAN_POINT ( 'NONE',  ( -2.022757268986824730, -10.07035769906783784, 1.675405020440470238 ) ) ;
#3380=CARTESIAN_POINT ( 'NONE',  ( -13.85403523778986390, 3.941279508358651817, 5.991705257707216958 ) ) ;
#3384=CARTESIAN_POINT ( 'NONE',  ( 3.974842109207560537, -21.73478823434188456, 6.006404853634143670 ) ) ;
#3385=CARTESIAN_POINT ( 'NONE',  ( -8.027808582316795949, -22.97900456129165647, 3.964901035250747885 ) ) ;
#3388=CARTESIAN_POINT ( 'NONE',  ( 13.83079205777725917, 2.017498917744843023, 6.700359435863729729 ) ) ;
#3389=CARTESIAN_POINT ( 'NONE',  ( 13.10192273101908000, 3.834597916462216816, 6.003936301248457674 ) ) ;
#3398=CARTESIAN_POINT ( 'NONE',  ( 2.110348196723525138, -10.58007678474401914, 1.806311064303893099 ) ) ;
#3403=CARTESIAN_POINT ( 'NONE',  ( -11.87155858231679417, -20.24999999999999289, 3.449312527122348371 ) ) ;
#3404=CARTESIAN_POINT ( 'NONE',  ( -0.9854920305337621089, -9.114917468222230923, 2.372643865078341019 ) ) ;
#3405=CARTESIAN_POINT ( 'NONE',  ( -13.09300823383486900, 4.134415808666423331, 5.226944302881396887 ) ) ;
#3406=CARTESIAN_POINT ( 'NONE',  ( -11.59030858231679417, -21.32581373872472597, 1.729004561291657582 ) ) ;
#3408=CARTESIAN_POINT ( 'NONE',  ( -6.534691417683176518, -20.22900456129164581, 2.825813738724747726 ) ) ;
#3411=CARTESIAN_POINT ( 'NONE',  ( 13.38929389708972195, -18.77815819697223887, 4.753083296715700179 ) ) ;
#3422=CARTESIAN_POINT ( 'NONE',  ( -2.693754455098655409, -10.04853567022903782, 2.237415670251142519 ) ) ;
#3425=CARTESIAN_POINT ( 'NONE',  ( -1.742625132518061504, -9.872369070458363538, 2.374557585393312298 ) ) ;
#3426=CARTESIAN_POINT ( 'NONE',  ( 2.559937518207947793, -9.746075135043517079, 2.534737762559237773 ) ) ;
#3427=CARTESIAN_POINT ( 'NONE',  ( -12.80905858231679417, -23.27327832286945153, 2.298404588716537411 ) ) ;
#3430=CARTESIAN_POINT ( 'NONE',  ( 7.284691417683176518, -23.77099543870834353, 4.174186261275252718 ) ) ;
#3432=CARTESIAN_POINT ( 'NONE',  ( -4.847191417683178294, -21.22443879296941915, 1.770995438708345748 ) ) ;
#3434=CARTESIAN_POINT ( 'NONE',  ( 9.152808582316795949, -20.91377862118960351, 5.979004561291660913 ) ) ;
#3435=CARTESIAN_POINT ( 'NONE',  ( 12.64195242771744709, -19.39390240027112000, 5.496549442168085164 ) ) ;
#3436=CARTESIAN_POINT ( 'NONE',  ( -13.15498566372047762, 5.764276017890828108, 4.942557026581394730 ) ) ;
#3443=CARTESIAN_POINT ( 'NONE',  ( 12.73791931723291881, -19.98176637867805283, 3.535752669880253940 ) ) ;
#3445=CARTESIAN_POINT ( 'NONE',  ( -7.465308582316795061, -20.22900456129164937, 4.174186261275266929 ) ) ;
#3447=CARTESIAN_POINT ( 'NONE',  ( 12.64931222250080545, -19.02223276370786209, 5.512399842915133519 ) ) ;
#3450=CARTESIAN_POINT ( 'NONE',  ( 12.62599079447150885, -20.19996487918709249, 4.820256282269618886 ) ) ;
#3452=CARTESIAN_POINT ( 'NONE',  ( -13.37499999999998579, -20.24999999999999289, 3.666666666666653640 ) ) ;
#3453=CARTESIAN_POINT ( 'NONE',  ( 11.68405858231679595, -20.26807450282662160, 1.696391591240633101 ) ) ;
#3454=CARTESIAN_POINT ( 'NONE',  ( -13.15452713448031297, 5.741120291255121799, 5.290164123766007087 ) ) ;
#3455=CARTESIAN_POINT ( 'NONE',  ( -11.22219141768317741, -19.52099543870834353, 4.586221378810406257 ) ) ;
#3458=CARTESIAN_POINT ( 'NONE',  ( 12.43405858231679595, -22.67126532539354855, 4.242948236979545484 ) ) ;
#3459=CARTESIAN_POINT ( 'NONE',  ( -8.034691417683175629, -20.22900456129164581, 2.825813738724748170 ) ) ;
#3462=CARTESIAN_POINT ( 'NONE',  ( 13.84090061271218985, 4.027980941966571748, 5.240332426532912535 ) ) ;
#3470=CARTESIAN_POINT ( 'NONE',  ( -13.12529397354238192, 5.014845663890295846, 4.916666666666650087 ) ) ;
#3475=CARTESIAN_POINT ( 'NONE',  ( -13.12503131243110843, 5.001581277770153378, 5.166347330538456184 ) ) ;
#3476=CARTESIAN_POINT ( 'NONE',  ( 7.652808582316794173, -21.22443879296942626, 5.229004561291660025 ) ) ;
#3478=CARTESIAN_POINT ( 'NONE',  ( 13.09293046926041626, 3.380488697651010011, 5.994170676248444352 ) ) ;
#3483=CARTESIAN_POINT ( 'NONE',  ( -13.43259567872942917, -17.34141822415733714, 5.534013032956523581 ) ) ;
#3485=CARTESIAN_POINT ( 'NONE',  ( 5.503441417683177406, -22.05068747287766229, 6.000000000000001776 ) ) ;
#3486=CARTESIAN_POINT ( 'NONE',  ( -5.965308582316795949, -20.97900456129165647, 3.863526089495444626 ) ) ;
#3488=CARTESIAN_POINT ( 'NONE',  ( 12.62499999998404299, -20.99999999996810729, 2.793053905886972998 ) ) ;
#3489=CARTESIAN_POINT ( 'NONE',  ( 13.10821839766814279, 4.152529082241303904, 5.997503362667785609 ) ) ;
#3490=CARTESIAN_POINT ( 'NONE',  ( -13.37499999884080637, -20.15165736766552484, 3.448843054164315802 ) ) ;
#3491=ORIENTED_EDGE ( 'NONE', *, *, #2402, .F. ) ;
#3498=CARTESIAN_POINT ( 'NONE',  ( 1.733187991654075777, -9.867296153774269385, 1.623254759047128237 ) ) ;
#3504=CARTESIAN_POINT ( 'NONE',  ( -3.475298211275419380, -9.785109117490691233, 1.987377451789144933 ) ) ;
#3506=CARTESIAN_POINT ( 'NONE',  ( -13.09494140422671471, 4.232040913449062636, 5.131376921800749003 ) ) ;
#3507=CARTESIAN_POINT ( 'NONE',  ( -5.121558582316795061, -22.99999999999999645, 3.550687472877652073 ) ) ;
#3508=CARTESIAN_POINT ( 'NONE',  ( -9.159691417683179182, -22.67418626127524917, 1.729004561291651809 ) ) ;
#3510=CARTESIAN_POINT ( 'NONE',  ( 13.84497512400090891, 4.233743762047977199, 5.032110966142367303 ) ) ;
#3517=DIRECTION ( 'NONE',  ( 1.000000000000000000, 0.000000000000000000, -0.000000000000000000 ) ) ;
#3522=CARTESIAN_POINT ( 'NONE',  ( 6.347191417683176518, -21.22443879296941915, 1.770995438708345748 ) ) ;
#3526=CARTESIAN_POINT ( 'NONE',  ( -2.567175533087980188, -9.771398394011347577, 2.541241281345096859 ) ) ;
#3531=CARTESIAN_POINT ( 'NONE',  ( 11.78469141768317563, -23.77099543870834353, 4.174186261275252718 ) ) ;
#3533=CARTESIAN_POINT ( 'NONE',  ( -4.284691417683176518, -23.77099543870834353, 4.174186261275252718 ) ) ;
#3535=CARTESIAN_POINT ( 'NONE',  ( 12.90280858231679595, -23.08622137881038938, 1.020995438708339309 ) ) ;
#3536=CARTESIAN_POINT ( 'NONE',  ( 12.69247507894198712, -16.84250851341299082, 5.559274842915185033 ) ) ;
#3537=CARTESIAN_POINT ( 'NONE',  ( -12.63465172146706728, -19.76258806590802664, 5.372658420469845986 ) ) ;
#3546=CARTESIAN_POINT ( 'NONE',  ( -7.934058582316792396, -23.20159541128345992, 4.773278322869455970 ) ) ;
#3549=CARTESIAN_POINT ( 'NONE',  ( 12.65051119073526564, -18.96168486786632457, 5.513701926248478102 ) ) ;
#3551=CARTESIAN_POINT ( 'NONE',  ( -13.37741471237955260, -20.12805702483293757, 4.993653275319895890 ) ) ;
#3552=CARTESIAN_POINT ( 'NONE',  ( 9.621558582316795949, -24.50000000000000000, 3.550687472877651629 ) ) ;
#3553=CARTESIAN_POINT ( 'NONE',  ( -12.62500000000001954, -20.25000000000274269, 4.083333333315724012 ) ) ;
#3554=CARTESIAN_POINT ( 'NONE',  ( -7.465308582316796837, -19.47900456129164937, 4.484846433055089676 ) ) ;
#3558=CARTESIAN_POINT ( 'NONE',  ( 7.840308582316795949, -22.36352608949544418, 4.520995438708343528 ) ) ;
#3559=CARTESIAN_POINT ( 'NONE',  ( -5.128441417683177406, -20.24999999999999289, 3.550687472877664952 ) ) ;
#3561=ORIENTED_EDGE ( 'NONE', *, *, #16527, .F. ) ;
#3562=CARTESIAN_POINT ( 'NONE',  ( 13.81612658856640863, 2.776892722604777930, 5.216624963382545666 ) ) ;
#3569=CARTESIAN_POINT ( 'NONE',  ( 13.83065313257865370, 2.760483195222930952, 5.966304699623404595 ) ) ;
#3573=CARTESIAN_POINT ( 'NONE',  ( -12.95145221759166354, -3.764163011652346569, 5.840524842913703552 ) ) ;
#3574=CARTESIAN_POINT ( 'NONE',  ( 5.215308582316794173, -23.77099543870833998, 2.825813738724734847 ) ) ;
#3576=CARTESIAN_POINT ( 'NONE',  ( 13.10431844137356627, 3.955581289335645234, 6.006545679920360925 ) ) ;
#3578=CARTESIAN_POINT ( 'NONE',  ( -13.66279757975024722, -5.716222222589476765, 5.784013032957989964 ) ) ;
#3580=CARTESIAN_POINT ( 'NONE',  ( 8.972191417683177406, -23.72900456129165292, 2.724438792969417822 ) ) ;
#3581=CARTESIAN_POINT ( 'NONE',  ( -8.871558582316795949, -20.99999999999999645, 3.449312527122348371 ) ) ;
#3583=CARTESIAN_POINT ( 'NONE',  ( 12.62499999999998224, -20.99999999999998934, 4.291666666666699825 ) ) ;
#3584=CARTESIAN_POINT ( 'NONE',  ( 13.12529397354238192, 5.014845663890295846, 4.166666666666765551 ) ) ;
#3596=CARTESIAN_POINT ( 'NONE',  ( 1.963707630584672570, -9.980492102769451535, 1.652325740065381909 ) ) ;
#3600=CARTESIAN_POINT ( 'NONE',  ( 12.63267999405561071, -20.34063974247287376, 3.549900554235012162 ) ) ;
#3602=CARTESIAN_POINT ( 'NONE',  ( -8.121558582316792396, -23.74999999999999645, 3.550687472877651629 ) ) ;
#3603=CARTESIAN_POINT ( 'NONE',  ( -2.076833265075072266, -8.407161531158021006, 2.383492984350220389 ) ) ;
#3605=CARTESIAN_POINT ( 'NONE',  ( -12.63478567848856571, -19.00582323632600890, 4.762720106674273701 ) ) ;
#3606=CARTESIAN_POINT ( 'NONE',  ( -6.527808582316794173, -23.72900456129165647, 4.275561207030568411 ) ) ;
#3607=CARTESIAN_POINT ( 'NONE',  ( -7.190941417683176518, -23.27327832286946219, 4.701595411283453707 ) ) ;
#3609=CARTESIAN_POINT ( 'NONE',  ( 13.38007464613909470, -19.24373036997283037, 4.743072998953621777 ) ) ;
#3618=B_SPLINE_CURVE_WITH_KNOTS ( 'NONE', 3,
 ( #878, #18458, #15410, #9237, #7473, #12265 ),
 .UNSPECIFIED., .F., .F.,
 ( 4, 2, 4 ),
 ( 0.000000000000000000, 0.5000000000000000000, 1.000000000000000000 ),
 .UNSPECIFIED. ) ;
#3624=CARTESIAN_POINT ( 'NONE',  ( -5.121558582316794173, -23.74999999999999645, 3.550687472877651629 ) ) ;
#3629=CARTESIAN_POINT ( 'NONE',  ( 9.347191417683177406, -21.22443879296941915, 1.770995438708345748 ) ) ;
#3631=CARTESIAN_POINT ( 'NONE',  ( -9.722191417683177406, -21.02099543870834353, 3.964901035250761208 ) ) ;
#3632=CARTESIAN_POINT ( 'NONE',  ( -7.465308582316796837, -19.47900456129164937, 4.484846433055089676 ) ) ;
#3634=CARTESIAN_POINT ( 'NONE',  ( 12.62499999999998224, -20.24999999999998934, 4.166666666666636765 ) ) ;
#3635=CARTESIAN_POINT ( 'NONE',  ( -12.62499999998404121, -20.24999999996810729, 2.793053905886972998 ) ) ;
#3649=CARTESIAN_POINT ( 'NONE',  ( 12.74043380832193684, -14.42059267975384529, 5.611358176248560703 ) ) ;
#3651=EDGE_CURVE ( 'NONE', #2288, #11536, #6336, .T. ) ;
#3652=CARTESIAN_POINT ( 'NONE',  ( 12.69247507894198712, -16.84250851341299082, 5.559274842915185033 ) ) ;
#3655=CARTESIAN_POINT ( 'NONE',  ( 9.996558582316795949, -22.05068747287764452, 0.9999999999999978906 ) ) ;
#3656=CARTESIAN_POINT ( 'NONE',  ( -12.62499999999998224, -20.25000000000006395, 4.416666666666681174 ) ) ;
#3657=CARTESIAN_POINT ( 'NONE',  ( -12.53469141768317741, -19.47900456129164581, 2.515153566944927199 ) ) ;
#3661=CARTESIAN_POINT ( 'NONE',  ( 11.68405858231679595, -21.32873467460644079, 2.757051763020455404 ) ) ;
#3663=CARTESIAN_POINT ( 'NONE',  ( -9.440941417683177406, -20.72672167713052715, 2.298404588716546293 ) ) ;
#3667=CARTESIAN_POINT ( 'NONE',  ( 13.85343352903393388, 3.910893216212274925, 5.991044282956552891 ) ) ;
#3674=CARTESIAN_POINT ( 'NONE',  ( 13.12500000000000533, 4.265117264764102245, 4.000000000000000888 ) ) ;
#3675=CARTESIAN_POINT ( 'NONE',  ( 13.49014615398506045, -14.43511922376608680, 5.596513032956658584 ) ) ;
#3677=CARTESIAN_POINT ( 'NONE',  ( 3.317048600639548095, -9.800042196285016161, 2.741212564741740465 ) ) ;
#3682=CARTESIAN_POINT ( 'NONE',  ( -12.62499999999998224, -19.49999999999998934, 4.166666666666637653 ) ) ;
#3683=CARTESIAN_POINT ( 'NONE',  ( 9.621558582316794173, -23.74999999999999645, 3.550687472877651629 ) ) ;
#3685=CARTESIAN_POINT ( 'NONE',  ( 12.95145221759166354, -3.764163011652346569, 5.840524842913703552 ) ) ;
#3686=CARTESIAN_POINT ( 'NONE',  ( -1.619022621591186928, -9.864917468222230923, 2.372643865078341019 ) ) ;
#3687=CARTESIAN_POINT ( 'NONE',  ( 7.746558582316795949, -21.94931252712234127, 4.499999999999999112 ) ) ;
#3689=CARTESIAN_POINT ( 'NONE',  ( 8.597191417683177406, -22.77556120703057729, 5.229004561291655584 ) ) ;
#3690=CARTESIAN_POINT ( 'NONE',  ( -6.621558582316796837, -22.99999999999999645, 3.550687472877652073 ) ) ;
#3692=CARTESIAN_POINT ( 'NONE',  ( 13.89992416064626646, 5.508670112635706495, 5.888743936161951353 ) ) ;
#3693=CARTESIAN_POINT ( 'NONE',  ( 13.12529397354238192, 5.014845663890295846, 3.000000000000000000 ) ) ;
#3701=B_SPLINE_CURVE_WITH_KNOTS ( 'NONE', 3,
 ( #11551, #14889, #3600, #5585, #7163, #6948, #14793, #14991, #3811, #13215, #5171, #17931, #13423, #7059, #19829, #13526, #5482, #9979, #16559, #18247, #11755, #3910, #16362, #13318, #2038, #6846, #19718, #10290, #15100, #472, #18146, #10189 ),
 .UNSPECIFIED., .F., .F.,
 ( 4, 2, 2, 2, 1, 2, 2, 2, 2, 2, 2, 2, 1, 2, 2, 2, 4 ),
 ( 0.000000000000000000, 0.06250846311920765785, 0.09376269467881148678, 0.1093898104586116665, 0.1172033683485095151, 0.1211101472934592721, 0.1250169262384090152, 0.1875253893575668795, 0.2500338524767247161, 0.3125423155958825805, 0.3437965471554634833, 0.3594236629352539625, 0.3672372208251511450, 0.3711439997701008187, 0.3750507787150505479, 0.4375592418342420520, 0.5000677049534336671 ),
 .UNSPECIFIED. ) ;
#3704=CARTESIAN_POINT ( 'NONE',  ( 1.655860418491166941, -9.114909740826840689, 2.372641880528837621 ) ) ;
#3711=CARTESIAN_POINT ( 'NONE',  ( -2.109407804498405703, -9.207748739546751438, 2.396484790045401603 ) ) ;
#3712=CARTESIAN_POINT ( 'NONE',  ( -10.74655858231679417, -21.94931252712234482, 5.250000000000000888 ) ) ;
#3715=CARTESIAN_POINT ( 'NONE',  ( -1.619022621591186928, -8.364917468222230923, 2.372643865078341019 ) ) ;
#3717=CARTESIAN_POINT ( 'NONE',  ( -12.99447614883396973, -0.8414544838704021146, 5.153345106674984244 ) ) ;
#3718=CARTESIAN_POINT ( 'NONE',  ( -9.621558582316794173, -23.74999999999999645, 3.550687472877651629 ) ) ;
#3719=CARTESIAN_POINT ( 'NONE',  ( -5.784691417683179182, -23.77099543870834353, 4.174186261275252718 ) ) ;
#3721=CARTESIAN_POINT ( 'NONE',  ( 13.84501469867711698, 4.235742283194553259, 4.333333333333380999 ) ) ;
#3729=CARTESIAN_POINT ( 'NONE',  ( 7.659691417683176518, -22.67418626127524917, 1.729004561291651587 ) ) ;
#3734=ADVANCED_FACE ( 'NONE', ( #16264 ), #14831, .T. ) ;
#3735=CARTESIAN_POINT ( 'NONE',  ( 13.86676110481170632, 3.833935792988865110, 6.739421935864088553 ) ) ;
#3737=CARTESIAN_POINT ( 'NONE',  ( 7.565941417683176518, -23.20159541128344927, 2.226721677130534705 ) ) ;
#3739=CARTESIAN_POINT ( 'NONE',  ( -8.972191417683177406, -22.97900456129165292, 3.035098964749240125 ) ) ;
#3741=CARTESIAN_POINT ( 'NONE',  ( -9.621558582316795949, -24.50000000000000000, 3.550687472877651629 ) ) ;
#3744=CARTESIAN_POINT ( 'NONE',  ( 13.10372118337080849, 3.925419760224517329, 6.005889426248455010 ) ) ;
#3745=CARTESIAN_POINT ( 'NONE',  ( -12.62500000000001954, -20.24999999999450040, 3.833333333368183382 ) ) ;
#3757=CARTESIAN_POINT ( 'NONE',  ( 13.10431844137356627, 3.955581289335645234, 6.006545679920360925 ) ) ;
#3758=CARTESIAN_POINT ( 'NONE',  ( -1.948765222931501784, -9.143197003266354983, 1.629906614618163552 ) ) ;
#3762=CARTESIAN_POINT ( 'NONE',  ( 12.62499999999998224, -20.24999999999991829, 4.333333333333343695 ) ) ;
#3764=CARTESIAN_POINT ( 'NONE',  ( 9.902808582316795949, -23.08622137881038938, 1.020995438708339309 ) ) ;
#3765=CARTESIAN_POINT ( 'NONE',  ( -12.62499999999998224, -20.24999999999998934, 4.291666666666698937 ) ) ;
#3766=CARTESIAN_POINT ( 'NONE',  ( -9.347191417683177406, -20.91377862118959285, 1.020995438708345082 ) ) ;
#3770=CARTESIAN_POINT ( 'NONE',  ( 10.65280858231679595, -21.53509896474924901, 4.479004561291659137 ) ) ;
#3773=EDGE_LOOP ( 'NONE', ( #763, #19842, #10079, #12431, #16955 ) ) ;
#3774=CARTESIAN_POINT ( 'NONE',  ( 13.39902456816392906, -19.03675930772010361, 5.497554699623231400 ) ) ;
#3782=CARTESIAN_POINT ( 'NONE',  ( 13.43259567872942917, -17.34141822415733714, 5.534013032956523581 ) ) ;
#3784=CARTESIAN_POINT ( 'NONE',  ( 1.126276606324276619, -8.364917468222230923, 2.372643865078341019 ) ) ;
#3789=CARTESIAN_POINT ( 'NONE',  ( -12.78345773956433895, -11.49788415197707181, 4.924178440007425550 ) ) ;
#3790=CARTESIAN_POINT ( 'NONE',  ( 5.121558582316794173, -23.74999999999999645, 3.550687472877651629 ) ) ;
#3792=CARTESIAN_POINT ( 'NONE',  ( 13.10372118337080849, 3.925419760224517329, 6.005889426248455010 ) ) ;
#3794=CARTESIAN_POINT ( 'NONE',  ( 9.902808582316795949, -22.46490103525074034, 2.520995438708341307 ) ) ;
#3795=CARTESIAN_POINT ( 'NONE',  ( 7.378441417683176518, -23.74999999999999645, 3.449312527122335492 ) ) ;
#3796=CARTESIAN_POINT ( 'NONE',  ( -8.402808582316794173, -22.77556120703056308, 1.770995438708339975 ) ) ;
#3798=CARTESIAN_POINT ( 'NONE',  ( 12.67103257592000176, -18.67535491604046172, 6.269892079155907183 ) ) ;
#3799=CARTESIAN_POINT ( 'NONE',  ( 12.62499999999998224, -19.49999999999998934, 4.166666666666637653 ) ) ;
#3805=DIRECTION ( 'NONE',  ( -1.000000000000000000, 0.000000000000000000, 0.000000000000000000 ) ) ;
#3808=CARTESIAN_POINT ( 'NONE',  ( 2.623717082130370137, -10.12934627674766830, 2.633169448359191644 ) ) ;
#3811=CARTESIAN_POINT ( 'NONE',  ( 12.71979495292231910, -20.49936819972870694, 3.538210221529994648 ) ) ;
#3813=CARTESIAN_POINT ( 'NONE',  ( -9.152808582316794173, -21.22443879296942626, 5.229004561291659137 ) ) ;
#3814=CARTESIAN_POINT ( 'NONE',  ( -3.607313482701580476, -10.70492285834919244, 2.223603995567122293 ) ) ;
#3816=CARTESIAN_POINT ( 'NONE',  ( -13.47561960997282071, -14.41870969638424071, 4.846833296715798767 ) ) ;
#3817=CARTESIAN_POINT ( 'NONE',  ( -7.746558582316794173, -21.94931252712234482, 5.250000000000000888 ) ) ;
#3818=CARTESIAN_POINT ( 'NONE',  ( -4.940941417683177406, -20.72672167713052715, 2.298404588716546293 ) ) ;
#3820=CARTESIAN_POINT ( 'NONE',  ( 13.39482594849551944, -19.24878960097397140, 5.493002502378098839 ) ) ;
#3833=CARTESIAN_POINT ( 'NONE',  ( 3.779650890485476200, -11.92851441922421607, 2.537846752097290715 ) ) ;
#3834=CARTESIAN_POINT ( 'NONE',  ( -7.746558582316794173, -21.94931252712234482, 5.250000000000000888 ) ) ;
#3835=CARTESIAN_POINT ( 'NONE',  ( 12.62500000000002132, -20.99999999999450395, 3.833333333368183382 ) ) ;
#3837=CARTESIAN_POINT ( 'NONE',  ( 9.722191417683177406, -21.02099543870834353, 3.964901035250761208 ) ) ;
#3838=CARTESIAN_POINT ( 'NONE',  ( -6.815941417683177406, -21.32873467460645145, 4.242948236979555254 ) ) ;
#3839=CARTESIAN_POINT ( 'NONE',  ( -6.059058582316795949, -20.19639159124062999, 5.231925497173373074 ) ) ;
#3841=CARTESIAN_POINT ( 'NONE',  ( 12.62499999999998579, -20.24999999999999289, 3.666666666666653640 ) ) ;
#3842=CARTESIAN_POINT ( 'NONE',  ( -12.62515553039088090, -20.24214571525854467, 4.629702272822510345 ) ) ;
#3850=CARTESIAN_POINT ( 'NONE',  ( 13.21006596862446969, -19.93552635338812706, 3.471618140591925084 ) ) ;
#3854=CARTESIAN_POINT ( 'NONE',  ( 12.83635126708105823, -9.576761012430582198, 5.715524842913705328 ) ) ;
#3856=CARTESIAN_POINT ( 'NONE',  ( -3.059891148793807414, -12.07002330923453570, 2.381574079220715401 ) ) ;
#3862=CARTESIAN_POINT ( 'NONE',  ( 6.152808582316795949, -20.91377862118960351, 5.979004561291660913 ) ) ;
#3863=CARTESIAN_POINT ( 'NONE',  ( -12.66849571425264287, -18.05346643024382303, 5.533233176248494978 ) ) ;
#3864=CARTESIAN_POINT ( 'NONE',  ( -7.565941417683177406, -23.73192549717336064, 1.696391591240623331 ) ) ;
#3866=CARTESIAN_POINT ( 'NONE',  ( 13.09030858231679417, -21.32581373872472597, 1.729004561291657582 ) ) ;
#3868=CARTESIAN_POINT ( 'NONE',  ( 11.02780858231679595, -22.97900456129165647, 3.964901035250747885 ) ) ;
#3870=ORIENTED_EDGE ( 'NONE', *, *, #15979, .T. ) ;
#3872=CARTESIAN_POINT ( 'NONE',  ( 13.40621837757088564, -18.67347193267085714, 5.505367199623145247 ) ) ;
#3880=CARTESIAN_POINT ( 'NONE',  ( 13.37524505148396514, -20.23762490005974968, 4.659512268729234741 ) ) ;
#3882=CARTESIAN_POINT ( 'NONE',  ( 2.445888733774860935, -8.532121313016713060, 2.415585152653916712 ) ) ;
#3884=CARTESIAN_POINT ( 'NONE',  ( -13.12529397354238192, 5.014845663890295846, 4.666666666666619889 ) ) ;
#3885=CARTESIAN_POINT ( 'NONE',  ( 5.965308582316793284, -20.22900456129164937, 4.174186261275266929 ) ) ;
#3887=CARTESIAN_POINT ( 'NONE',  ( 12.62562019941893432, -20.21867992933967173, 4.757612834768309540 ) ) ;
#3889=CARTESIAN_POINT ( 'NONE',  ( -2.534747216115884161, -9.671180236796224960, 2.515503256513427210 ) ) ;
#3890=CARTESIAN_POINT ( 'NONE',  ( 7.559058582316795949, -21.25705176302045274, 4.171265325393551215 ) ) ;
#3891=CARTESIAN_POINT ( 'NONE',  ( 7.003441417683177406, -22.05068747287765873, 5.250000000000000888 ) ) ;
#3892=( BOUNDED_SURFACE ( )  B_SPLINE_SURFACE ( 3, 3, ( 
 ( #9503, #499, #6680, #3841, #1864, #2168, #3634, #8151, #10016, #10124, #8457, #8552, #19450, #11487, #1764, #16395, #8246, #6879, #4998, #2073, #14824, #14514, #19646, #290, #3435, #14612, #191, #17767, #13049, #14723, #6574, #14922, #16199, #11679, #13153, #5107, #13248, #6783, #3536, #9813, #5305, #600, #16496, #17866, #19755, #5205, #9912, #16293, #1965, #18077, #8348, #6986, #401, #19550, #5415, #16095, #11583, #3744, #13355, #11788, #17963, #12939, #18179, #19343, #11377, #13770, #812, #5515, #18592, #2266, #5930, #10537, #10637, #8867, #7295, #11993, #7509, #8655, #15027, #2475, #18391, #20068, #17012, #13872, #2689, #11887 ),
 ( #19863, #20272, #20173, #708, #5733, #15337, #4256, #16698, #15447, #5833, #12202, #7196, #16589, #9076, #1131, #7094, #2578, #4054, #10438, #16807, #10221, #13558, #13459, #18279, #909, #12303, #10329, #3942, #18699, #4155, #16907, #2376, #13658, #8766, #15137, #19959, #1018, #8963, #5619, #15236, #12104, #18493, #7408, #1532, #10952, #17318, #7605, #9578, #10748, #6040, #12608, #20487, #18909, #14386, #6237, #15952, #4772, #20685, #4666, #4567, #15853, #14079, #12716, #6456, #3108, #17120, #69, #19119, #3003, #2800, #6142, #3207, #9378, #12512, #1334, #13972, #11057, #14177, #4472, #9174, #15549, #17430, #20585, #7815, #1634, #9484 ),
 ( #19012, #7912, #11157, #10856, #8016, #14275, #6347, #7711, #1229, #17527, #12819, #20377, #4365, #15753, #1436, #12411, #18806, #17220, #2898, #9273, #15647, #14901, #19319, #169, #11251, #6553, #379, #3609, #9992, #6857, #14590, #19429, #19219, #3411, #577, #2050, #16372, #9792, #6957, #4976, #5281, #6763, #17630, #13132, #13226, #11560, #11658, #1841, #265, #4873, #19530, #11356, #8435, #8126, #5182, #17941, #3304, #14804, #16177, #12916, #17745, #9685, #8226, #6656, #17845, #16072, #14492, #19623, #1743, #13026, #481, #18051, #3510, #16271, #5085, #16475, #11464, #9891, #1940, #8324, #14698, #3721, #2148, #10099, #8529, #18565 ),
 ( #2661, #2553, #11764, #8844, #18468, #7380, #19839, #4230, #16882, #8939, #10302, #19729, #13744, #20146, #10199, #5706, #788, #15111, #7173, #13330, #16673, #5390, #18156, #4027, #9050, #13434, #15002, #3820, #683, #15211, #4130, #10511, #992, #8742, #13536, #16568, #18258, #15419, #15310, #5806, #3920, #1104, #5491, #12177, #887, #2245, #7272, #10611, #12077, #16983, #2349, #19938, #8631, #13633, #11864, #7069, #5596, #20042, #11966, #18366, #10411, #16783, #2451, #13943, #12276, #9151, #6010, #6117, #18668, #6314, #7580, #3083, #4542, #20345, #14154, #18880, #15618, #15519, #20561, #14247, #1506, #9248, #11132, #17291, #1204, #2871 ),
 ( #20657, #17195, #12386, #17501, #7482, #20460, #6212, #12583, #12689, #10926, #13843, #19091, #9555, #1410, #11031, #18779, #4745, #10829, #1301, #20246, #7791, #4446, #18983, #17094, #4639, #17402, #5904, #9457, #7683, #14052, #12488, #4338, #2973, #9350, #15729, #10721, #3181, #15829, #7888, #15928, #2771, #8298, #12999, #9766, #3278, #14672, #8411, #16346, #3388, #5254, #11437, #9657, #17717, #1719, #6739, #14568, #14778, #11329, #8103, #11631, #1605, #241, #352, #13104, #455, #19402, #7986, #6833, #3692, #16248, #5158, #12893, #17606, #9964, #14358, #18021, #1917, #2021, #6630, #5060, #16152, #19601, #44, #6429, #17821, #1816 ),
 ( #19507, #3488, #9864, #13202, #11537, #10076, #17916, #3583, #8202, #12793, #19195, #4848, #11229, #16044, #14467, #146, #6532, #19297, #4950, #8505, #18443, #12048, #18232, #2221, #16757, #15082, #3999, #16545, #10385, #7042, #764, #8820, #16858, #15187, #3798, #4105, #864, #2322, #8604, #2428, #14975, #5677, #7247, #13299, #19700, #10488, #2525, #16450, #7150, #13609, #2124, #16642, #13513, #552, #5363, #19915, #20013, #14876, #6932, #10175, #653, #5569, #11741, #18133, #13410, #19815, #18336, #5469, #11841, #11940, #3895, #10274, #8711, #8367, #418, #14426, #17882, #6591, #8166, #18097, #5219, #13166, #16111, #14532, #19663, #6895 ),
 ( #311, #17674, #5325, #109, #1779, #1981, #9827, #8262, #3762, #16309, #11699, #14840, #10034, #14742, #14628, #11597, #3450, #2088, #16513, #19566, #6495, #10140, #8473, #6696, #12856, #16213, #13264, #19467, #1881, #11397, #3347, #6798, #3549, #207, #19258, #4911, #17982, #9928, #3652, #2185, #16413, #11289, #5122, #515, #13068, #11502, #9726, #12959, #19360, #5017, #17782, #18294, #5433, #4354, #13861, #7004, #6133, #20477, #15437, #13475, #18795, #10739, #20366, #7112, #6028, #3957, #17109, #10846, #10940, #17209, #15043, #12502, #2886, #12292, #19878, #4461, #5532, #14068, #9264, #11806, #18195, #4557, #17308, #8568, #18687, #15635 ) ),
 .UNSPECIFIED., .T., .F., .F. ) 
 B_SPLINE_SURFACE_WITH_KNOTS ( ( 4, 3, 4 ),
 ( 4, 2, 2, 2, 2, 2, 2, 2, 2, 2, 2, 2, 2, 2, 2, 2, 2, 2, 2, 2, 2, 2, 2, 2, 2, 2, 2, 2, 2, 2, 2, 2, 2, 2, 2, 2, 2, 2, 2, 2, 2, 2, 4 ),
 ( 0.000000000000000000, 0.5000000000000000000, 1.000000000000000000 ),
 ( 0.000000000000000000, 0.03481082764294501225, 0.05122453910963481460, 0.05943139484297971231, 0.06353482270965216117, 0.06763825057632461002, 0.07081696859385246123, 0.07399568661138031245, 0.08035312264643601488, 0.09306799471654741973, 0.1057828667866588246, 0.1121403028217145270, 0.1153190208392423644, 0.1184977388567702156, 0.1214804596100246270, 0.1244631803632790246, 0.1304286218697878197, 0.1423595048828054099, 0.1662212709088405904, 0.2139448029609109514, 0.3093918670650516733, 0.5002859952733331728, 0.6911801234816146167, 0.7866271875857553386, 0.8343507196378256996, 0.8582124856638608801, 0.8701433686768784703, 0.8761088101833873765, 0.8790915309366418295, 0.8820742516898961716, 0.8853411830926052328, 0.8886081144953141830, 0.8951419773007323055, 0.9082097029115685505, 0.9212774285224047954, 0.9278112913278229179, 0.9310782227305318681, 0.9343451541332409294, 0.9384485819999133227, 0.9425520098665858271, 0.9507588655999306138, 0.9671725770666204092, 1.000000000000000000 ),
 .UNSPECIFIED. ) 
 GEOMETRIC_REPRESENTATION_ITEM ( )  RATIONAL_B_SPLINE_SURFACE ( (
 ( 1.000000000000000000, 1.000000000000000000, 1.000000000000000000, 1.000000000000000000, 1.000000000000000000, 1.000000000000000000, 1.000000000000000000, 1.000000000000000000, 1.000000000000000000, 1.000000000000000000, 1.000000000000000000, 1.000000000000000000, 1.000000000000000000, 1.000000000000000000, 1.000000000000000000, 1.000000000000000000, 1.000000000000000000, 1.000000000000000000, 1.000000000000000000, 1.000000000000000000, 1.000000000000000000, 1.000000000000000000, 1.000000000000000000, 1.000000000000000000, 1.000000000000000000, 1.000000000000000000, 1.000000000000000000, 1.000000000000000000, 1.000000000000000000, 1.000000000000000000, 1.000000000000000000, 1.000000000000000000, 1.000000000000000000, 1.000000000000000000, 1.000000000000000000, 1.000000000000000000, 1.000000000000000000, 1.000000000000000000, 1.000000000000000000, 1.000000000000000000, 1.000000000000000000, 1.000000000000000000, 1.000000000000000000, 1.000000000000000000, 1.000000000000000000, 1.000000000000000000, 1.000000000000000000, 1.000000000000000000, 1.000000000000000000, 1.000000000000000000, 1.000000000000000000, 1.000000000000000000, 1.000000000000000000, 1.000000000000000000, 1.000000000000000000, 1.000000000000000000, 1.000000000000000000, 1.000000000000000000, 1.000000000000000000, 1.000000000000000000, 1.000000000000000000, 1.000000000000000000, 1.000000000000000000, 1.000000000000000000, 1.000000000000000000, 1.000000000000000000, 1.000000000000000000, 1.000000000000000000, 1.000000000000000000, 1.000000000000000000, 1.000000000000000000, 1.000000000000000000, 1.000000000000000000, 1.000000000000000000, 1.000000000000000000, 1.000000000000000000, 1.000000000000000000, 1.000000000000000000, 1.000000000000000000, 1.000000000000000000, 1.000000000000000000, 1.000000000000000000, 1.000000000000000000, 1.000000000000000000, 1.000000000000000000, 1.000000000000000000),
 ( 0.3333333333333333703, 0.3333333333333333703, 0.3333333333333333703, 0.3333333333333333703, 0.3333333333333333703, 0.3333333333333333703, 0.3333333333333333703, 0.3333333333333333703, 0.3333333333333333703, 0.3333333333333333703, 0.3333333333333333703, 0.3333333333333333703, 0.3333333333333333703, 0.3333333333333333703, 0.3333333333333333703, 0.3333333333333333703, 0.3333333333333333703, 0.3333333333333333703, 0.3333333333333333703, 0.3333333333333333703, 0.3333333333333333703, 0.3333333333333333703, 0.3333333333333333703, 0.3333333333333333703, 0.3333333333333333703, 0.3333333333333333703, 0.3333333333333333703, 0.3333333333333333703, 0.3333333333333333703, 0.3333333333333333703, 0.3333333333333333703, 0.3333333333333333703, 0.3333333333333333703, 0.3333333333333333703, 0.3333333333333333703, 0.3333333333333333703, 0.3333333333333333703, 0.3333333333333333703, 0.3333333333333333703, 0.3333333333333333703, 0.3333333333333333703, 0.3333333333333333703, 0.3333333333333333703, 0.3333333333333333703, 0.3333333333333333703, 0.3333333333333333703, 0.3333333333333333703, 0.3333333333333333703, 0.3333333333333333703, 0.3333333333333333703, 0.3333333333333333703, 0.3333333333333333703, 0.3333333333333333703, 0.3333333333333333703, 0.3333333333333333703, 0.3333333333333333703, 0.3333333333333333703, 0.3333333333333333703, 0.3333333333333333703, 0.3333333333333333703, 0.3333333333333333703, 0.3333333333333333703, 0.3333333333333333703, 0.3333333333333333703, 0.3333333333333333703, 0.3333333333333333703, 0.3333333333333333703, 0.3333333333333333703, 0.3333333333333333703, 0.3333333333333333703, 0.3333333333333333703, 0.3333333333333333703, 0.3333333333333333703, 0.3333333333333333703, 0.3333333333333333703, 0.3333333333333333703, 0.3333333333333333703, 0.3333333333333333703, 0.3333333333333333703, 0.3333333333333333703, 0.3333333333333333703, 0.3333333333333333703, 0.3333333333333333703, 0.3333333333333333703, 0.3333333333333333703, 0.3333333333333333703),
 ( 0.3333333333333333703, 0.3333333333333333703, 0.3333333333333333703, 0.3333333333333333703, 0.3333333333333333703, 0.3333333333333333703, 0.3333333333333333703, 0.3333333333333333703, 0.3333333333333333703, 0.3333333333333333703, 0.3333333333333333703, 0.3333333333333333703, 0.3333333333333333703, 0.3333333333333333703, 0.3333333333333333703, 0.3333333333333333703, 0.3333333333333333703, 0.3333333333333333703, 0.3333333333333333703, 0.3333333333333333703, 0.3333333333333333703, 0.3333333333333333703, 0.3333333333333333703, 0.3333333333333333703, 0.3333333333333333703, 0.3333333333333333703, 0.3333333333333333703, 0.3333333333333333703, 0.3333333333333333703, 0.3333333333333333703, 0.3333333333333333703, 0.3333333333333333703, 0.3333333333333333703, 0.3333333333333333703, 0.3333333333333333703, 0.3333333333333333703, 0.3333333333333333703, 0.3333333333333333703, 0.3333333333333333703, 0.3333333333333333703, 0.3333333333333333703, 0.3333333333333333703, 0.3333333333333333703, 0.3333333333333333703, 0.3333333333333333703, 0.3333333333333333703, 0.3333333333333333703, 0.3333333333333333703, 0.3333333333333333703, 0.3333333333333333703, 0.3333333333333333703, 0.3333333333333333703, 0.3333333333333333703, 0.3333333333333333703, 0.3333333333333333703, 0.3333333333333333703, 0.3333333333333333703, 0.3333333333333333703, 0.3333333333333333703, 0.3333333333333333703, 0.3333333333333333703, 0.3333333333333333703, 0.3333333333333333703, 0.3333333333333333703, 0.3333333333333333703, 0.3333333333333333703, 0.3333333333333333703, 0.3333333333333333703, 0.3333333333333333703, 0.3333333333333333703, 0.3333333333333333703, 0.3333333333333333703, 0.3333333333333333703, 0.3333333333333333703, 0.3333333333333333703, 0.3333333333333333703, 0.3333333333333333703, 0.3333333333333333703, 0.3333333333333333703, 0.3333333333333333703, 0.3333333333333333703, 0.3333333333333333703, 0.3333333333333333703, 0.3333333333333333703, 0.3333333333333333703, 0.3333333333333333703),
 ( 1.000000000000000000, 1.000000000000000000, 1.000000000000000000, 1.000000000000000000, 1.000000000000000000, 1.000000000000000000, 1.000000000000000000, 1.000000000000000000, 1.000000000000000000, 1.000000000000000000, 1.000000000000000000, 1.000000000000000000, 1.000000000000000000, 1.000000000000000000, 1.000000000000000000, 1.000000000000000000, 1.000000000000000000, 1.000000000000000000, 1.000000000000000000, 1.000000000000000000, 1.000000000000000000, 1.000000000000000000, 1.000000000000000000, 1.000000000000000000, 1.000000000000000000, 1.000000000000000000, 1.000000000000000000, 1.000000000000000000, 1.000000000000000000, 1.000000000000000000, 1.000000000000000000, 1.000000000000000000, 1.000000000000000000, 1.000000000000000000, 1.000000000000000000, 1.000000000000000000, 1.000000000000000000, 1.000000000000000000, 1.000000000000000000, 1.000000000000000000, 1.000000000000000000, 1.000000000000000000, 1.000000000000000000, 1.000000000000000000, 1.000000000000000000, 1.000000000000000000, 1.000000000000000000, 1.000000000000000000, 1.000000000000000000, 1.000000000000000000, 1.000000000000000000, 1.000000000000000000, 1.000000000000000000, 1.000000000000000000, 1.000000000000000000, 1.000000000000000000, 1.000000000000000000, 1.000000000000000000, 1.000000000000000000, 1.000000000000000000, 1.000000000000000000, 1.000000000000000000, 1.000000000000000000, 1.000000000000000000, 1.000000000000000000, 1.000000000000000000, 1.000000000000000000, 1.000000000000000000, 1.000000000000000000, 1.000000000000000000, 1.000000000000000000, 1.000000000000000000, 1.000000000000000000, 1.000000000000000000, 1.000000000000000000, 1.000000000000000000, 1.000000000000000000, 1.000000000000000000, 1.000000000000000000, 1.000000000000000000, 1.000000000000000000, 1.000000000000000000, 1.000000000000000000, 1.000000000000000000, 1.000000000000000000, 1.000000000000000000),
 ( 0.3333333333333333703, 0.3333333333333333703, 0.3333333333333333703, 0.3333333333333333703, 0.3333333333333333703, 0.3333333333333333703, 0.3333333333333333703, 0.3333333333333333703, 0.3333333333333333703, 0.3333333333333333703, 0.3333333333333333703, 0.3333333333333333703, 0.3333333333333333703, 0.3333333333333333703, 0.3333333333333333703, 0.3333333333333333703, 0.3333333333333333703, 0.3333333333333333703, 0.3333333333333333703, 0.3333333333333333703, 0.3333333333333333703, 0.3333333333333333703, 0.3333333333333333703, 0.3333333333333333703, 0.3333333333333333703, 0.3333333333333333703, 0.3333333333333333703, 0.3333333333333333703, 0.3333333333333333703, 0.3333333333333333703, 0.3333333333333333703, 0.3333333333333333703, 0.3333333333333333703, 0.3333333333333333703, 0.3333333333333333703, 0.3333333333333333703, 0.3333333333333333703, 0.3333333333333333703, 0.3333333333333333703, 0.3333333333333333703, 0.3333333333333333703, 0.3333333333333333703, 0.3333333333333333703, 0.3333333333333333703, 0.3333333333333333703, 0.3333333333333333703, 0.3333333333333333703, 0.3333333333333333703, 0.3333333333333333703, 0.3333333333333333703, 0.3333333333333333703, 0.3333333333333333703, 0.3333333333333333703, 0.3333333333333333703, 0.3333333333333333703, 0.3333333333333333703, 0.3333333333333333703, 0.3333333333333333703, 0.3333333333333333703, 0.3333333333333333703, 0.3333333333333333703, 0.3333333333333333703, 0.3333333333333333703, 0.3333333333333333703, 0.3333333333333333703, 0.3333333333333333703, 0.3333333333333333703, 0.3333333333333333703, 0.3333333333333333703, 0.3333333333333333703, 0.3333333333333333703, 0.3333333333333333703, 0.3333333333333333703, 0.3333333333333333703, 0.3333333333333333703, 0.3333333333333333703, 0.3333333333333333703, 0.3333333333333333703, 0.3333333333333333703, 0.3333333333333333703, 0.3333333333333333703, 0.3333333333333333703, 0.3333333333333333703, 0.3333333333333333703, 0.3333333333333333703, 0.3333333333333333703),
 ( 0.3333333333333333703, 0.3333333333333333703, 0.3333333333333333703, 0.3333333333333333703, 0.3333333333333333703, 0.3333333333333333703, 0.3333333333333333703, 0.3333333333333333703, 0.3333333333333333703, 0.3333333333333333703, 0.3333333333333333703, 0.3333333333333333703, 0.3333333333333333703, 0.3333333333333333703, 0.3333333333333333703, 0.3333333333333333703, 0.3333333333333333703, 0.3333333333333333703, 0.3333333333333333703, 0.3333333333333333703, 0.3333333333333333703, 0.3333333333333333703, 0.3333333333333333703, 0.3333333333333333703, 0.3333333333333333703, 0.3333333333333333703, 0.3333333333333333703, 0.3333333333333333703, 0.3333333333333333703, 0.3333333333333333703, 0.3333333333333333703, 0.3333333333333333703, 0.3333333333333333703, 0.3333333333333333703, 0.3333333333333333703, 0.3333333333333333703, 0.3333333333333333703, 0.3333333333333333703, 0.3333333333333333703, 0.3333333333333333703, 0.3333333333333333703, 0.3333333333333333703, 0.3333333333333333703, 0.3333333333333333703, 0.3333333333333333703, 0.3333333333333333703, 0.3333333333333333703, 0.3333333333333333703, 0.3333333333333333703, 0.3333333333333333703, 0.3333333333333333703, 0.3333333333333333703, 0.3333333333333333703, 0.3333333333333333703, 0.3333333333333333703, 0.3333333333333333703, 0.3333333333333333703, 0.3333333333333333703, 0.3333333333333333703, 0.3333333333333333703, 0.3333333333333333703, 0.3333333333333333703, 0.3333333333333333703, 0.3333333333333333703, 0.3333333333333333703, 0.3333333333333333703, 0.3333333333333333703, 0.3333333333333333703, 0.3333333333333333703, 0.3333333333333333703, 0.3333333333333333703, 0.3333333333333333703, 0.3333333333333333703, 0.3333333333333333703, 0.3333333333333333703, 0.3333333333333333703, 0.3333333333333333703, 0.3333333333333333703, 0.3333333333333333703, 0.3333333333333333703, 0.3333333333333333703, 0.3333333333333333703, 0.3333333333333333703, 0.3333333333333333703, 0.3333333333333333703, 0.3333333333333333703),
 ( 1.000000000000000000, 1.000000000000000000, 1.000000000000000000, 1.000000000000000000, 1.000000000000000000, 1.000000000000000000, 1.000000000000000000, 1.000000000000000000, 1.000000000000000000, 1.000000000000000000, 1.000000000000000000, 1.000000000000000000, 1.000000000000000000, 1.000000000000000000, 1.000000000000000000, 1.000000000000000000, 1.000000000000000000, 1.000000000000000000, 1.000000000000000000, 1.000000000000000000, 1.000000000000000000, 1.000000000000000000, 1.000000000000000000, 1.000000000000000000, 1.000000000000000000, 1.000000000000000000, 1.000000000000000000, 1.000000000000000000, 1.000000000000000000, 1.000000000000000000, 1.000000000000000000, 1.000000000000000000, 1.000000000000000000, 1.000000000000000000, 1.000000000000000000, 1.000000000000000000, 1.000000000000000000, 1.000000000000000000, 1.000000000000000000, 1.000000000000000000, 1.000000000000000000, 1.000000000000000000, 1.000000000000000000, 1.000000000000000000, 1.000000000000000000, 1.000000000000000000, 1.000000000000000000, 1.000000000000000000, 1.000000000000000000, 1.000000000000000000, 1.000000000000000000, 1.000000000000000000, 1.000000000000000000, 1.000000000000000000, 1.000000000000000000, 1.000000000000000000, 1.000000000000000000, 1.000000000000000000, 1.000000000000000000, 1.000000000000000000, 1.000000000000000000, 1.000000000000000000, 1.000000000000000000, 1.000000000000000000, 1.000000000000000000, 1.000000000000000000, 1.000000000000000000, 1.000000000000000000, 1.000000000000000000, 1.000000000000000000, 1.000000000000000000, 1.000000000000000000, 1.000000000000000000, 1.000000000000000000, 1.000000000000000000, 1.000000000000000000, 1.000000000000000000, 1.000000000000000000, 1.000000000000000000, 1.000000000000000000, 1.000000000000000000, 1.000000000000000000, 1.000000000000000000, 1.000000000000000000, 1.000000000000000000, 1.000000000000000000) ) ) 
 REPRESENTATION_ITEM ( '' )  SURFACE ( )  );
#3893=CARTESIAN_POINT ( 'NONE',  ( -12.62155858231679417, -23.74999999999999645, 3.550687472877651629 ) ) ;
#3895=CARTESIAN_POINT ( 'NONE',  ( 13.15384296923648400, 5.706569946443514674, 5.461568745250741763 ) ) ;
#3896=CARTESIAN_POINT ( 'NONE',  ( 12.72590726430969532, -14.40418315237199742, 4.861678440007700885 ) ) ;
#3907=CARTESIAN_POINT ( 'NONE',  ( 1.904508877737772998, -9.138371295333994837, 2.378667276417936627 ) ) ;
#3910=CARTESIAN_POINT ( 'NONE',  ( 13.23867574658679303, -20.53938148496870042, 3.467514063319057982 ) ) ;
#3911=CARTESIAN_POINT ( 'NONE',  ( -1.797604806073912709, -9.120796646272857799, 2.374153755450133740 ) ) ;
#3912=CARTESIAN_POINT ( 'NONE',  ( -6.246558582316794173, -21.94931252712234482, 5.250000000000000888 ) ) ;
#3913=CARTESIAN_POINT ( 'NONE',  ( -2.616191246582922680, -8.630616848980537270, 2.440880773935528048 ) ) ;
#3915=CARTESIAN_POINT ( 'NONE',  ( -13.38929389708972195, -18.77815819697223887, 4.753083296715700179 ) ) ;
#3916=CARTESIAN_POINT ( 'NONE',  ( -5.309058582316794173, -23.27327832286945153, 2.298404588716537411 ) ) ;
#3917=CARTESIAN_POINT ( 'NONE',  ( 8.496558582316795949, -22.05068747287764452, 0.9999999999999978906 ) ) ;
#3918=CARTESIAN_POINT ( 'NONE',  ( -7.940941417683175629, -21.25705176302044208, 2.828734674606458555 ) ) ;
#3919=ORIENTED_EDGE ( 'NONE', *, *, #1049, .F. ) ;
#3920=CARTESIAN_POINT ( 'NONE',  ( 13.49014615398506045, -14.43511922376608680, 5.596513032956658584 ) ) ;
#3928=CARTESIAN_POINT ( 'NONE',  ( 4.565941417683176518, -23.20159541128344927, 2.226721677130534705 ) ) ;
#3931=CARTESIAN_POINT ( 'NONE',  ( 3.336296098497695262, -9.936854405034125648, 2.776348673047012383 ) ) ;
#3934=CARTESIAN_POINT ( 'NONE',  ( 13.89730118381875279, 5.376209782841177898, 6.083536567043803522 ) ) ;
#3936=CARTESIAN_POINT ( 'NONE',  ( 9.159691417683175629, -22.36352608949543352, 2.479004561291652031 ) ) ;
#3937=CARTESIAN_POINT ( 'NONE',  ( -12.64323021897839006, -19.32937394158751943, 5.504219675487169283 ) ) ;
#3938=CARTESIAN_POINT ( 'NONE',  ( -7.190941417683177406, -22.74294823697955081, 4.171265325393542334 ) ) ;
#3939=CARTESIAN_POINT ( 'NONE',  ( -10.94094141768317741, -20.19639159124061933, 1.768074502826635586 ) ) ;
#3942=CARTESIAN_POINT ( 'NONE',  ( 12.63036675113625407, -19.22897906761645004, 4.757923088130392664 ) ) ;
#3943=CARTESIAN_POINT ( 'NONE',  ( -13.12512971825177033, 5.006550771716304915, 5.133277049491872468 ) ) ;
#3954=CARTESIAN_POINT ( 'NONE',  ( -3.502569552650398155, -9.961070227720959736, 2.032567780072621400 ) ) ;
#3957=CARTESIAN_POINT ( 'NONE',  ( 13.11514659413808737, 4.502403003978772134, 5.887634658581065494 ) ) ;
#3959=CARTESIAN_POINT ( 'NONE',  ( 10.09719141768317741, -23.08622137881040359, 5.979004561291654696 ) ) ;
#3960=CARTESIAN_POINT ( 'NONE',  ( -13.09293046926041626, 3.380488697651010011, 5.994170676248444352 ) ) ;
#3961=CARTESIAN_POINT ( 'NONE',  ( -8.315941417683177406, -20.26807450282663225, 5.303608408759377113 ) ) ;
#3966=CARTESIAN_POINT ( 'NONE',  ( -13.79242507427300879, 0.07996625081441015304, 6.658692769197546824 ) ) ;
#3969=CARTESIAN_POINT ( 'NONE',  ( 4.934058582316795061, -22.67126532539354855, 4.242948236979545484 ) ) ;
#3974=CARTESIAN_POINT ( 'NONE',  ( 13.39296152110871851, -19.34294318400601753, 5.489418334493660012 ) ) ;
#3983=CARTESIAN_POINT ( 'NONE',  ( 13.41341218697771609, -18.31018455762212227, 5.513179699623425023 ) ) ;
#3986=CARTESIAN_POINT ( 'NONE',  ( 2.616191246582922680, -8.630616848980537270, 2.440880773935528048 ) ) ;
#3989=CARTESIAN_POINT ( 'NONE',  ( -13.12529397353891270, 5.014845663890295846, 3.333333333333220239 ) ) ;
#3990=DIRECTION ( 'NONE',  ( 0.000000000000000000, -0.000000000000000000, -1.000000000000000000 ) ) ;
#3991=CARTESIAN_POINT ( 'NONE',  ( 12.62155858231679417, -23.74999999999999645, 3.550687472877651629 ) ) ;
#3992=CARTESIAN_POINT ( 'NONE',  ( -13.86316420010827777, 3.652292105464413297, 6.735515685864076119 ) ) ;
#3995=CARTESIAN_POINT ( 'NONE',  ( 11.59030858231679417, -21.32581373872472597, 1.729004561291657582 ) ) ;
#3996=CARTESIAN_POINT ( 'NONE',  ( 10.00344141768317563, -22.05068747287765873, 5.250000000000000888 ) ) ;
#3997=CARTESIAN_POINT ( 'NONE',  ( -12.90280858231679773, -22.77556120703056308, 1.770995438708339975 ) ) ;
#3999=CARTESIAN_POINT ( 'NONE',  ( 12.65816212372154403, -19.32531275206247301, 6.255900543948403225 ) ) ;
#4001=CARTESIAN_POINT ( 'NONE',  ( 12.62499994688180749, -19.50000268246798640, 4.473800639250938183 ) ) ;
#4012=CARTESIAN_POINT ( 'NONE',  ( 1.732184490400474175, -9.869581059509965115, 2.373841568485653308 ) ) ;
#4013=CARTESIAN_POINT ( 'NONE',  ( 13.87470602645761808, 4.985154336109792972, 4.000000000000000000 ) ) ;
#4018=CARTESIAN_POINT ( 'NONE',  ( -10.55905858231679595, -20.72672167713054137, 4.701595411283463477 ) ) ;
#4019=CARTESIAN_POINT ( 'NONE',  ( -2.121089610268797276, -8.411987239090384705, 1.634732322550447758 ) ) ;
#4021=CARTESIAN_POINT ( 'NONE',  ( -13.53317008522746434, -11.51241069598931510, 4.909333296715523431 ) ) ;
#4022=CARTESIAN_POINT ( 'NONE',  ( -9.059058582316794173, -20.72672167713054137, 4.701595411283463477 ) ) ;
#4024=CARTESIAN_POINT ( 'NONE',  ( 12.80905858231679417, -23.80360840875935935, 1.768074502826626260 ) ) ;
#4025=CARTESIAN_POINT ( 'NONE',  ( -11.69094141768317741, -22.74294823697955081, 4.171265325393542334 ) ) ;
#4027=CARTESIAN_POINT ( 'NONE',  ( 13.39107665282975645, -19.43812903209671461, 5.476542851584349947 ) ) ;
#4033=CARTESIAN_POINT ( 'NONE',  ( -13.38800411018677572, -19.59329243556743805, 5.436267741224407146 ) ) ;
#4043=CARTESIAN_POINT ( 'NONE',  ( 3.321934647848983957, -9.834888441627915867, 2.750161776669472591 ) ) ;
#4046=CARTESIAN_POINT ( 'NONE',  ( 12.63806878948643231, -20.34002613093225520, 5.891296472647073124 ) ) ;
#4047=DIRECTION ( 'NONE',  ( -1.000000000000000000, 0.000000000000000000, 0.000000000000000000 ) ) ;
#4049=CARTESIAN_POINT ( 'NONE',  ( 11.69094141768317741, -22.74294823697955081, 4.171265325393542334 ) ) ;
#4050=CARTESIAN_POINT ( 'NONE',  ( -12.62499999999998224, -20.25000000000006395, 4.416666666666681174 ) ) ;
#4051=CARTESIAN_POINT ( 'NONE',  ( -7.097191417683176518, -22.46490103525075810, 4.479004561291653808 ) ) ;
#4052=CARTESIAN_POINT ( 'NONE',  ( -9.815941417683177406, -20.26807450282663225, 5.303608408759377113 ) ) ;
#4054=CARTESIAN_POINT ( 'NONE',  ( 12.62562661273123332, -19.46835605706984040, 4.628101975944573176 ) ) ;
#4055=CARTESIAN_POINT ( 'NONE',  ( -13.12529397354238192, 5.014845663890295846, 4.666666666666619889 ) ) ;
#4066=CARTESIAN_POINT ( 'NONE',  ( -3.002445346198714837, -11.66215945560911749, 2.276826493710632171 ) ) ;
#4071=CARTESIAN_POINT ( 'NONE',  ( 11.87844141768317741, -24.50000000000000000, 3.449312527122335048 ) ) ;
#4072=CARTESIAN_POINT ( 'NONE',  ( -12.64387510712649565, -19.29680709011273976, 5.506486987317513737 ) ) ;
#4073=CARTESIAN_POINT ( 'NONE',  ( -9.628441417683177406, -19.49999999999998934, 3.550687472877664952 ) ) ;
#4075=CARTESIAN_POINT ( 'NONE',  ( 12.34030858231679240, -22.67418626127525982, 5.270995438708342640 ) ) ;
#4077=CARTESIAN_POINT ( 'NONE',  ( -13.86616162069444691, 3.803661845068127878, 6.738770894197415373 ) ) ;
#4078=CARTESIAN_POINT ( 'NONE',  ( 12.24655858231679240, -21.94931252712234482, 5.250000000000000888 ) ) ;
#4082=CARTESIAN_POINT ( 'NONE',  ( 13.83544900551672185, 3.002674778589386140, 5.971513032956590195 ) ) ;
#4091=CARTESIAN_POINT ( 'NONE',  ( 13.87467358130843387, 4.983515856073828409, 5.065827972856573602 ) ) ;
#4093=CARTESIAN_POINT ( 'NONE',  ( 3.528325504133930313, -10.14411005961392398, 2.079576065490765124 ) ) ;
#4096=CARTESIAN_POINT ( 'NONE',  ( -13.12529397354238192, 5.014845663890295846, 4.333333333333382775 ) ) ;
#4097=CARTESIAN_POINT ( 'NONE',  ( 10.84030858231679240, -22.67418626127525982, 5.270995438708342640 ) ) ;
#4098=CARTESIAN_POINT ( 'NONE',  ( -13.86616162069444691, 3.803661845068127878, 6.738770894197415373 ) ) ;
#4101=CARTESIAN_POINT ( 'NONE',  ( 10.65280858231679240, -21.22443879296942626, 5.229004561291659137 ) ) ;
#4102=CARTESIAN_POINT ( 'NONE',  ( 5.409691417683178294, -21.32581373872474373, 5.270995438708348857 ) ) ;
#4103=CARTESIAN_POINT ( 'NONE',  ( -12.99655858231679417, -22.05068747287764452, 1.749999999999998446 ) ) ;
#4105=CARTESIAN_POINT ( 'NONE',  ( 12.67822638532683577, -18.31206754099172684, 6.277704579156187847 ) ) ;
#4106=CARTESIAN_POINT ( 'NONE',  ( 12.62917185724685254, -19.28932120903463598, 4.753410794856941735 ) ) ;
#4113=CARTESIAN_POINT ( 'NONE',  ( -12.64387510712649565, -19.29680709011273976, 5.506486987317513737 ) ) ;
#4117=CARTESIAN_POINT ( 'NONE',  ( 1.824488249492779879, -9.124319963227819130, 2.375058613629473570 ) ) ;
#4121=CARTESIAN_POINT ( 'NONE',  ( -1.655860418491166941, -9.114909740826840689, 2.372641880528837621 ) ) ;
#4122=CARTESIAN_POINT ( 'NONE',  ( -12.90280858231679595, -23.08622137881038938, 1.020995438708339309 ) ) ;
#4123=CARTESIAN_POINT ( 'NONE',  ( -0.9854920305337621089, -9.114917468222230923, 1.622643865078341463 ) ) ;
#4125=CARTESIAN_POINT ( 'NONE',  ( -13.80173896975277437, 2.050317972508536535, 5.200999963382010094 ) ) ;
#4127=CARTESIAN_POINT ( 'NONE',  ( 9.253441417683177406, -21.94931252712233061, 0.9999999999999978906 ) ) ;
#4128=CARTESIAN_POINT ( 'NONE',  ( -8.315941417683177406, -21.32873467460645145, 4.242948236979555254 ) ) ;
#4130=CARTESIAN_POINT ( 'NONE',  ( 13.39722611581222189, -19.12758115148224647, 5.495601574623241170 ) ) ;
#4136=CARTESIAN_POINT ( 'NONE',  ( -13.83544900551672185, 3.002674778589386140, 5.971513032956590195 ) ) ;
#4141=( BOUNDED_SURFACE ( )  B_SPLINE_SURFACE ( 3, 3, ( 
 ( #18451, #8924, #15293, #974, #13724, #9032, #20129, #5790, #10594, #16966, #2644, #15402, #7466, #13825, #20229, #5889, #4321, #9230, #18763, #10704, #7563, #20329, #5993, #12368, #4428, #10812, #17589, #1702, #14035, #20545, #7775, #25, #7968, #10910, #17486, #3264, #17698, #9639, #1392, #12878 ),
 ( #20639, #6296, #6516, #15912, #6197, #3371, #19180, #6412, #14138, #17272, #12777, #18965, #4619, #2954, #16025, #4833, #12565, #7871, #15601, #20445, #17384, #9334, #8085, #14449, #132, #11014, #19282, #3066, #18865, #4933, #11314, #11215, #1286, #3167, #7666, #15710, #4525, #6101, #9440, #15813 ),
 ( #12471, #1490, #14231, #12669, #19072, #14341, #4729, #11116, #9539, #1589, #11422, #824, #3954, #724, #17806, #5632, #12007, #7108, #11801, #921, #5430, #15149, #9750, #13569, #14553, #614, #16133, #10137, #7001, #13368, #13472, #19874, #225, #8186, #5529, #2182, #18191, #1800, #6613, #12983 ),
 ( #10342, #16712, #19771, #3856, #4066, #2280, #10234, #11900, #18291, #2389, #5045, #16822, #18403, #10453, #16600, #2486, #8670, #19386, #8879, #15247, #7309, #13671, #8780, #12116, #3758, #16509, #8565, #15040, #14934, #7208, #19972, #20079, #5745, #18508, #10866, #15457, #10651, #12523, #20595, #4577 ),
 ( #15662, #18818, #15559, #5847, #20499, #6155, #1241, #5941, #15765, #20284, #9285, #4168, #7726, #8978, #1141, #10549, #4266, #7519, #13883, #7615, #13983, #15352, #2591, #20392, #17025, #12315, #16919, #1034, #7420, #6054, #12216, #4482, #13782, #18918, #18712, #14090, #9184, #4377, #17334, #20187 ),
 ( #18604, #2704, #9087, #10760, #17130, #2809, #12422, #17231, #10963, #12620, #1447, #2910, #1346, #3017, #9393, #7825, #14188, #6246, #277, #5096, #17441, #3217, #11169, #3425, #11368, #14285, #181, #6669, #391, #13040, #4784, #16283, #19441, #1755, #9803, #8336, #16189, #17540, #11477, #1543 ),
 ( #9589, #20698, #1854, #1649, #8032, #6361, #17857, #8238, #15965, #11262, #6774, #14400, #4679, #83, #12830, #3526, #9902, #1954, #14714, #3120, #6471, #19232, #14602, #17756, #12731, #6565, #19025, #11072, #9494, #4883, #15865, #7921, #8141, #19132, #17642, #3317, #9698, #16085, #14503, #12928 ) ),
 .UNSPECIFIED., .T., .F., .F. ) 
 B_SPLINE_SURFACE_WITH_KNOTS ( ( 4, 3, 4 ),
 ( 4, 2, 2, 2, 2, 2, 2, 2, 2, 2, 2, 2, 2, 2, 2, 2, 2, 2, 2, 4 ),
 ( 0.000000000000000000, 0.5000000000000000000, 1.000000000000000000 ),
 ( 0.000000000000000000, 0.3100443560520446118, 0.4650665340780669177, 0.5425776230910780429, 0.5813331675975836887, 0.6007109398508364562, 0.6200887121040892236, 0.6309950902025724950, 0.6419014683010558775, 0.6637142244980225314, 0.7073397368919559502, 0.7509652492858893691, 0.7727780054828560230, 0.7836843835813394055, 0.7945907616798226769, 0.8074288390748337596, 0.8202669164698448423, 0.8459430712598670077, 0.8972953808399113385, 1.000000000000000000 ),
 .UNSPECIFIED. ) 
 GEOMETRIC_REPRESENTATION_ITEM ( )  RATIONAL_B_SPLINE_SURFACE ( (
 ( 1.000000000000000000, 1.000000000000000000, 1.000000000000000000, 1.000000000000000000, 1.000000000000000000, 1.000000000000000000, 1.000000000000000000, 1.000000000000000000, 1.000000000000000000, 1.000000000000000000, 1.000000000000000000, 1.000000000000000000, 1.000000000000000000, 1.000000000000000000, 1.000000000000000000, 1.000000000000000000, 1.000000000000000000, 1.000000000000000000, 1.000000000000000000, 1.000000000000000000, 1.000000000000000000, 1.000000000000000000, 1.000000000000000000, 1.000000000000000000, 1.000000000000000000, 1.000000000000000000, 1.000000000000000000, 1.000000000000000000, 1.000000000000000000, 1.000000000000000000, 1.000000000000000000, 1.000000000000000000, 1.000000000000000000, 1.000000000000000000, 1.000000000000000000, 1.000000000000000000, 1.000000000000000000, 1.000000000000000000, 1.000000000000000000, 1.000000000000000000),
 ( 0.3333333333333333703, 0.3333333333333333703, 0.3333333333333333703, 0.3333333333333333703, 0.3333333333333333703, 0.3333333333333333703, 0.3333333333333333703, 0.3333333333333333703, 0.3333333333333333703, 0.3333333333333333703, 0.3333333333333333703, 0.3333333333333333703, 0.3333333333333333703, 0.3333333333333333703, 0.3333333333333333703, 0.3333333333333333703, 0.3333333333333333703, 0.3333333333333333703, 0.3333333333333333703, 0.3333333333333333703, 0.3333333333333333703, 0.3333333333333333703, 0.3333333333333333703, 0.3333333333333333703, 0.3333333333333333703, 0.3333333333333333703, 0.3333333333333333703, 0.3333333333333333703, 0.3333333333333333703, 0.3333333333333333703, 0.3333333333333333703, 0.3333333333333333703, 0.3333333333333333703, 0.3333333333333333703, 0.3333333333333333703, 0.3333333333333333703, 0.3333333333333333703, 0.3333333333333333703, 0.3333333333333333703, 0.3333333333333333703),
 ( 0.3333333333333333703, 0.3333333333333333703, 0.3333333333333333703, 0.3333333333333333703, 0.3333333333333333703, 0.3333333333333333703, 0.3333333333333333703, 0.3333333333333333703, 0.3333333333333333703, 0.3333333333333333703, 0.3333333333333333703, 0.3333333333333333703, 0.3333333333333333703, 0.3333333333333333703, 0.3333333333333333703, 0.3333333333333333703, 0.3333333333333333703, 0.3333333333333333703, 0.3333333333333333703, 0.3333333333333333703, 0.3333333333333333703, 0.3333333333333333703, 0.3333333333333333703, 0.3333333333333333703, 0.3333333333333333703, 0.3333333333333333703, 0.3333333333333333703, 0.3333333333333333703, 0.3333333333333333703, 0.3333333333333333703, 0.3333333333333333703, 0.3333333333333333703, 0.3333333333333333703, 0.3333333333333333703, 0.3333333333333333703, 0.3333333333333333703, 0.3333333333333333703, 0.3333333333333333703, 0.3333333333333333703, 0.3333333333333333703),
 ( 1.000000000000000000, 1.000000000000000000, 1.000000000000000000, 1.000000000000000000, 1.000000000000000000, 1.000000000000000000, 1.000000000000000000, 1.000000000000000000, 1.000000000000000000, 1.000000000000000000, 1.000000000000000000, 1.000000000000000000, 1.000000000000000000, 1.000000000000000000, 1.000000000000000000, 1.000000000000000000, 1.000000000000000000, 1.000000000000000000, 1.000000000000000000, 1.000000000000000000, 1.000000000000000000, 1.000000000000000000, 1.000000000000000000, 1.000000000000000000, 1.000000000000000000, 1.000000000000000000, 1.000000000000000000, 1.000000000000000000, 1.000000000000000000, 1.000000000000000000, 1.000000000000000000, 1.000000000000000000, 1.000000000000000000, 1.000000000000000000, 1.000000000000000000, 1.000000000000000000, 1.000000000000000000, 1.000000000000000000, 1.000000000000000000, 1.000000000000000000),
 ( 0.3333333333333333703, 0.3333333333333333703, 0.3333333333333333703, 0.3333333333333333703, 0.3333333333333333703, 0.3333333333333333703, 0.3333333333333333703, 0.3333333333333333703, 0.3333333333333333703, 0.3333333333333333703, 0.3333333333333333703, 0.3333333333333333703, 0.3333333333333333703, 0.3333333333333333703, 0.3333333333333333703, 0.3333333333333333703, 0.3333333333333333703, 0.3333333333333333703, 0.3333333333333333703, 0.3333333333333333703, 0.3333333333333333703, 0.3333333333333333703, 0.3333333333333333703, 0.3333333333333333703, 0.3333333333333333703, 0.3333333333333333703, 0.3333333333333333703, 0.3333333333333333703, 0.3333333333333333703, 0.3333333333333333703, 0.3333333333333333703, 0.3333333333333333703, 0.3333333333333333703, 0.3333333333333333703, 0.3333333333333333703, 0.3333333333333333703, 0.3333333333333333703, 0.3333333333333333703, 0.3333333333333333703, 0.3333333333333333703),
 ( 0.3333333333333333703, 0.3333333333333333703, 0.3333333333333333703, 0.3333333333333333703, 0.3333333333333333703, 0.3333333333333333703, 0.3333333333333333703, 0.3333333333333333703, 0.3333333333333333703, 0.3333333333333333703, 0.3333333333333333703, 0.3333333333333333703, 0.3333333333333333703, 0.3333333333333333703, 0.3333333333333333703, 0.3333333333333333703, 0.3333333333333333703, 0.3333333333333333703, 0.3333333333333333703, 0.3333333333333333703, 0.3333333333333333703, 0.3333333333333333703, 0.3333333333333333703, 0.3333333333333333703, 0.3333333333333333703, 0.3333333333333333703, 0.3333333333333333703, 0.3333333333333333703, 0.3333333333333333703, 0.3333333333333333703, 0.3333333333333333703, 0.3333333333333333703, 0.3333333333333333703, 0.3333333333333333703, 0.3333333333333333703, 0.3333333333333333703, 0.3333333333333333703, 0.3333333333333333703, 0.3333333333333333703, 0.3333333333333333703),
 ( 1.000000000000000000, 1.000000000000000000, 1.000000000000000000, 1.000000000000000000, 1.000000000000000000, 1.000000000000000000, 1.000000000000000000, 1.000000000000000000, 1.000000000000000000, 1.000000000000000000, 1.000000000000000000, 1.000000000000000000, 1.000000000000000000, 1.000000000000000000, 1.000000000000000000, 1.000000000000000000, 1.000000000000000000, 1.000000000000000000, 1.000000000000000000, 1.000000000000000000, 1.000000000000000000, 1.000000000000000000, 1.000000000000000000, 1.000000000000000000, 1.000000000000000000, 1.000000000000000000, 1.000000000000000000, 1.000000000000000000, 1.000000000000000000, 1.000000000000000000, 1.000000000000000000, 1.000000000000000000, 1.000000000000000000, 1.000000000000000000, 1.000000000000000000, 1.000000000000000000, 1.000000000000000000, 1.000000000000000000, 1.000000000000000000, 1.000000000000000000) ) ) 
 REPRESENTATION_ITEM ( '' )  SURFACE ( )  );
#4143=CARTESIAN_POINT ( 'NONE',  ( 3.882031223148668886, -13.81156101447257889, 3.771450735391772557 ) ) ;
#4145=CARTESIAN_POINT ( 'NONE',  ( 13.90394305879618386, 5.711624469205903942, 5.287712306078340418 ) ) ;
#4149=CARTESIAN_POINT ( 'NONE',  ( 12.53469141768317741, -20.97900456129164581, 3.136473910504570917 ) ) ;
#4150=CARTESIAN_POINT ( 'NONE',  ( -12.62499999998404121, -20.24999999996810729, 2.793053905886972998 ) ) ;
#4152=CARTESIAN_POINT ( 'NONE',  ( -13.37155858231679595, -20.99999999999999645, 3.449312527122348371 ) ) ;
#4153=CARTESIAN_POINT ( 'NONE',  ( -12.44094141768317741, -20.19639159124061933, 1.768074502826635586 ) ) ;
#4155=CARTESIAN_POINT ( 'NONE',  ( 12.63238774201960268, -19.12691902800888499, 4.760115940007608515 ) ) ;
#4156=CARTESIAN_POINT ( 'NONE',  ( -13.00900269284621302, -0.8578640112522492034, 5.903024842915844062 ) ) ;
#4168=CARTESIAN_POINT ( 'NONE',  ( -2.067263844777544435, -10.27417889452513933, 1.727750375171331676 ) ) ;
#4172=CARTESIAN_POINT ( 'NONE',  ( 4.717959273841179524, -21.63341328858655999, 5.993595146365859883 ) ) ;
#4173=CARTESIAN_POINT ( 'NONE',  ( -13.11017182064853159, 4.251176942750957366, 5.979809059808775196 ) ) ;
#4175=CARTESIAN_POINT ( 'NONE',  ( -5.784691417683178294, -24.52099543870834708, 4.484846433055073689 ) ) ;
#4176=ORIENTED_EDGE ( 'NONE', *, *, #16737, .T. ) ;
#4177=CARTESIAN_POINT ( 'NONE',  ( 12.62155858231679417, -23.74999999999999645, 3.550687472877651629 ) ) ;
#4179=CARTESIAN_POINT ( 'NONE',  ( -13.82120031190154208, 1.533115751011936867, 6.689942769197355865 ) ) ;
#4180=CARTESIAN_POINT ( 'NONE',  ( 4.717959273841179524, -21.82295283170803302, 4.493595146365858994 ) ) ;
#4183=ORIENTED_EDGE ( 'NONE', *, *, #3651, .T. ) ;
#4184=CARTESIAN_POINT ( 'NONE',  ( 13.39782821820594627, -19.84717498059871943, 6.143582220458365661 ) ) ;
#4191=CARTESIAN_POINT ( 'NONE',  ( -12.80905858231679417, -23.27327832286945153, 2.298404588716537411 ) ) ;
#4192=CARTESIAN_POINT ( 'NONE',  ( 13.86693669322925260, 4.592803008081209448, 5.801483467520450077 ) ) ;
#4195=CARTESIAN_POINT ( 'NONE',  ( 2.787023586469211001, -10.13267000451481614, 1.884023048047904103 ) ) ;
#4197=CARTESIAN_POINT ( 'NONE',  ( -13.37500000000002132, -19.49999999999450040, 3.833333333368183382 ) ) ;
#4198=CARTESIAN_POINT ( 'NONE',  ( 12.15280858231679595, -21.22443879296942626, 5.229004561291659137 ) ) ;
#4199=CARTESIAN_POINT ( 'NONE',  ( -13.56222317325195093, -11.54522975075300728, 6.408692769197242178 ) ) ;
#4202=CARTESIAN_POINT ( 'NONE',  ( 10.37155858231679417, -20.24999999999999289, 3.449312527122348371 ) ) ;
#4203=CARTESIAN_POINT ( 'NONE',  ( 10.56594141768317741, -22.67126532539353789, 2.757051763020445634 ) ) ;
#4204=CARTESIAN_POINT ( 'NONE',  ( -8.777808582316792396, -20.27099543870833642, 2.724438792969431589 ) ) ;
#4206=CARTESIAN_POINT ( 'NONE',  ( 13.09073190589589331, 4.019461247742575516, 5.257453802652931607 ) ) ;
#4213=CARTESIAN_POINT ( 'NONE',  ( -13.02818618459764188, 0.1109023222084986743, 5.923858176248589125 ) ) ;
#4215=CARTESIAN_POINT ( 'NONE',  ( -13.86693669322925260, 4.592803008081209448, 5.801483467520450077 ) ) ;
#4217=CARTESIAN_POINT ( 'NONE',  ( -12.62499999999998579, -20.24999999999999289, 3.666666666666653640 ) ) ;
#4221=CARTESIAN_POINT ( 'NONE',  ( -11.02780858231679595, -24.47900456129166358, 4.586221378810390270 ) ) ;
#4222=CARTESIAN_POINT ( 'NONE',  ( -2.722060606927515725, -8.660968749821154944, 1.698675748411476283 ) ) ;
#4224=CARTESIAN_POINT ( 'NONE',  ( -13.37499999999998579, -20.24999999999999289, 3.146526952850934755 ) ) ;
#4227=CARTESIAN_POINT ( 'NONE',  ( 10.75344141768317741, -21.94931252712233061, 0.9999999999999978906 ) ) ;
#4228=CARTESIAN_POINT ( 'NONE',  ( -9.159691417683175629, -22.36352608949543352, 2.479004561291652031 ) ) ;
#4230=CARTESIAN_POINT ( 'NONE',  ( 13.37499999999998224, -20.24999999999998934, 4.291666666666698937 ) ) ;
#4236=CARTESIAN_POINT ( 'NONE',  ( -13.87470602645761986, 4.985154336109792972, 4.833333333333344584 ) ) ;
#4245=CARTESIAN_POINT ( 'NONE',  ( 3.607313482701580476, -10.70492285834919244, 2.223603995567122293 ) ) ;
#4249=CARTESIAN_POINT ( 'NONE',  ( 13.12529397354238192, 5.014845663890295846, 3.666666666666500873 ) ) ;
#4250=CARTESIAN_POINT ( 'NONE',  ( 5.315941417683176518, -20.79840458871654363, 4.773278322869464851 ) ) ;
#4252=CARTESIAN_POINT ( 'NONE',  ( -10.84030858231679595, -22.36352608949544418, 4.520995438708343528 ) ) ;
#4254=CARTESIAN_POINT ( 'NONE',  ( -9.628441417683177406, -19.49999999999998934, 3.550687472877664952 ) ) ;
#4256=CARTESIAN_POINT ( 'NONE',  ( 12.62499999999998224, -19.49999999999998934, 4.166666666666637653 ) ) ;
#4257=CARTESIAN_POINT ( 'NONE',  ( -13.12270769621861355, 4.884238659038159902, 5.513847264053151065 ) ) ;
#4262=CARTESIAN_POINT ( 'NONE',  ( 2.109407804498405703, -9.207748739546751438, 2.396484790045401603 ) ) ;
#4266=CARTESIAN_POINT ( 'NONE',  ( -2.041623931606483033, -10.12028065167953272, 1.688226231982305370 ) ) ;
#4270=CARTESIAN_POINT ( 'NONE',  ( 6.996558582316795949, -22.05068747287764452, 0.9999999999999978906 ) ) ;
#4271=CARTESIAN_POINT ( 'NONE',  ( -12.64131715375063258, -19.42598373559290792, 5.491151580003103660 ) ) ;
#4273=CARTESIAN_POINT ( 'NONE',  ( -9.909691417683179182, -21.32581373872474373, 5.270995438708348857 ) ) ;
#4279=CARTESIAN_POINT ( 'NONE',  ( -13.40995420747273670, -19.23481252262645924, 6.243328185864100988 ) ) ;
#4280=CARTESIAN_POINT ( 'NONE',  ( 10.46530858231679417, -20.22900456129164937, 4.174186261275266929 ) ) ;
#4284=CARTESIAN_POINT ( 'NONE',  ( 13.41355111217617413, -19.05316883510194614, 6.247234435864091218 ) ) ;
#4293=CARTESIAN_POINT ( 'NONE',  ( -8.402808582316794173, -22.77556120703056308, 1.770995438708339975 ) ) ;
#4294=CARTESIAN_POINT ( 'NONE',  ( 13.87367531042247748, 4.933103176334663331, 5.324010972534209074 ) ) ;
#4296=CARTESIAN_POINT ( 'NONE',  ( 3.342893013439646843, -9.383962644129466568, 1.884355023724047173 ) ) ;
#4298=CARTESIAN_POINT ( 'NONE',  ( -13.08919463935856697, 3.941829287606363863, 5.256209690007596080 ) ) ;
#4301=CARTESIAN_POINT ( 'NONE',  ( -13.84997554952896515, 2.986265251207539606, 6.721192769197450012 ) ) ;
#4306=CARTESIAN_POINT ( 'NONE',  ( 9.996558582316794173, -22.05068747287764452, 1.749999999999998446 ) ) ;
#4307=CARTESIAN_POINT ( 'NONE',  ( 4.472191417683177406, -23.72900456129165292, 2.724438792969417822 ) ) ;
#4308=CARTESIAN_POINT ( 'NONE',  ( -5.684058582316794173, -20.79840458871652942, 2.226721677130544030 ) ) ;
#4310=CARTESIAN_POINT ( 'NONE',  ( 13.09533517714100093, 4.251926445620864747, 5.084080158857392284 ) ) ;
#4312=ORIENTED_EDGE ( 'NONE', *, *, #8911, .T. ) ;
#4318=CARTESIAN_POINT ( 'NONE',  ( -12.62499999999998224, -20.24999999999991829, 4.333333333333343695 ) ) ;
#4321=CARTESIAN_POINT ( 'NONE',  ( -2.559937518207947793, -9.746075135043517079, 2.534737762559237773 ) ) ;
#4322=CARTESIAN_POINT ( 'NONE',  ( -13.84863765609603625, 3.668701632846259830, 5.985835949623216301 ) ) ;
#4328=CARTESIAN_POINT ( 'NONE',  ( -10.46530858231679595, -19.47900456129164937, 4.484846433055089676 ) ) ;
#4329=CARTESIAN_POINT ( 'NONE',  ( -1.548630333695928396, -9.114917468222230923, 1.622643865078341463 ) ) ;
#4332=CARTESIAN_POINT ( 'NONE',  ( -13.37883250981221472, -20.05645825448334563, 5.102688967256983510 ) ) ;
#4334=CARTESIAN_POINT ( 'NONE',  ( 11.22219141768317741, -19.52099543870834353, 4.586221378810406257 ) ) ;
#4335=CARTESIAN_POINT ( 'NONE',  ( -7.378441417683177406, -22.99999999999999645, 3.449312527122335048 ) ) ;
#4336=AXIS2_PLACEMENT_3D ( 'NONE', #20659, #19094, #14469 ) ;
#4338=CARTESIAN_POINT ( 'NONE',  ( 13.41355111217617413, -19.05316883510194614, 6.247234435864091218 ) ) ;
#4339=FACE_OUTER_BOUND ( 'NONE', #8467, .T. ) ;
#4343=CIRCLE ( 'NONE', #15365, 0.3749999999999997224 ) ;
#4346=CARTESIAN_POINT ( 'NONE',  ( 2.109407804498405703, -9.207748739546751438, 2.396484790045401603 ) ) ;
#4352=CARTESIAN_POINT ( 'NONE',  ( 1.960495238260606010, -8.383787449798761671, 1.627490053312942164 ) ) ;
#4354=CARTESIAN_POINT ( 'NONE',  ( 13.09892531043291086, 3.683228176858501790, 6.000681092915118420 ) ) ;
#4359=CARTESIAN_POINT ( 'NONE',  ( 7.659691417683177406, -22.36352608949543352, 2.479004561291652031 ) ) ;
#4360=CARTESIAN_POINT ( 'NONE',  ( -13.10372118337080849, 3.925419760224517329, 6.005889426248455010 ) ) ;
#4361=CARTESIAN_POINT ( 'NONE',  ( -10.46530858231679595, -20.97900456129165647, 3.863526089495444626 ) ) ;
#4363=CARTESIAN_POINT ( 'NONE',  ( -10.47219141768317741, -24.47900456129165292, 2.413778621189595963 ) ) ;
#4365=CARTESIAN_POINT ( 'NONE',  ( 13.37500751150753864, -19.49962066887028556, 4.515663405036051792 ) ) ;
#4366=CARTESIAN_POINT ( 'NONE',  ( -12.65410809543883985, -18.78004118034163739, 5.517608176248461227 ) ) ;
#4370=CARTESIAN_POINT ( 'NONE',  ( 2.645259258103298983, -10.28229522185712241, 2.672449792925449596 ) ) ;
#4377=CARTESIAN_POINT ( 'NONE',  ( -0.5631383031621635116, -9.864917468222230923, 1.622643865078341907 ) ) ;
#4384=CARTESIAN_POINT ( 'NONE',  ( 4.847191417683177406, -20.91377862118959285, 1.020995438708345082 ) ) ;
#4385=CARTESIAN_POINT ( 'NONE',  ( -13.12529397353891270, 5.014845663890295846, 3.333333333333220239 ) ) ;
#4386=CARTESIAN_POINT ( 'NONE',  ( -7.753441417683176518, -21.94931252712233061, 1.749999999999998446 ) ) ;
#4390=CARTESIAN_POINT ( 'NONE',  ( 7.277808582316794173, -20.27099543870833642, 2.724438792969431589 ) ) ;
#4392=CARTESIAN_POINT ( 'NONE',  ( -13.37607268932110038, -20.94582918928111681, 4.945564004704174010 ) ) ;
#4393=CARTESIAN_POINT ( 'NONE',  ( 10.55905858231679595, -20.72672167713054137, 4.701595411283463477 ) ) ;
#4397=CARTESIAN_POINT ( 'NONE',  ( 13.40322194933353828, -19.57479155865495457, 6.214283636730510096 ) ) ;
#4402=CARTESIAN_POINT ( 'NONE',  ( -10.09030858231679595, -21.32581373872472597, 1.729004561291657582 ) ) ;
#4407=CARTESIAN_POINT ( 'NONE',  ( 1.819865260185086875, -9.122006307963404836, 1.624464420737683046 ) ) ;
#4409=CARTESIAN_POINT ( 'NONE',  ( -13.37930517931174634, -19.28258844475809042, 4.742233558278135419 ) ) ;
#4411=CARTESIAN_POINT ( 'NONE',  ( -13.42074492158312715, -18.68988146005270679, 6.255046935864005064 ) ) ;
#4412=CYLINDRICAL_SURFACE ( 'NONE', #19068, 0.3750000000000003331 ) ;
#4413=CARTESIAN_POINT ( 'NONE',  ( 11.49655858231679417, -22.05068747287764452, 1.749999999999998446 ) ) ;
#4416=CARTESIAN_POINT ( 'NONE',  ( 11.87844141768317741, -22.99999999999999645, 3.449312527122335048 ) ) ;
#4417=CARTESIAN_POINT ( 'NONE',  ( -12.53469141768317741, -20.22900456129164581, 2.825813738724748170 ) ) ;
#4418=VERTEX_POINT ( 'NONE', #15098 ) ;
#4419=CARTESIAN_POINT ( 'NONE',  ( 13.09494140422671471, 4.232040913449062636, 5.131376921800749003 ) ) ;
#4420=DIRECTION ( 'NONE',  ( 0.000000000000000000, 0.2487476929738665354, 0.9685683172808094987 ) ) ;
#4425=CARTESIAN_POINT ( 'NONE',  ( -12.62562019941893432, -20.21867992933967173, 4.757612834768309540 ) ) ;
#4428=CARTESIAN_POINT ( 'NONE',  ( -1.904508877737772998, -9.138371295333994837, 2.378667276417936627 ) ) ;
#4429=CARTESIAN_POINT ( 'NONE',  ( -13.87470602645761986, 4.985154336109792972, 4.666666666666619889 ) ) ;
#4432=CARTESIAN_POINT ( 'NONE',  ( -12.62500000000001954, -20.24999999999450040, 3.833333333368183382 ) ) ;
#4436=CARTESIAN_POINT ( 'NONE',  ( -10.93405858231679595, -23.73192549717337130, 5.303608408759367343 ) ) ;
#4437=CARTESIAN_POINT ( 'NONE',  ( -2.801385037117921861, -10.23463596792102415, 1.910209944425432349 ) ) ;
#4439=CARTESIAN_POINT ( 'NONE',  ( -13.38450946332969771, -19.76977210184853462, 5.359796180098093998 ) ) ;
#4443=CARTESIAN_POINT ( 'NONE',  ( 5.777808582316795949, -19.52099543870833642, 2.413778621189609286 ) ) ;
#4444=CARTESIAN_POINT ( 'NONE',  ( -13.18405858231679595, -21.32873467460644079, 2.757051763020455404 ) ) ;
#4446=CARTESIAN_POINT ( 'NONE',  ( 13.39782821820594627, -19.84717498059871943, 6.143582220458365661 ) ) ;
#4453=CARTESIAN_POINT ( 'NONE',  ( -13.40382044110196347, -18.79456772435387890, 5.502763032956559108 ) ) ;
#4454=CARTESIAN_POINT ( 'NONE',  ( 2.534747216115884161, -9.671180236796224960, 2.515503256513427210 ) ) ;
#4459=CARTESIAN_POINT ( 'NONE',  ( 2.887553741010006281, -10.84643174835951207, 2.067331322690557638 ) ) ;
#4461=CARTESIAN_POINT ( 'NONE',  ( 13.12529418130016445, 5.014856155665242454, 4.958178834604180629 ) ) ;
#4466=CARTESIAN_POINT ( 'NONE',  ( 5.690941417683177406, -22.74294823697955081, 4.171265325393542334 ) ) ;
#4467=CARTESIAN_POINT ( 'NONE',  ( -13.10756170493883310, 4.119366099410778581, 6.001761809183453700 ) ) ;
#4468=CARTESIAN_POINT ( 'NONE',  ( -8.965308582316795949, -20.97900456129165647, 3.863526089495444626 ) ) ;
#4470=CARTESIAN_POINT ( 'NONE',  ( -4.284691417683177406, -24.52099543870834708, 4.484846433055073689 ) ) ;
#4472=CARTESIAN_POINT ( 'NONE',  ( 13.09560264576187905, 4.265433610975056133, 4.791666666666684726 ) ) ;
#4478=CARTESIAN_POINT ( 'NONE',  ( 2.513306525444908512, -9.622685169956881168, 2.503048754562789746 ) ) ;
#4482=CARTESIAN_POINT ( 'NONE',  ( -1.548630333695928618, -9.864917468222230923, 1.622643865078341907 ) ) ;
#4486=CARTESIAN_POINT ( 'NONE',  ( 5.972191417683178294, -24.47900456129165292, 2.413778621189595963 ) ) ;
#4487=CARTESIAN_POINT ( 'NONE',  ( -11.69094141768317563, -23.27327832286946219, 4.701595411283453707 ) ) ;
#4489=CARTESIAN_POINT ( 'NONE',  ( 4.840308582316793284, -22.67418626127525982, 5.270995438708342640 ) ) ;
#4491=CARTESIAN_POINT ( 'NONE',  ( -12.66503773474750894, -18.97809439524806052, 6.263381662489337920 ) ) ;
#4494=CARTESIAN_POINT ( 'NONE',  ( 7.746558582316794173, -21.94931252712234482, 5.250000000000000888 ) ) ;
#4497=CARTESIAN_POINT ( 'NONE',  ( 13.85716935893578317, 3.349552626256921517, 6.729005269197402939 ) ) ;
#4504=CARTESIAN_POINT ( 'NONE',  ( -12.05905858231679417, -20.72672167713054137, 4.701595411283463477 ) ) ;
#4507=CARTESIAN_POINT ( 'NONE',  ( 3.049989092406311109, -8.938202327316346896, 1.769874869409437279 ) ) ;
#4509=CARTESIAN_POINT ( 'NONE',  ( -13.09560264575884503, 4.265433610975056133, 3.333333333333364568 ) ) ;
#4510=CARTESIAN_POINT ( 'NONE',  ( 5.777808582316794173, -20.27099543870833642, 2.724438792969431589 ) ) ;
#4511=CARTESIAN_POINT ( 'NONE',  ( -13.90439735423812273, 5.734566389025032684, 4.166666666666765551 ) ) ;
#4512=CARTESIAN_POINT ( 'NONE',  ( -13.87500000000000000, 5.000000000000049738, 4.000000000000000888 ) ) ;
#4513=CARTESIAN_POINT ( 'NONE',  ( 9.621558582316794173, -23.74999999999999645, 3.550687472877651629 ) ) ;
#4515=CARTESIAN_POINT ( 'NONE',  ( 13.09030858231679417, -21.63647391050454871, 2.479004561291657804 ) ) ;
#4516=CARTESIAN_POINT ( 'NONE',  ( -7.559058582316794173, -20.72672167713054137, 4.701595411283463477 ) ) ;
#4517=VERTEX_POINT ( 'NONE', #13831 ) ;
#4518=CARTESIAN_POINT ( 'NONE',  ( 13.37818000216760694, -19.33940989053615311, 4.728953261990445966 ) ) ;
#4519=CARTESIAN_POINT ( 'NONE',  ( -2.777355782919915139, -10.06396397089670458, 1.866377966073868411 ) ) ;
#4523=CARTESIAN_POINT ( 'NONE',  ( -12.62499999999998224, -20.25000000000006395, 4.416666666666681174 ) ) ;
#4525=CARTESIAN_POINT ( 'NONE',  ( -0.9854920305337622199, -8.364917468222230923, 2.372643865078341019 ) ) ;
#4526=CARTESIAN_POINT ( 'NONE',  ( -13.87470602645761986, 4.985154336109792972, 4.833333333333344584 ) ) ;
#4530=CARTESIAN_POINT ( 'NONE',  ( 11.49655858231679417, -22.05068747287764452, 1.749999999999998446 ) ) ;
#4532=CARTESIAN_POINT ( 'NONE',  ( 13.14123030749026277, 5.069630528265579805, 6.418963484850015000 ) ) ;
#4533=CARTESIAN_POINT ( 'NONE',  ( -12.62155858231679417, -24.50000000000000000, 3.550687472877651629 ) ) ;
#4534=CARTESIAN_POINT ( 'NONE',  ( -1.548630333695928618, -9.864917468222230923, 1.622643865078341907 ) ) ;
#4536=CARTESIAN_POINT ( 'NONE',  ( -13.83710853266996388, 3.836480899831821834, 5.239411421715695738 ) ) ;
#4538=CARTESIAN_POINT ( 'NONE',  ( 11.50344141768317741, -22.05068747287766229, 6.000000000000001776 ) ) ;
#4539=CARTESIAN_POINT ( 'NONE',  ( -11.59030858231679595, -21.63647391050454871, 2.479004561291657804 ) ) ;
#4542=CARTESIAN_POINT ( 'NONE',  ( 13.87454419214980739, 4.976981703567351367, 5.131312659523921127 ) ) ;
#4549=CARTESIAN_POINT ( 'NONE',  ( -13.41820805991576826, -18.06799297425606454, 5.518388032956592859 ) ) ;
#4553=CARTESIAN_POINT ( 'NONE',  ( 2.559937518207947793, -9.746075135043517079, 2.534737762559237773 ) ) ;
#4555=CARTESIAN_POINT ( 'NONE',  ( 1.619022621591186928, -8.364917468222230923, 1.622643865078341907 ) ) ;
#4557=CARTESIAN_POINT ( 'NONE',  ( 13.12529397354238192, 5.014845663890295846, 4.333333333333382775 ) ) ;
#4561=CARTESIAN_POINT ( 'NONE',  ( 7.472191417683177406, -22.97900456129165292, 3.035098964749240125 ) ) ;
#4562=CARTESIAN_POINT ( 'NONE',  ( -12.79798428357658047, -11.51429367935891790, 5.673858176248284479 ) ) ;
#4563=CARTESIAN_POINT ( 'NONE',  ( -8.590308582316797725, -21.63647391050454871, 2.479004561291657804 ) ) ;
#4564=CARTESIAN_POINT ( 'NONE',  ( -11.03469141768318273, -20.22900456129164581, 2.825813738724747726 ) ) ;
#4567=CARTESIAN_POINT ( 'NONE',  ( 13.09080647246885576, 4.023226859705822278, 5.257958009367514229 ) ) ;
#4571=ORIENTED_EDGE ( 'NONE', *, *, #8544, .F. ) ;
#4572=CARTESIAN_POINT ( 'NONE',  ( 1.732184490400474175, -9.869581059509965115, 2.373841568485653308 ) ) ;
#4574=CARTESIAN_POINT ( 'NONE',  ( 11.87844141768317563, -23.74999999999999645, 3.449312527122335492 ) ) ;
#4577=CARTESIAN_POINT ( 'NONE',  ( 0.000000000000000000, -9.114917468222230923, 1.622643865078341019 ) ) ;
#4581=CARTESIAN_POINT ( 'NONE',  ( 5.034691417683177406, -19.47900456129164581, 2.515153566944927199 ) ) ;
#4583=CARTESIAN_POINT ( 'NONE',  ( -12.62844141768317741, -20.24999999999999289, 3.550687472877664952 ) ) ;
#4585=CARTESIAN_POINT ( 'NONE',  ( 8.309058582316792396, -23.27327832286945153, 2.298404588716537411 ) ) ;
#4587=CARTESIAN_POINT ( 'NONE',  ( -12.70700162295422864, -16.85891804079483691, 6.308954579156044851 ) ) ;
#4595=CARTESIAN_POINT ( 'NONE',  ( -9.246558582316794173, -21.94931252712234482, 5.250000000000000888 ) ) ;
#4596=CARTESIAN_POINT ( 'NONE',  ( 12.62515553039088090, -20.24214571525854467, 4.629702272822510345 ) ) ;
#4598=CARTESIAN_POINT ( 'NONE',  ( 2.067263844777544435, -10.27417889452513933, 1.727750375171331676 ) ) ;
#4602=CARTESIAN_POINT ( 'NONE',  ( -13.38007464613909470, -19.24373036997283037, 4.743072998953621777 ) ) ;
#4603=CARTESIAN_POINT ( 'NONE',  ( 8.121558582316792396, -23.74999999999999645, 3.550687472877651629 ) ) ;
#4604=CARTESIAN_POINT ( 'NONE',  ( -12.64183575740756993, -20.14979425091403087, 6.022201559249563907 ) ) ;
#4606=CARTESIAN_POINT ( 'NONE',  ( 9.434058582316794173, -23.20159541128345992, 4.773278322869455970 ) ) ;
#4607=CARTESIAN_POINT ( 'NONE',  ( 6.065941417683177406, -22.67126532539353789, 2.757051763020445634 ) ) ;
#4608=CARTESIAN_POINT ( 'NONE',  ( -10.75344141768317741, -21.94931252712233061, 1.749999999999998446 ) ) ;
#4611=CARTESIAN_POINT ( 'NONE',  ( 13.09560264576187905, 4.265433610975056133, 2.999999999999999556 ) ) ;
#4612=CARTESIAN_POINT ( 'NONE',  ( -2.768424032093183662, -10.00067216410020166, 1.850123365707658785 ) ) ;
#4619=CARTESIAN_POINT ( 'NONE',  ( -3.317048600639548095, -9.800042196285016161, 2.741212564741740465 ) ) ;
#4620=CARTESIAN_POINT ( 'NONE',  ( -13.85403523778986390, 3.941279508358651817, 5.991705257707216958 ) ) ;
#4623=CARTESIAN_POINT ( 'NONE',  ( 2.747777887823422471, -9.906471667804277459, 1.825930796414880763 ) ) ;
#4625=CARTESIAN_POINT ( 'NONE',  ( 11.40280858231679595, -22.77556120703056308, 1.770995438708340197 ) ) ;
#4627=CARTESIAN_POINT ( 'NONE',  ( 13.11862022235054503, 3.927821228673052723, 6.755987001683414483 ) ) ;
#4628=CARTESIAN_POINT ( 'NONE',  ( -4.746558582316795061, -21.94931252712234127, 6.000000000000001776 ) ) ;
#4629=CARTESIAN_POINT ( 'NONE',  ( -1.716273078461125090, -9.866787073280026021, 2.373124017006284170 ) ) ;
#4633=CARTESIAN_POINT ( 'NONE',  ( -13.83411111208379474, 3.685111160228107252, 5.236156213382356484 ) ) ;
#4635=CARTESIAN_POINT ( 'NONE',  ( 4.097191417683177406, -23.08622137881040359, 5.979004561291654696 ) ) ;
#4636=CARTESIAN_POINT ( 'NONE',  ( -5.409691417683178294, -21.63647391050456648, 4.520995438708348857 ) ) ;
#4639=CARTESIAN_POINT ( 'NONE',  ( 13.40432071140796744, -19.51930407389869515, 6.223619713037471968 ) ) ;
#4651=CARTESIAN_POINT ( 'NONE',  ( 13.87500000000000000, 4.995017896875348917, 3.999999999999998224 ) ) ;
#4653=CARTESIAN_POINT ( 'NONE',  ( 2.780192134145684779, -10.08406280675441735, 1.871539748636713130 ) ) ;
#4658=CARTESIAN_POINT ( 'NONE',  ( -13.27780858231679595, -20.27099543870833642, 2.724438792969431589 ) ) ;
#4659=CARTESIAN_POINT ( 'NONE',  ( -2.567175533087980188, -9.771398394011347577, 2.541241281345096859 ) ) ;
#4661=CARTESIAN_POINT ( 'NONE',  ( 4.847191417683177406, -21.53509896474923835, 2.520995438708346192 ) ) ;
#4662=CARTESIAN_POINT ( 'NONE',  ( -12.62499999999998224, -19.49999999999998934, 4.166666666666637653 ) ) ;
#4663=CARTESIAN_POINT ( 'NONE',  ( -12.15280858231679950, -21.53509896474924901, 4.479004561291659137 ) ) ;
#4664=CARTESIAN_POINT ( 'NONE',  ( -6.159691417683175629, -22.98484643305507191, 0.9790045612916508100 ) ) ;
#4666=CARTESIAN_POINT ( 'NONE',  ( 13.09001666039658573, 3.983341349998239966, 5.257104358157307367 ) ) ;
#4672=CARTESIAN_POINT ( 'NONE',  ( 2.817596665886821672, -11.50588678273290988, 2.986692549455723267 ) ) ;
#4675=CARTESIAN_POINT ( 'NONE',  ( 9.534691417683177406, -20.22900456129164581, 2.825813738724748170 ) ) ;
#4679=CARTESIAN_POINT ( 'NONE',  ( -2.594671182134835163, -9.923034775318452461, 2.580184533305832861 ) ) ;
#4681=CARTESIAN_POINT ( 'NONE',  ( -9.902808582316794173, -22.77556120703056308, 1.770995438708340197 ) ) ;
#4684=CARTESIAN_POINT ( 'NONE',  ( 4.097191417683177406, -23.08622137881040359, 5.979004561291654696 ) ) ;
#4686=CARTESIAN_POINT ( 'NONE',  ( -11.59719141768317563, -22.77556120703057729, 5.229004561291655584 ) ) ;
#4687=( BOUNDED_CURVE ( )  B_SPLINE_CURVE ( 3, ( #1380, #15800, #1683, #17260 ),
 .UNSPECIFIED., .F., .T. ) 
 B_SPLINE_CURVE_WITH_KNOTS ( ( 4, 4 ),
 ( 0.5000000000000000000, 0.7500000000000000000 ),
 .UNSPECIFIED. ) 
 CURVE ( )  GEOMETRIC_REPRESENTATION_ITEM ( )  RATIONAL_B_SPLINE_CURVE ( ( 0.9667580569362952403, 0.6445053712908636045, 0.4833790284681485083, 0.4833790284681493410 ) ) 
 REPRESENTATION_ITEM ( '' )  );
#4689=CARTESIAN_POINT ( 'NONE',  ( 9.059058582316794173, -20.72672167713054137, 4.701595411283463477 ) ) ;
#4691=CARTESIAN_POINT ( 'NONE',  ( -12.62505438222622622, -20.99725369757571869, 4.613400783263607252 ) ) ;
#4702=CARTESIAN_POINT ( 'NONE',  ( -11.21530858231679595, -24.52099543870834708, 2.515153566944913432 ) ) ;
#4706=CARTESIAN_POINT ( 'NONE',  ( 1.337453470010121714, -9.114917468222230923, 1.622643865078341463 ) ) ;
#4711=CARTESIAN_POINT ( 'NONE',  ( -13.83531008031826026, 3.745659056069631898, 5.237458296715707284 ) ) ;
#4712=CARTESIAN_POINT ( 'NONE',  ( 13.27780858231679417, -19.52099543870833642, 2.413778621189609286 ) ) ;
#4713=CARTESIAN_POINT ( 'NONE',  ( -12.62499999999998224, -20.99999999999998934, 4.166666666666637653 ) ) ;
#4717=CARTESIAN_POINT ( 'NONE',  ( 4.472191417683178294, -22.97900456129165292, 3.035098964749240125 ) ) ;
#4718=CARTESIAN_POINT ( 'NONE',  ( -6.059058582316793284, -20.72672167713054137, 4.701595411283463477 ) ) ;
#4720=CARTESIAN_POINT ( 'NONE',  ( 13.09560260347216953, 4.265431475339161338, 5.020858537328734883 ) ) ;
#4727=CARTESIAN_POINT ( 'NONE',  ( -13.12270769621861355, 4.884238659038159902, 5.513847264053151065 ) ) ;
#4729=CARTESIAN_POINT ( 'NONE',  ( -3.607313482701580476, -10.70492285834919244, 2.223603995567122293 ) ) ;
#4731=CARTESIAN_POINT ( 'NONE',  ( 2.589709240944451096, -9.559844081062008669, 1.736909907557668165 ) ) ;
#4732=CARTESIAN_POINT ( 'NONE',  ( -12.64931222250080545, -19.02223276370786209, 5.512399842915133519 ) ) ;
#4733=CARTESIAN_POINT ( 'NONE',  ( 12.80905858231679417, -23.27327832286945153, 2.298404588716537411 ) ) ;
#4735=CARTESIAN_POINT ( 'NONE',  ( 13.15316049959406364, 5.672105229501871904, 5.573635960501007958 ) ) ;
#4738=CARTESIAN_POINT ( 'NONE',  ( -2.110348196723525138, -10.58007678474401914, 1.806311064303893099 ) ) ;
#4740=CARTESIAN_POINT ( 'NONE',  ( -13.87470602645761986, 4.985154336109792972, 4.833333333333344584 ) ) ;
#4742=CARTESIAN_POINT ( 'NONE',  ( 12.25344141768317741, -21.94931252712233061, 1.749999999999998446 ) ) ;
#4743=CARTESIAN_POINT ( 'NONE',  ( -5.034691417683177406, -20.97900456129164581, 3.136473910504570917 ) ) ;
#4745=CARTESIAN_POINT ( 'NONE',  ( 13.37671366598624800, -20.91345986769124465, 5.053911344471881506 ) ) ;
#4748=EDGE_LOOP ( 'NONE', ( #3561, #12688, #9884, #8177, #19560 ) ) ;
#4757=CARTESIAN_POINT ( 'NONE',  ( 2.579281110863027582, -9.822567596814183233, 2.554382554832406615 ) ) ;
#4759=CARTESIAN_POINT ( 'NONE',  ( 2.762374231067749708, -9.968169115173667549, 1.841775933429679268 ) ) ;
#4764=CARTESIAN_POINT ( 'NONE',  ( -12.99655858231679417, -22.05068747287764452, 1.749999999999998446 ) ) ;
#4765=CARTESIAN_POINT ( 'NONE',  ( -1.513434189748285696, -9.114917468222230923, 2.372643865078341019 ) ) ;
#4766=CARTESIAN_POINT ( 'NONE',  ( 13.37155858231679595, -20.99999999999999645, 3.449312527122348371 ) ) ;
#4767=CARTESIAN_POINT ( 'NONE',  ( -13.12503131243110843, 5.001581277770153378, 5.166347330538456184 ) ) ;
#4768=CARTESIAN_POINT ( 'NONE',  ( -11.87155858231679417, -20.24999999999999289, 3.449312527122348371 ) ) ;
#4770=CARTESIAN_POINT ( 'NONE',  ( -4.565941417683176518, -23.73192549717336064, 1.696391591240623331 ) ) ;
#4772=CARTESIAN_POINT ( 'NONE',  ( 13.08799567112409790, 3.881281391764801025, 5.254907606674271037 ) ) ;
#4781=DIRECTION ( 'NONE',  ( 0.000000000000000000, 0.2487476929738665354, 0.9685683172808094987 ) ) ;
#4784=CARTESIAN_POINT ( 'NONE',  ( -1.619022621591186928, -9.864917468222230923, 2.372643865078341019 ) ) ;
#4786=CARTESIAN_POINT ( 'NONE',  ( -12.71530858231679417, -23.77099543870833998, 2.825813738724734847 ) ) ;
#4789=CARTESIAN_POINT ( 'NONE',  ( 8.503441417683177406, -22.05068747287766229, 6.000000000000001776 ) ) ;
#4791=CARTESIAN_POINT ( 'NONE',  ( -5.409691417683178294, -21.32581373872474373, 5.270995438708348857 ) ) ;
#4794=ADVANCED_BREP_SHAPE_REPRESENTATION ( '', ( #11472, #18039 ), #12033 ) ;
#4795=CARTESIAN_POINT ( 'NONE',  ( 4.746558582316793284, -21.94931252712234482, 5.250000000000000888 ) ) ;
#4797=CARTESIAN_POINT ( 'NONE',  ( -12.66144083004408571, -19.15973808277258073, 6.259475412489329038 ) ) ;
#4799=CARTESIAN_POINT ( 'NONE',  ( 7.184058582316794173, -20.79840458871652942, 2.226721677130544030 ) ) ;
#4804=DIRECTION ( 'NONE',  ( 0.000000000000000000, -0.2487476929738665354, -0.9685683172808094987 ) ) ;
#4810=CARTESIAN_POINT ( 'NONE',  ( -6.434058582316794173, -23.20159541128345992, 4.773278322869455970 ) ) ;
#4811=CARTESIAN_POINT ( 'NONE',  ( 12.64511805349267526, -19.23403829861753422, 5.507852591554869726 ) ) ;
#4813=CARTESIAN_POINT ( 'NONE',  ( 1.733187991654075777, -9.867296153774269385, 1.623254759047128237 ) ) ;
#4815=( BOUNDED_CURVE ( )  B_SPLINE_CURVE ( 3, ( #4512, #17474, #7760, #14126 ),
 .UNSPECIFIED., .F., .T. ) 
 B_SPLINE_CURVE_WITH_KNOTS ( ( 4, 4 ),
 ( 0.001187255941418635012, 0.002344578398797381343 ),
 .UNSPECIFIED. ) 
 CURVE ( )  GEOMETRIC_REPRESENTATION_ITEM ( )  RATIONAL_B_SPLINE_CURVE ( ( 0.9619191252709787809, 0.3335846922424358096, 0.3462783171521095493, 1.000000000000000000 ) ) 
 REPRESENTATION_ITEM ( '' )  );
#4817=CARTESIAN_POINT ( 'NONE',  ( -13.42766088059286922, -16.84062553004338625, 4.794749963382423985 ) ) ;
#4818=CARTESIAN_POINT ( 'NONE',  ( 9.621558582316794173, -23.74999999999999645, 3.550687472877651629 ) ) ;
#4819=CARTESIAN_POINT ( 'NONE',  ( -13.88684657106908205, 4.848251838987907014, 6.535242036940271504 ) ) ;
#4821=CARTESIAN_POINT ( 'NONE',  ( -7.559058582316795949, -20.19639159124062999, 5.231925497173373074 ) ) ;
#4822=CARTESIAN_POINT ( 'NONE',  ( 7.371558582316794173, -20.24999999999999289, 3.449312527122348371 ) ) ;
#4823=CARTESIAN_POINT ( 'NONE',  ( 8.222191417683175629, -21.02099543870834353, 3.964901035250761208 ) ) ;
#4824=CARTESIAN_POINT ( 'NONE',  ( -8.222191417683175629, -20.27099543870833998, 4.275561207030583510 ) ) ;
#4826=CARTESIAN_POINT ( 'NONE',  ( 13.84402619238587206, 4.185822715484293077, 5.150938132831436533 ) ) ;
#4827=CARTESIAN_POINT ( 'NONE',  ( -2.708677329869237482, -9.785633270066144362, 1.794897081886200230 ) ) ;
#4833=CARTESIAN_POINT ( 'NONE',  ( -3.270401025279431995, -9.547343748290430199, 2.676314555138040063 ) ) ;
#4836=DIRECTION ( 'NONE',  ( 0.000000000000000000, -0.2487476929738665354, -0.9685683172808094987 ) ) ;
#4837=CARTESIAN_POINT ( 'NONE',  ( -12.83635126708105823, -9.576761012430582198, 5.715524842913705328 ) ) ;
#4838=CARTESIAN_POINT ( 'NONE',  ( 11.77780858231679773, -20.27099543870833642, 2.724438792969431589 ) ) ;
#4840=CARTESIAN_POINT ( 'NONE',  ( 13.15498530132288479, 5.764257716805535559, 3.666666666666500873 ) ) ;
#4841=CARTESIAN_POINT ( 'NONE',  ( -1.903957340438703572, -10.27085516675799148, 2.476896775482616331 ) ) ;
#4843=CARTESIAN_POINT ( 'NONE',  ( -13.39722611581222189, -19.12758115148224647, 5.495601574623241170 ) ) ;
#4845=CARTESIAN_POINT ( 'NONE',  ( 5.690941417683177406, -23.80360840875937001, 5.231925497173365081 ) ) ;
#4846=CARTESIAN_POINT ( 'NONE',  ( -12.90280858231679595, -22.46490103525074034, 2.520995438708341307 ) ) ;
#4848=CARTESIAN_POINT ( 'NONE',  ( 12.62500028073152869, -20.99998582305707728, 4.544498183892649479 ) ) ;
#4849=CARTESIAN_POINT ( 'NONE',  ( 12.62499999999998401, -19.49999999999998934, 3.146526952850934755 ) ) ;
#4858=CARTESIAN_POINT ( 'NONE',  ( 2.557403344953185442, -14.91030650174552896, 3.668400560659690779 ) ) ;
#4864=CARTESIAN_POINT ( 'NONE',  ( -12.90280858231679773, -22.77556120703056308, 1.770995438708339975 ) ) ;
#4865=CARTESIAN_POINT ( 'NONE',  ( -13.37327929115833491, -20.24999999560066399, 3.449077790995343840 ) ) ;
#4867=CARTESIAN_POINT ( 'NONE',  ( 10.09030858231679595, -21.63647391050454871, 2.479004561291657804 ) ) ;
#4868=CARTESIAN_POINT ( 'NONE',  ( -12.62562661273123332, -19.46835605706984040, 4.628101975944573176 ) ) ;
#4869=CARTESIAN_POINT ( 'NONE',  ( -5.777808582316795949, -21.02099543870833998, 3.035098964749253003 ) ) ;
#4870=CARTESIAN_POINT ( 'NONE',  ( -11.69094141768317563, -23.27327832286946219, 4.701595411283453707 ) ) ;
#4873=CARTESIAN_POINT ( 'NONE',  ( 13.81612658856640863, 2.776892722604777930, 5.216624963382545666 ) ) ;
#4876=ORIENTED_EDGE ( 'NONE', *, *, #16737, .F. ) ;
#4881=CARTESIAN_POINT ( 'NONE',  ( 9.065941417683177406, -23.20159541128344927, 2.226721677130534705 ) ) ;
#4883=CARTESIAN_POINT ( 'NONE',  ( -1.655860418491166941, -9.114909740826840689, 2.372641880528837621 ) ) ;
#4884=CARTESIAN_POINT ( 'NONE',  ( 2.602174906157317835, -9.976397331638239052, 2.593889103792902606 ) ) ;
#4887=CARTESIAN_POINT ( 'NONE',  ( 8.784691417683177406, -23.77099543870834353, 4.174186261275252718 ) ) ;
#4889=CARTESIAN_POINT ( 'NONE',  ( -11.78469141768317741, -23.02099543870834353, 3.863526089495429972 ) ) ;
#4891=CARTESIAN_POINT ( 'NONE',  ( 7.277808582316795061, -19.52099543870833642, 2.413778621189609286 ) ) ;
#4894=CARTESIAN_POINT ( 'NONE',  ( -12.62499999999998224, -21.00000000000006395, 4.416666666666682062 ) ) ;
#4906=CARTESIAN_POINT ( 'NONE',  ( -12.34030858231679773, -22.98484643305508612, 6.020995438708344416 ) ) ;
#4909=CARTESIAN_POINT ( 'NONE',  ( 1.963707630584672570, -9.980492102769451535, 1.652325740065381909 ) ) ;
#4911=CARTESIAN_POINT ( 'NONE',  ( 12.66369984131459070, -18.29565801360988075, 5.528024842915327142 ) ) ;
#4914=CARTESIAN_POINT ( 'NONE',  ( -13.79214722387705905, 1.565934805775630601, 5.190583296715636230 ) ) ;
#4915=CARTESIAN_POINT ( 'NONE',  ( 5.402808582316794173, -22.77556120703056308, 1.770995438708339975 ) ) ;
#4916=CARTESIAN_POINT ( 'NONE',  ( -12.66863463945108137, -18.79645070772368953, 6.267287912489321045 ) ) ;
#4918=CARTESIAN_POINT ( 'NONE',  ( -9.059058582316795949, -20.19639159124062999, 5.231925497173373074 ) ) ;
#4919=CARTESIAN_POINT ( 'NONE',  ( 4.934058582316793284, -23.20159541128345992, 4.773278322869455970 ) ) ;
#4920=CARTESIAN_POINT ( 'NONE',  ( 5.972191417683178294, -22.97900456129165292, 3.035098964749240125 ) ) ;
#4921=CARTESIAN_POINT ( 'NONE',  ( -6.347191417683176518, -21.22443879296941915, 1.770995438708345748 ) ) ;
#4924=CARTESIAN_POINT ( 'NONE',  ( 13.84501469867365131, 4.235742283194553259, 3.333333333332063386 ) ) ;
#4932=CARTESIAN_POINT ( 'NONE',  ( 13.37327929115833669, -20.24999999707183207, 3.449077790995325632 ) ) ;
#4933=CARTESIAN_POINT ( 'NONE',  ( -1.643076795806035717, -8.364903549957356077, 2.372640290589878909 ) ) ;
#4938=CARTESIAN_POINT ( 'NONE',  ( -12.62503117662529739, -20.24842558042254836, 4.565011198945062354 ) ) ;
#4941=CARTESIAN_POINT ( 'NONE',  ( 13.13728495444130751, 4.870390199291127153, 6.548325014280736767 ) ) ;
#4942=CARTESIAN_POINT ( 'NONE',  ( -1.776440835594205847, -9.874406767442327038, 1.625080906685880233 ) ) ;
#4944=CARTESIAN_POINT ( 'NONE',  ( -13.87470586348985258, 4.985146106231644225, 5.033049509202228933 ) ) ;
#4947=CARTESIAN_POINT ( 'NONE',  ( 4.378441417683176518, -24.50000000000000000, 3.449312527122335048 ) ) ;
#4948=CARTESIAN_POINT ( 'NONE',  ( -6.996558582316795949, -22.05068747287764452, 2.499999999999999112 ) ) ;
#4950=CARTESIAN_POINT ( 'NONE',  ( 12.63178515739782348, -20.65734955141111584, 5.567013446834313761 ) ) ;
#4951=CARTESIAN_POINT ( 'NONE',  ( 13.05696142222617695, 1.564051822406025583, 5.955108176248398166 ) ) ;
#4962=CARTESIAN_POINT ( 'NONE',  ( 1.872293763630120678, -10.04602735435188698, 2.419156501869924369 ) ) ;
#4965=CARTESIAN_POINT ( 'NONE',  ( -13.50000000000000178, 5.000000000000047962, 2.000000000000000000 ) ) ;
#4968=CARTESIAN_POINT ( 'NONE',  ( -12.90248710081030481, -20.62497818207526024, 3.513302565646801323 ) ) ;
#4970=CIRCLE ( 'NONE', #15639, 0.3749999999999997224 ) ;
#4971=CARTESIAN_POINT ( 'NONE',  ( -13.09533517714100093, 4.251926445620864747, 5.084080158857392284 ) ) ;
#4972=CARTESIAN_POINT ( 'NONE',  ( -6.152808582316795949, -21.53509896474924901, 4.479004561291659137 ) ) ;
#4973=CARTESIAN_POINT ( 'NONE',  ( -5.034691417683178294, -20.22900456129164581, 2.825813738724747726 ) ) ;
#4976=CARTESIAN_POINT ( 'NONE',  ( 13.45643611822145225, -15.38747602984844853, 4.825999963382285429 ) ) ;
#4986=CARTESIAN_POINT ( 'NONE',  ( 8.409691417683177406, -21.32581373872474373, 5.270995438708348857 ) ) ;
#4990=CARTESIAN_POINT ( 'NONE',  ( 2.513306525444908512, -9.622685169956881168, 2.503048754562789746 ) ) ;
#4993=CARTESIAN_POINT ( 'NONE',  ( 7.940941417683176518, -20.72672167713052715, 2.298404588716546293 ) ) ;
#4995=CARTESIAN_POINT ( 'NONE',  ( -10.37844141768317741, -22.99999999999999645, 3.449312527122335048 ) ) ;
#4997=CARTESIAN_POINT ( 'NONE',  ( 9.809058582316795949, -23.80360840875935935, 1.768074502826626260 ) ) ;
#4998=CARTESIAN_POINT ( 'NONE',  ( 12.62888984277510218, -20.05356293986039873, 5.111704976569332537 ) ) ;
#4999=CARTESIAN_POINT ( 'NONE',  ( -13.12405442816082868, 4.202248622120948518, 6.747400073346936367 ) ) ;
#5010=CARTESIAN_POINT ( 'NONE',  ( 13.28675616151867267, -20.00825975431586912, 3.460912183795370023 ) ) ;
#5012=CARTESIAN_POINT ( 'NONE',  ( -7.090308582316794173, -21.32581373872472597, 1.729004561291657582 ) ) ;
#5015=CARTESIAN_POINT ( 'NONE',  ( 1.513434189748285918, -9.864917468222230923, 1.622643865078341907 ) ) ;
#5017=CARTESIAN_POINT ( 'NONE',  ( 13.08094078691552831, 2.775009739235173356, 5.981149842915306714 ) ) ;
#5019=CARTESIAN_POINT ( 'NONE',  ( -13.84501469867711698, 4.235742283194553259, 4.583333333333295734 ) ) ;
#5020=CARTESIAN_POINT ( 'NONE',  ( 12.99655858231679595, -22.05068747287764452, 0.9999999999999978906 ) ) ;
#5021=CARTESIAN_POINT ( 'NONE',  ( -13.15316049959406364, 5.672105229501871904, 5.573635960501007958 ) ) ;
#5022=CARTESIAN_POINT ( 'NONE',  ( -12.62844141768317741, -19.49999999999998934, 3.550687472877664952 ) ) ;
#5025=CARTESIAN_POINT ( 'NONE',  ( 4.315753587183822404, -21.47141115243053378, 5.558207674221720573 ) ) ;
#5026=CARTESIAN_POINT ( 'NONE',  ( 9.527808582316795949, -22.97900456129165647, 3.964901035250747885 ) ) ;
#5027=CARTESIAN_POINT ( 'NONE',  ( -5.597191417683177406, -22.77556120703057729, 5.229004561291656472 ) ) ;
#5030=CARTESIAN_POINT ( 'NONE',  ( 13.37503071710846925, -20.24844878602346299, 4.564052989354591361 ) ) ;
#5042=CARTESIAN_POINT ( 'NONE',  ( -13.11145189917479392, 4.315820908324673688, 5.961432613039677086 ) ) ;
#5045=CARTESIAN_POINT ( 'NONE',  ( -2.801385037117921861, -10.23463596792102415, 1.910209944425432349 ) ) ;
#5047=CARTESIAN_POINT ( 'NONE',  ( -13.12463908936614132, 4.981774012991869505, 5.264611377988129171 ) ) ;
#5050=CARTESIAN_POINT ( 'NONE',  ( 12.64195242771744709, -19.39390240027112000, 5.496549442168085164 ) ) ;
#5052=CARTESIAN_POINT ( 'NONE',  ( -1.513434189748285918, -9.864917468222230923, 2.372643865078341019 ) ) ;
#5054=CARTESIAN_POINT ( 'NONE',  ( -13.44218742460511073, -16.85703505742523234, 5.544429699623282914 ) ) ;
#5057=CARTESIAN_POINT ( 'NONE',  ( 6.628441417683177406, -19.49999999999998934, 3.550687472877664952 ) ) ;
#5058=CARTESIAN_POINT ( 'NONE',  ( -5.402808582316795949, -22.46490103525074034, 2.520995438708341307 ) ) ;
#5060=CARTESIAN_POINT ( 'NONE',  ( 13.90439735423812273, 5.734566389025032684, 4.666666666666618113 ) ) ;
#5061=CARTESIAN_POINT ( 'NONE',  ( 12.65410809543883985, -18.78004118034163739, 5.517608176248461227 ) ) ;
#5071=CARTESIAN_POINT ( 'NONE',  ( 13.87470602645761808, 4.985154336109792972, 4.000000000000000000 ) ) ;
#5072=CARTESIAN_POINT ( 'NONE',  ( 1.407845757905374695, -9.864917468222230923, 1.622643865078341907 ) ) ;
#5075=ADVANCED_FACE ( 'NONE', ( #9117 ), #19799, .F. ) ;
#5079=CARTESIAN_POINT ( 'NONE',  ( -2.616536356806028696, -10.07836329504444706, 2.620076000170431296 ) ) ;
#5081=CARTESIAN_POINT ( 'NONE',  ( -13.09001666039658573, 3.983341349998239966, 5.257104358157307367 ) ) ;
#5082=CARTESIAN_POINT ( 'NONE',  ( -4.746558582316795061, -21.94931252712234127, 4.499999999999999112 ) ) ;
#5083=CARTESIAN_POINT ( 'NONE',  ( -10.00344141768317563, -22.05068747287765873, 5.250000000000000888 ) ) ;
#5085=CARTESIAN_POINT ( 'NONE',  ( 13.84501465882535598, 4.235740270674679842, 5.020612255068622076 ) ) ;
#5094=CARTESIAN_POINT ( 'NONE',  ( 5.128441417683177406, -20.24999999999999289, 3.550687472877664952 ) ) ;
#5096=CARTESIAN_POINT ( 'NONE',  ( -1.837882866761050282, -9.938290523052360825, 2.391487531332776140 ) ) ;
#5098=CARTESIAN_POINT ( 'NONE',  ( -10.74655858231679417, -21.94931252712234482, 5.250000000000000888 ) ) ;
#5102=CARTESIAN_POINT ( 'NONE',  ( 6.722191417683177406, -20.27099543870833998, 4.275561207030583510 ) ) ;
#5104=CARTESIAN_POINT ( 'NONE',  ( -11.22219141768317741, -21.02099543870834353, 3.964901035250761208 ) ) ;
#5106=CARTESIAN_POINT ( 'NONE',  ( 11.21530858231679595, -24.52099543870834708, 2.515153566944913432 ) ) ;
#5107=CARTESIAN_POINT ( 'NONE',  ( 12.66369984131459070, -18.29565801360988075, 5.528024842915327142 ) ) ;
#5108=CARTESIAN_POINT ( 'NONE',  ( -13.12519991495504712, 4.260095705229160146, 6.739971950528219402 ) ) ;
#5118=CARTESIAN_POINT ( 'NONE',  ( -11.49655858231679595, -22.05068747287764452, 0.9999999999999978906 ) ) ;
#5119=CARTESIAN_POINT ( 'NONE',  ( 13.09293046926041626, 3.380488697651010011, 5.994170676248444352 ) ) ;
#5122=CARTESIAN_POINT ( 'NONE',  ( 12.83635126708105823, -9.576761012430582198, 5.715524842913705328 ) ) ;
#5124=CARTESIAN_POINT ( 'NONE',  ( -13.38449802415168932, -19.02034978033825396, 4.747874963382372471 ) ) ;
#5125=CARTESIAN_POINT ( 'NONE',  ( 12.62155858231679417, -24.50000000000000000, 3.550687472877651629 ) ) ;
#5126=CARTESIAN_POINT ( 'NONE',  ( -12.75496035233418013, -14.43700220713569138, 6.361037912489419632 ) ) ;
#5127=CARTESIAN_POINT ( 'NONE',  ( -11.69094141768317741, -23.80360840875937001, 5.231925497173365081 ) ) ;
#5131=CARTESIAN_POINT ( 'NONE',  ( 11.96530858231679773, -20.97900456129165647, 3.863526089495444626 ) ) ;
#5132=CARTESIAN_POINT ( 'NONE',  ( -5.784691417683177406, -23.77099543870834353, 4.174186261275251830 ) ) ;
#5136=CARTESIAN_POINT ( 'NONE',  ( 13.38450946332969771, -19.76977210184853462, 5.359796180098093998 ) ) ;
#5143=CARTESIAN_POINT ( 'NONE',  ( 13.77789853026076550, 0.09637577819625635367, 5.909013032956687006 ) ) ;
#5145=CARTESIAN_POINT ( 'NONE',  ( 2.602174906157317835, -9.976397331638239052, 2.593889103792902606 ) ) ;
#5147=CARTESIAN_POINT ( 'NONE',  ( -12.64195242771744709, -19.39390240027112000, 5.496549442168085164 ) ) ;
#5148=CARTESIAN_POINT ( 'NONE',  ( 5.777808582316794173, -20.27099543870833642, 2.724438792969431589 ) ) ;
#5150=CARTESIAN_POINT ( 'NONE',  ( 13.12463908936614132, 4.981774012991869505, 5.264611377988129171 ) ) ;
#5151=EDGE_CURVE ( 'NONE', #6462, #18369, #10444, .T. ) ;
#5152=CARTESIAN_POINT ( 'NONE',  ( -1.957016269584227031, -9.152392576945766578, 2.382268221639079364 ) ) ;
#5153=CARTESIAN_POINT ( 'NONE',  ( -13.87444723674697755, 4.972085455720938185, 5.163895512850782410 ) ) ;
#5155=CARTESIAN_POINT ( 'NONE',  ( 11.97219141768317563, -23.72900456129165292, 2.724438792969417822 ) ) ;
#5156=CARTESIAN_POINT ( 'NONE',  ( -8.215308582316795949, -23.02099543870833998, 3.136473910504556262 ) ) ;
#5158=CARTESIAN_POINT ( 'NONE',  ( 13.90326467458556969, 5.677366066573198644, 5.457668599364335904 ) ) ;
#5159=CARTESIAN_POINT ( 'NONE',  ( 13.12529397354238192, 5.014845663890295846, 4.791666666666685614 ) ) ;
#5167=CARTESIAN_POINT ( 'NONE',  ( 1.337453470010121714, -9.114917468222230923, 1.622643865078341463 ) ) ;
#5171=CARTESIAN_POINT ( 'NONE',  ( 12.73094043006643616, -20.51123272440521816, 3.536703532973982433 ) ) ;
#5173=CARTESIAN_POINT ( 'NONE',  ( -8.777808582316792396, -20.27099543870833642, 2.724438792969431589 ) ) ;
#5175=CARTESIAN_POINT ( 'NONE',  ( -3.336296098497695262, -9.936854405034125648, 2.776348673047012383 ) ) ;
#5177=CARTESIAN_POINT ( 'NONE',  ( -12.62500004114794372, -19.49999792202770621, 4.520295319612473328 ) ) ;
#5178=CARTESIAN_POINT ( 'NONE',  ( -12.05905858231679417, -20.72672167713054137, 4.701595411283463477 ) ) ;
#5179=B_SPLINE_CURVE_WITH_KNOTS ( 'NONE', 3,
 ( #17883, #8569, #16310, #6592, #11807, #419 ),
 .UNSPECIFIED., .F., .F.,
 ( 4, 2, 4 ),
 ( 0.000000000000000000, 0.5000000000000000000, 1.000000000000000000 ),
 .UNSPECIFIED. ) ;
#5180=CARTESIAN_POINT ( 'NONE',  ( -6.253441417683176518, -21.94931252712233061, 1.749999999999998446 ) ) ;
#5182=CARTESIAN_POINT ( 'NONE',  ( 13.83531008031826026, 3.745659056069631898, 5.237458296715707284 ) ) ;
#5200=CARTESIAN_POINT ( 'NONE',  ( 8.503441417683177406, -22.05068747287765873, 5.250000000000000888 ) ) ;
#5202=CARTESIAN_POINT ( 'NONE',  ( -9.815941417683177406, -21.32873467460645145, 4.242948236979555254 ) ) ;
#5204=CARTESIAN_POINT ( 'NONE',  ( 11.96530858231679773, -19.47900456129164937, 4.484846433055089676 ) ) ;
#5205=CARTESIAN_POINT ( 'NONE',  ( 13.00900269284621302, -0.8578640112522492034, 5.903024842915844062 ) ) ;
#5206=CARTESIAN_POINT ( 'NONE',  ( -13.15047398821051239, 5.536436404627260721, 5.896317606305554015 ) ) ;
#5213=CARTESIAN_POINT ( 'NONE',  ( 13.36733061693429292, -20.15943224161095770, 3.450097756028646323 ) ) ;
#5216=CARTESIAN_POINT ( 'NONE',  ( 13.02818618459764188, 0.1109023222084986743, 5.923858176248589125 ) ) ;
#5219=CARTESIAN_POINT ( 'NONE',  ( 13.15498530132288479, 5.764257716805535559, 4.583333333333295734 ) ) ;
#5221=CARTESIAN_POINT ( 'NONE',  ( -13.37561105820882013, -20.21914156045197686, 4.753815841436231260 ) ) ;
#5222=CARTESIAN_POINT ( 'NONE',  ( 8.496558582316795949, -22.05068747287764452, 0.9999999999999978906 ) ) ;
#5223=CARTESIAN_POINT ( 'NONE',  ( -13.13084019862132479, 4.544930030374419339, 6.677052771569639944 ) ) ;
#5224=CARTESIAN_POINT ( 'NONE',  ( -6.809058582316796837, -23.80360840875935935, 1.768074502826626260 ) ) ;
#5226=CARTESIAN_POINT ( 'NONE',  ( 3.944195004867014909, -21.56714562517547051, 5.389209506672564487 ) ) ;
#5228=CARTESIAN_POINT ( 'NONE',  ( 8.684058582316795949, -21.32873467460644079, 2.757051763020455404 ) ) ;
#5229=CARTESIAN_POINT ( 'NONE',  ( -5.503441417683176518, -22.05068747287765873, 5.250000000000000888 ) ) ;
#5231=EDGE_LOOP ( 'NONE', ( #2530, #15186, #6629, #10491, #4571 ) ) ;
#5232=CARTESIAN_POINT ( 'NONE',  ( 13.87470602645761986, 4.985154336109792972, 3.666666666666500873 ) ) ;
#5240=CARTESIAN_POINT ( 'NONE',  ( 13.38800411018677572, -19.59329243556743805, 5.436267741224407146 ) ) ;
#5242=CARTESIAN_POINT ( 'NONE',  ( 1.904508877737772998, -9.138371295333994837, 2.378667276417936627 ) ) ;
#5243=CARTESIAN_POINT ( 'NONE',  ( 0.5631383031621635116, -9.114917468222230923, 1.622643865078341463 ) ) ;
#5244=CARTESIAN_POINT ( 'NONE',  ( -12.72590726430969532, -14.40418315237199742, 4.861678440007700885 ) ) ;
#5245=CARTESIAN_POINT ( 'NONE',  ( 7.465308582316795061, -20.22900456129164937, 4.174186261275266929 ) ) ;
#5247=CARTESIAN_POINT ( 'NONE',  ( 12.79798428357658047, -11.51429367935891790, 5.673858176248284479 ) ) ;
#5248=CARTESIAN_POINT ( 'NONE',  ( -1.655860418491166941, -9.114909740826840689, 2.372641880528837621 ) ) ;
#5249=CARTESIAN_POINT ( 'NONE',  ( 8.496558582316795949, -22.05068747287764452, 2.499999999999999112 ) ) ;
#5251=CARTESIAN_POINT ( 'NONE',  ( 11.03469141768318273, -20.22900456129164581, 2.825813738724747726 ) ) ;
#5252=CARTESIAN_POINT ( 'NONE',  ( -5.496558582316795949, -22.05068747287764452, 2.499999999999999112 ) ) ;
#5254=CARTESIAN_POINT ( 'NONE',  ( 13.84517967659089521, 2.744073667841084418, 6.715984435864265301 ) ) ;
#5255=CARTESIAN_POINT ( 'NONE',  ( 13.12529380813666435, 5.014837310896125722, 5.033295791462342628 ) ) ;
#5262=CARTESIAN_POINT ( 'NONE',  ( -13.50000000000000178, 5.000000000000047962, 4.000000000000000000 ) ) ;
#5265=CARTESIAN_POINT ( 'NONE',  ( -2.693754455098655409, -10.14181605509423711, 1.874202551270839123 ) ) ;
#5266=CARTESIAN_POINT ( 'NONE',  ( 0.9854920305337622199, -9.864917468222230923, 1.622643865078341907 ) ) ;
#5274=CARTESIAN_POINT ( 'NONE',  ( -9.434058582316794173, -23.20159541128345992, 4.773278322869455970 ) ) ;
#5275=CARTESIAN_POINT ( 'NONE',  ( -3.779650890485476200, -11.92851441922421607, 2.537846752097290715 ) ) ;
#5277=CARTESIAN_POINT ( 'NONE',  ( -12.93692567357942202, -3.747753484270499591, 5.090845106672844622 ) ) ;
#5278=CARTESIAN_POINT ( 'NONE',  ( -9.715308582316794173, -23.77099543870833998, 2.825813738724734847 ) ) ;
#5279=CARTESIAN_POINT ( 'NONE',  ( -9.722191417683177406, -20.27099543870833998, 4.275561207030583510 ) ) ;
#5281=CARTESIAN_POINT ( 'NONE',  ( 13.47561960997282071, -14.41870969638424071, 4.846833296715798767 ) ) ;
#5282=( NAMED_UNIT ( * ) PLANE_ANGLE_UNIT ( ) SI_UNIT ( $, .RADIAN. ) );
#5286=ORIENTED_EDGE ( 'NONE', *, *, #2791, .F. ) ;
#5290=CARTESIAN_POINT ( 'NONE',  ( 6.628441417683176518, -20.24999999999999289, 3.550687472877664952 ) ) ;
#5295=CARTESIAN_POINT ( 'NONE',  ( -5.402808582316794173, -22.77556120703056308, 1.770995438708340197 ) ) ;
#5299=CARTESIAN_POINT ( 'NONE',  ( 12.06594141768317563, -23.20159541128344927, 2.226721677130534705 ) ) ;
#5302=CARTESIAN_POINT ( 'NONE',  ( -5.597191417683177406, -22.46490103525075810, 4.479004561291653808 ) ) ;
#5303=CARTESIAN_POINT ( 'NONE',  ( -9.434058582316795949, -23.73192549717337130, 5.303608408759367343 ) ) ;
#5305=CARTESIAN_POINT ( 'NONE',  ( 12.74043380832193684, -14.42059267975384529, 5.611358176248560703 ) ) ;
#5306=CARTESIAN_POINT ( 'NONE',  ( -12.62599079447150885, -20.19996487918709249, 4.820256282269618886 ) ) ;
#5320=ORIENTED_EDGE ( 'NONE', *, *, #15642, .F. ) ;
#5322=CARTESIAN_POINT ( 'NONE',  ( 13.12526104302547836, 5.013182672784613381, 5.066812735559260261 ) ) ;
#5325=CARTESIAN_POINT ( 'NONE',  ( 12.62499999999998579, -20.24999999999999289, 3.146526952850934755 ) ) ;
#5328=CARTESIAN_POINT ( 'NONE',  ( 7.465308582316796837, -19.47900456129164937, 4.484846433055089676 ) ) ;
#5329=CARTESIAN_POINT ( 'NONE',  ( -13.15498530132288479, 5.764257716805535559, 4.833333333333343695 ) ) ;
#5331=CARTESIAN_POINT ( 'NONE',  ( -7.277808582316795061, -19.52099543870833642, 2.413778621189609286 ) ) ;
#5336=CARTESIAN_POINT ( 'NONE',  ( 11.87155858231679595, -20.99999999999999645, 3.449312527122348371 ) ) ;
#5340=CARTESIAN_POINT ( 'NONE',  ( 13.87470602645415063, 4.985154336109792972, 3.333333333332063830 ) ) ;
#5346=CARTESIAN_POINT ( 'NONE',  ( 13.87470602645761808, 4.985154336109792972, 4.000000000000000000 ) ) ;
#5347=CARTESIAN_POINT ( 'NONE',  ( 13.85343352903393388, 3.910893216212274925, 5.991044282956552891 ) ) ;
#5350=CARTESIAN_POINT ( 'NONE',  ( 0.000000000000000000, -9.114917468222230923, 2.372643865078340575 ) ) ;
#5352=CARTESIAN_POINT ( 'NONE',  ( 1.819865260185086875, -9.122006307963404836, 1.624464420737683046 ) ) ;
#5353=CARTESIAN_POINT ( 'NONE',  ( -13.04243487821393721, 1.580461349787872782, 5.205428440007538349 ) ) ;
#5354=CARTESIAN_POINT ( 'NONE',  ( 7.277808582316795061, -20.27099543870833642, 2.724438792969431589 ) ) ;
#5356=CARTESIAN_POINT ( 'NONE',  ( 12.65051119073526564, -18.96168486786632457, 5.513701926248478102 ) ) ;
#5358=CARTESIAN_POINT ( 'NONE',  ( -2.623717082130370137, -10.12934627674766830, 2.633169448359191644 ) ) ;
#5359=CARTESIAN_POINT ( 'NONE',  ( 12.15280858231679950, -21.53509896474924901, 4.479004561291659137 ) ) ;
#5360=CARTESIAN_POINT ( 'NONE',  ( 10.75344141768317741, -21.94931252712233061, 1.749999999999998446 ) ) ;
#5361=CARTESIAN_POINT ( 'NONE',  ( -9.059058582316795949, -21.25705176302045274, 4.171265325393551215 ) ) ;
#5363=CARTESIAN_POINT ( 'NONE',  ( 13.11465082267961968, 3.727366545318180791, 6.751662912489328150 ) ) ;
#5364=CARTESIAN_POINT ( 'NONE',  ( 13.09206359972826661, 4.086711786274932479, 5.245812454509717782 ) ) ;
#5375=CARTESIAN_POINT ( 'NONE',  ( 2.367358971471363649, -9.400572650371021410, 2.446005822389718087 ) ) ;
#5381=CARTESIAN_POINT ( 'NONE',  ( -9.996558582316794173, -22.05068747287764452, 1.749999999999998446 ) ) ;
#5383=CARTESIAN_POINT ( 'NONE',  ( -3.722205087890566144, -11.52065056559861134, 2.433099166587254558 ) ) ;
#5385=CARTESIAN_POINT ( 'NONE',  ( -13.74418849449709512, -0.8559810278826442964, 5.138499963383082125 ) ) ;
#5386=CARTESIAN_POINT ( 'NONE',  ( -8.496558582316794173, -22.05068747287764452, 1.749999999999998446 ) ) ;
#5388=CARTESIAN_POINT ( 'NONE',  ( -6.909691417683177406, -21.32581373872474373, 5.270995438708348857 ) ) ;
#5390=CARTESIAN_POINT ( 'NONE',  ( 13.38800411018677572, -19.59329243556743805, 5.436267741224407146 ) ) ;
#5397=EDGE_CURVE ( 'NONE', #19275, #4418, #5541, .T. ) ;
#5404=CARTESIAN_POINT ( 'NONE',  ( 1.717920576997000737, -9.114924032904250240, 2.372645551019823884 ) ) ;
#5405=CARTESIAN_POINT ( 'NONE',  ( -8.590308582316794173, -21.32581373872472952, 1.729004561291657138 ) ) ;
#5406=CARTESIAN_POINT ( 'NONE',  ( 13.90439735423812273, 5.734566389025032684, 4.583333333333295734 ) ) ;
#5408=CARTESIAN_POINT ( 'NONE',  ( 11.31594141768317741, -21.32873467460645145, 4.242948236979555254 ) ) ;
#5409=CARTESIAN_POINT ( 'NONE',  ( -12.62499999999998224, -20.24999999999998934, 4.166666666666636765 ) ) ;
#5410=CARTESIAN_POINT ( 'NONE',  ( -8.503441417683177406, -22.05068747287766229, 4.499999999999999112 ) ) ;
#5413=CARTESIAN_POINT ( 'NONE',  ( -9.152808582316795949, -20.91377862118960351, 5.979004561291660913 ) ) ;
#5415=CARTESIAN_POINT ( 'NONE',  ( 13.10012427866737639, 3.743776072700027324, 6.001983176248468332 ) ) ;
#5416=CARTESIAN_POINT ( 'NONE',  ( -12.62888984277510218, -20.05356293986039873, 5.111704976569332537 ) ) ;
#5429=CARTESIAN_POINT ( 'NONE',  ( 13.12270769621861355, 4.884238659038159902, 5.513847264053151065 ) ) ;
#5430=CARTESIAN_POINT ( 'NONE',  ( -3.049989092406311109, -8.938202327316346896, 1.769874869409437279 ) ) ;
#5433=CARTESIAN_POINT ( 'NONE',  ( 13.09532840572934376, 3.501584489333809724, 5.996774842915142401 ) ) ;
#5435=CARTESIAN_POINT ( 'NONE',  ( 10.74655858231679595, -21.94931252712234127, 6.000000000000001776 ) ) ;
#5436=CARTESIAN_POINT ( 'NONE',  ( -13.15498530131898214, 5.764257716805535559, 3.333333333333075466 ) ) ;
#5437=CARTESIAN_POINT ( 'NONE',  ( -5.034691417683177406, -19.47900456129164581, 2.515153566944927199 ) ) ;
#5444=CARTESIAN_POINT ( 'NONE',  ( 7.559058582316795949, -21.25705176302045274, 4.171265325393551215 ) ) ;
#5448=CARTESIAN_POINT ( 'NONE',  ( 13.43259567872942917, -17.34141822415733714, 5.534013032956523581 ) ) ;
#5455=CARTESIAN_POINT ( 'NONE',  ( 13.70116456325478893, -3.778689555664588973, 5.825679699621801433 ) ) ;
#5457=CARTESIAN_POINT ( 'NONE',  ( 3.257364212367626966, -9.501732542047829355, 2.664600686199549706 ) ) ;
#5459=CARTESIAN_POINT ( 'NONE',  ( 1.720709671993384093, -9.114925383610804843, 1.622645897908254753 ) ) ;
#5460=CARTESIAN_POINT ( 'NONE',  ( -12.63118877378512828, -19.18746692385052555, 4.758813856674282583 ) ) ;
#5463=CARTESIAN_POINT ( 'NONE',  ( 12.74043380832193684, -14.42059267975384529, 5.611358176248560703 ) ) ;
#5464=CARTESIAN_POINT ( 'NONE',  ( -1.824488249492779879, -9.124319963227819130, 2.375058613629473570 ) ) ;
#5465=CARTESIAN_POINT ( 'NONE',  ( 9.996558582316795949, -22.05068747287764452, 2.499999999999999112 ) ) ;
#5466=CARTESIAN_POINT ( 'NONE',  ( 9.159691417683179182, -22.67418626127524917, 1.729004561291651809 ) ) ;
#5467=CARTESIAN_POINT ( 'NONE',  ( -9.996558582316794173, -22.05068747287764452, 1.749999999999998446 ) ) ;
#5469=CARTESIAN_POINT ( 'NONE',  ( 13.14782865898149034, 5.402847278557675104, 6.092770214907355708 ) ) ;
#5470=CARTESIAN_POINT ( 'NONE',  ( 12.70672377255832686, -15.37294948583620346, 4.840845106674187548 ) ) ;
#5472=ORIENTED_EDGE ( 'NONE', *, *, #9240, .F. ) ;
#5479=CARTESIAN_POINT ( 'NONE',  ( 2.203959450683124377, -9.262433282444222371, 2.410528873095051594 ) ) ;
#5482=CARTESIAN_POINT ( 'NONE',  ( 13.06507523707239038, -20.62500821465549095, 3.491123088105135608 ) ) ;
#5484=CARTESIAN_POINT ( 'NONE',  ( -10.09030858231679595, -21.32581373872472597, 1.729004561291657582 ) ) ;
#5485=CARTESIAN_POINT ( 'NONE',  ( 0.000000000000000000, -9.114917468222230923, 2.372643865078340575 ) ) ;
#5487=CARTESIAN_POINT ( 'NONE',  ( -13.37499999999998224, -19.50000000000006040, 4.416666666666682062 ) ) ;
#5488=CARTESIAN_POINT ( 'NONE',  ( -8.215308582316792396, -23.77099543870833998, 2.825813738724734847 ) ) ;
#5489=CARTESIAN_POINT ( 'NONE',  ( -10.47219141768317741, -22.97900456129165292, 3.035098964749240125 ) ) ;
#5491=CARTESIAN_POINT ( 'NONE',  ( 13.58606361274418184, -9.591287556442823714, 5.700679699621803209 ) ) ;
#5497=CARTESIAN_POINT ( 'NONE',  ( -13.38450946332969771, -19.76977210184853462, 5.359796180098093998 ) ) ;
#5500=DIRECTION ( 'NONE',  ( 0.1351665943404306014, -0.9596796555888912339, 0.2464649070825229438 ) ) ;
#5503=CARTESIAN_POINT ( 'NONE',  ( 3.257364212367626966, -9.501732542047829355, 2.664600686199549706 ) ) ;
#5504=CARTESIAN_POINT ( 'NONE',  ( -6.715308582316794173, -23.77099543870833998, 2.825813738724734847 ) ) ;
#5505=CARTESIAN_POINT ( 'NONE',  ( 13.90439735423812273, 5.734566389025032684, 4.916666666666649199 ) ) ;
#5510=CARTESIAN_POINT ( 'NONE',  ( 9.347191417683177406, -21.53509896474923835, 2.520995438708346192 ) ) ;
#5511=CARTESIAN_POINT ( 'NONE',  ( -12.62499999999998401, -20.24999999999998934, 2.439580858552613751 ) ) ;
#5512=CARTESIAN_POINT ( 'NONE',  ( -8.784691417683177406, -23.02099543870834353, 3.863526089495429972 ) ) ;
#5513=CARTESIAN_POINT ( 'NONE',  ( -10.46530858231679595, -19.47900456129164937, 4.484846433055089676 ) ) ;
#5515=CARTESIAN_POINT ( 'NONE',  ( 13.12119116326504908, 4.807653744879115010, 5.626470997801169105 ) ) ;
#5516=CARTESIAN_POINT ( 'NONE',  ( -12.66849571425264287, -18.05346643024382303, 5.533233176248494978 ) ) ;
#5526=DIRECTION ( 'NONE',  ( -0.000000000000000000, -0.000000000000000000, -1.000000000000000000 ) ) ;
#5527=CARTESIAN_POINT ( 'NONE',  ( 12.65410809543883985, -18.78004118034163739, 5.517608176248461227 ) ) ;
#5529=CARTESIAN_POINT ( 'NONE',  ( -1.337453470010121714, -8.364917468222230923, 1.622643865078341907 ) ) ;
#5532=CARTESIAN_POINT ( 'NONE',  ( 13.12529397354238192, 5.014845663890295846, 4.916666666666650087 ) ) ;
#5536=CARTESIAN_POINT ( 'NONE',  ( 5.590308582316795949, -21.01515356694490322, 0.9790045612916562501 ) ) ;
#5537=CARTESIAN_POINT ( 'NONE',  ( -12.95145221759166354, -3.764163011652346569, 5.840524842913703552 ) ) ;
#5538=CARTESIAN_POINT ( 'NONE',  ( -4.097191417683177406, -23.08622137881040359, 5.979004561291654696 ) ) ;
#5541=LINE ( 'NONE', #934, #10420 ) ;
#5542=CARTESIAN_POINT ( 'NONE',  ( -13.83079205777725917, 2.017498917744843023, 6.700359435863729729 ) ) ;
#5543=CARTESIAN_POINT ( 'NONE',  ( 6.434058582316796837, -22.67126532539354855, 4.242948236979545484 ) ) ;
#5547=CARTESIAN_POINT ( 'NONE',  ( 13.80667376788930056, 1.549525278393783179, 5.940263032956496048 ) ) ;
#5554=CARTESIAN_POINT ( 'NONE',  ( 13.37499999999998757, -20.24999999999999289, 3.482947684955674639 ) ) ;
#5557=CARTESIAN_POINT ( 'NONE',  ( 3.343476823822036259, -9.987837386737346890, 2.789442121235767402 ) ) ;
#5559=CARTESIAN_POINT ( 'NONE',  ( -12.62515856830665584, -19.49199230051052822, 4.565864671500353467 ) ) ;
#5561=CARTESIAN_POINT ( 'NONE',  ( 11.96530858231679595, -20.22900456129164937, 4.174186261275266929 ) ) ;
#5562=CARTESIAN_POINT ( 'NONE',  ( -13.45671396861735403, -16.87344458480707843, 6.294109435864141844 ) ) ;
#5564=CARTESIAN_POINT ( 'NONE',  ( 12.71530858231679417, -23.02099543870833998, 3.136473910504556262 ) ) ;
#5566=CARTESIAN_POINT ( 'NONE',  ( 6.347191417683176518, -21.22443879296941915, 1.770995438708345748 ) ) ;
#5567=CARTESIAN_POINT ( 'NONE',  ( -10.74655858231679417, -21.94931252712234482, 5.250000000000000888 ) ) ;
#5569=CARTESIAN_POINT ( 'NONE',  ( 13.12405442816082868, 4.202248622120948518, 6.747400073346936367 ) ) ;
#5570=CARTESIAN_POINT ( 'NONE',  ( 13.05202662408965075, 2.064844516520778939, 5.215845106673912213 ) ) ;
#5581=CARTESIAN_POINT ( 'NONE',  ( 1.337453470010121714, -9.114917468222230923, 2.372643865078341019 ) ) ;
#5585=CARTESIAN_POINT ( 'NONE',  ( 12.66022036808238305, -20.41063448930580648, 3.546131378954796798 ) ) ;
#5587=CARTESIAN_POINT ( 'NONE',  ( -5.215308582316793284, -23.77099543870833998, 2.825813738724734847 ) ) ;
#5588=CARTESIAN_POINT ( 'NONE',  ( -3.385922596301560894, -9.481287983549590237, 1.909350115156127403 ) ) ;
#5590=CARTESIAN_POINT ( 'NONE',  ( -13.37499994994395891, -19.50000252782794519, 4.474109982178703149 ) ) ;
#5591=CARTESIAN_POINT ( 'NONE',  ( -4.687312169500632564, -21.51559725698341197, 5.182386163300427562 ) ) ;
#5593=CARTESIAN_POINT ( 'NONE',  ( 9.996558582316795949, -22.05068747287764452, 0.9999999999999978906 ) ) ;
#5594=CARTESIAN_POINT ( 'NONE',  ( -12.34719141768317741, -21.53509896474923835, 2.520995438708346192 ) ) ;
#5596=CARTESIAN_POINT ( 'NONE',  ( 13.85223456079946303, 3.850345320370711644, 5.989742199623227847 ) ) ;
#5602=CARTESIAN_POINT ( 'NONE',  ( -13.37524505148396514, -20.23762490005974968, 4.659512268729234741 ) ) ;
#5608=CARTESIAN_POINT ( 'NONE',  ( 3.767139617958116471, -12.99583330722436791, 3.561955564372631500 ) ) ;
#5609=CARTESIAN_POINT ( 'NONE',  ( -5.309058582316794173, -23.27327832286945153, 2.298404588716537411 ) ) ;
#5610=CARTESIAN_POINT ( 'NONE',  ( 12.62499999999998224, -21.00000000000006395, 4.416666666666682062 ) ) ;
#5612=CARTESIAN_POINT ( 'NONE',  ( 11.78469141768317741, -23.02099543870834353, 3.863526089495429972 ) ) ;
#5613=CARTESIAN_POINT ( 'NONE',  ( -12.62499999999998579, -20.24999999999999289, 3.146526952850934755 ) ) ;
#5614=CARTESIAN_POINT ( 'NONE',  ( -5.128441417683177406, -20.99999999999999645, 3.550687472877664952 ) ) ;
#5616=CARTESIAN_POINT ( 'NONE',  ( -12.62844141768317741, -19.49999999999998934, 3.550687472877664952 ) ) ;
#5619=CARTESIAN_POINT ( 'NONE',  ( 12.67794853492974561, -16.82609898603114118, 4.809595106674325216 ) ) ;
#5620=CARTESIAN_POINT ( 'NONE',  ( -12.65650603190776025, -18.65894538865861563, 5.520212342915047365 ) ) ;
#5632=CARTESIAN_POINT ( 'NONE',  ( -3.451003380014874722, -9.682417022083358304, 1.961004070207825523 ) ) ;
#5637=FACE_OUTER_BOUND ( 'NONE', #13589, .T. ) ;
#5638=CARTESIAN_POINT ( 'NONE',  ( 6.715308582316796837, -24.52099543870834708, 2.515153566944913432 ) ) ;
#5639=CARTESIAN_POINT ( 'NONE',  ( -13.11740841389447709, 4.616624901677048420, 5.813473370769506765 ) ) ;
#5640=CARTESIAN_POINT ( 'NONE',  ( -6.347191417683176518, -20.91377862118959285, 1.020995438708345082 ) ) ;
#5641=ORIENTED_EDGE ( 'NONE', *, *, #18837, .T. ) ;
#5642=CARTESIAN_POINT ( 'NONE',  ( 11.59030858231679417, -21.32581373872472597, 1.729004561291657582 ) ) ;
#5644=CARTESIAN_POINT ( 'NONE',  ( -13.44712222274167246, -17.35782775154002522, 6.283692769197384287 ) ) ;
#5647=CARTESIAN_POINT ( 'NONE',  ( 11.77780858231679417, -20.27099543870833642, 2.724438792969431589 ) ) ;
#5652=CARTESIAN_POINT ( 'NONE',  ( 13.75871503850933841, -0.8723905552644914962, 5.888179699623941943 ) ) ;
#5664=CARTESIAN_POINT ( 'NONE',  ( 1.407845757905374695, -9.114917468222230923, 2.372643865078341019 ) ) ;
#5667=CARTESIAN_POINT ( 'NONE',  ( -12.63958155142659834, -18.76363165295958524, 4.767928440007602298 ) ) ;
#5669=CARTESIAN_POINT ( 'NONE',  ( 11.02780858231679595, -23.72900456129165647, 4.275561207030568411 ) ) ;
#5670=CARTESIAN_POINT ( 'NONE',  ( -13.39995901559228031, -19.73956971259024229, 6.178279423016713956 ) ) ;
#5672=CARTESIAN_POINT ( 'NONE',  ( 13.37155858231679417, -20.24999999999999289, 3.449312527122348371 ) ) ;
#5674=CARTESIAN_POINT ( 'NONE',  ( 12.06594141768317741, -22.67126532539353789, 2.757051763020445634 ) ) ;
#5675=CARTESIAN_POINT ( 'NONE',  ( -13.09030858231679417, -21.32581373872472597, 1.729004561291657582 ) ) ;
#5677=CARTESIAN_POINT ( 'NONE',  ( 12.81251082758882376, -11.53070320674076576, 6.423537912489145185 ) ) ;
#5678=CARTESIAN_POINT ( 'NONE',  ( 12.62503976493681535, -19.49799187068907713, 4.533161381885315144 ) ) ;
#5685=CYLINDRICAL_SURFACE ( 'NONE', #12904, 0.3750000000000003331 ) ;
#5689=CARTESIAN_POINT ( 'NONE',  ( 0.000000000000000000, -9.114917468222230923, 2.372643865078340575 ) ) ;
#5693=CARTESIAN_POINT ( 'NONE',  ( -0.2815691515810352930, -9.114917468222230923, 2.372643865078523984 ) ) ;
#5694=CARTESIAN_POINT ( 'NONE',  ( -9.340308582316795949, -22.98484643305508612, 6.020995438708344416 ) ) ;
#5695=CARTESIAN_POINT ( 'NONE',  ( -1.513434189748285696, -9.114917468222230923, 1.622643865078341463 ) ) ;
#5698=CARTESIAN_POINT ( 'NONE',  ( -13.37499999999998401, -19.49999999999998934, 2.439580858552613751 ) ) ;
#5699=CARTESIAN_POINT ( 'NONE',  ( -7.371558582316794173, -20.24999999999999289, 3.449312527122348371 ) ) ;
#5702=CARTESIAN_POINT ( 'NONE',  ( 9.347191417683177406, -20.91377862118959285, 1.020995438708345082 ) ) ;
#5703=CARTESIAN_POINT ( 'NONE',  ( -8.409691417683177406, -21.63647391050456648, 4.520995438708348857 ) ) ;
#5706=CARTESIAN_POINT ( 'NONE',  ( 13.37561105820882013, -20.21914156045197686, 4.753815841436231260 ) ) ;
#5712=CARTESIAN_POINT ( 'NONE',  ( -13.49014615398506045, -14.43511922376608680, 5.596513032956658584 ) ) ;
#5721=CARTESIAN_POINT ( 'NONE',  ( 1.643076795806035717, -8.364903549957356077, 2.372640290589878909 ) ) ;
#5723=CARTESIAN_POINT ( 'NONE',  ( 13.87372783958217681, 4.185755898898970706, 6.732634959205082481 ) ) ;
#5727=CARTESIAN_POINT ( 'NONE',  ( 4.003441417683176518, -22.05068747287765873, 5.250000000000000888 ) ) ;
#5728=CARTESIAN_POINT ( 'NONE',  ( -12.62599079447150885, -20.19996487918709249, 4.820256282269618886 ) ) ;
#5729=CARTESIAN_POINT ( 'NONE',  ( -9.534691417683177406, -20.97900456129164581, 3.136473910504570917 ) ) ;
#5730=CIRCLE ( 'NONE', #10417, 0.3749999999999997224 ) ;
#5731=CARTESIAN_POINT ( 'NONE',  ( -8.690941417683177406, -23.80360840875937001, 5.231925497173365081 ) ) ;
#5733=CARTESIAN_POINT ( 'NONE',  ( 12.62500000000002132, -19.49999999999450040, 3.833333333368183382 ) ) ;
#5734=CARTESIAN_POINT ( 'NONE',  ( -12.68288333306630378, -17.32689168014509207, 5.548858176248425700 ) ) ;
#5745=CARTESIAN_POINT ( 'NONE',  ( -1.513434189748285696, -9.114917468222230923, 1.622643865078341463 ) ) ;
#5750=CARTESIAN_POINT ( 'NONE',  ( 12.34719141768317741, -20.91377862118959285, 1.020995438708345082 ) ) ;
#5751=CARTESIAN_POINT ( 'NONE',  ( -13.10557919622060652, 4.019249409169220577, 6.007898877577752650 ) ) ;
#5752=CARTESIAN_POINT ( 'NONE',  ( -8.128441417683177406, -19.49999999999998934, 3.550687472877664952 ) ) ;
#5756=CARTESIAN_POINT ( 'NONE',  ( -13.39995901559228031, -19.73956971259024229, 6.178279423016713956 ) ) ;
#5757=CARTESIAN_POINT ( 'NONE',  ( 10.65280858231679240, -21.22443879296942626, 5.229004561291659137 ) ) ;
#5761=CARTESIAN_POINT ( 'NONE',  ( 13.37526900345969771, -20.98641532528209908, 4.724331462949078464 ) ) ;
#5767=CARTESIAN_POINT ( 'NONE',  ( -9.715308582316794173, -23.77099543870833998, 2.825813738724734847 ) ) ;
#5770=CARTESIAN_POINT ( 'NONE',  ( 2.830107938415192148, -10.43856789473369950, 1.962583737180462418 ) ) ;
#5771=ADVANCED_FACE ( 'NONE', ( #11080 ), #3892, .F. ) ;
#5773=CARTESIAN_POINT ( 'NONE',  ( -13.09560264576187905, 4.265433610975056133, 4.333333333333380999 ) ) ;
#5775=CARTESIAN_POINT ( 'NONE',  ( -13.41175265982446696, -19.14399067886409256, 6.245281310864100988 ) ) ;
#5778=CARTESIAN_POINT ( 'NONE',  ( 6.059058582316795949, -21.25705176302045274, 4.171265325393551215 ) ) ;
#5780=CARTESIAN_POINT ( 'NONE',  ( 12.34719141768317741, -21.53509896474923835, 2.520995438708346192 ) ) ;
#5781=CARTESIAN_POINT ( 'NONE',  ( -12.15280858231679595, -21.22443879296942626, 5.229004561291659137 ) ) ;
#5783=CARTESIAN_POINT ( 'NONE',  ( 13.09080647246885576, 4.023226859705822278, 5.257958009367514229 ) ) ;
#5789=CARTESIAN_POINT ( 'NONE',  ( -12.72125031657057015, -15.38935901321805133, 5.590524842915047365 ) ) ;
#5790=CARTESIAN_POINT ( 'NONE',  ( -2.659620708751979645, -10.38426118526329489, 2.698636689302993830 ) ) ;
#5791=CARTESIAN_POINT ( 'NONE',  ( -13.85980676119184629, 4.232741440188380722, 5.965367510457697975 ) ) ;
#5797=CARTESIAN_POINT ( 'NONE',  ( -1.407845757905374695, -9.114917468222230923, 2.372643865078341019 ) ) ;
#5798=CARTESIAN_POINT ( 'NONE',  ( -12.15280858231679950, -20.91377862118960351, 5.979004561291660913 ) ) ;
#5799=CARTESIAN_POINT ( 'NONE',  ( -2.682825141213236009, -9.727160171598653093, 1.779880022082258373 ) ) ;
#5801=CARTESIAN_POINT ( 'NONE',  ( -13.38449802415168932, -19.02034978033825396, 4.747874963382372471 ) ) ;
#5803=CARTESIAN_POINT ( 'NONE',  ( 11.78469141768317741, -24.52099543870834708, 4.484846433055073689 ) ) ;
#5804=CARTESIAN_POINT ( 'NONE',  ( -12.06594141768317741, -22.67126532539353789, 2.757051763020445634 ) ) ;
#5806=CARTESIAN_POINT ( 'NONE',  ( 13.47096266223369376, -15.40388555723029462, 5.575679699623145247 ) ) ;
#5813=CARTESIAN_POINT ( 'NONE',  ( -13.41341218697771609, -18.31018455762212227, 5.513179699623425023 ) ) ;
#5815=CARTESIAN_POINT ( 'NONE',  ( 2.559937518207947793, -9.746075135043517079, 2.534737762559237773 ) ) ;
#5822=CARTESIAN_POINT ( 'NONE',  ( 0.000000000000000000, -8.364917468222230923, 2.372643865078341019 ) ) ;
#5824=CARTESIAN_POINT ( 'NONE',  ( 12.66503773474750894, -18.97809439524806052, 6.263381662489337920 ) ) ;
#5828=CARTESIAN_POINT ( 'NONE',  ( 10.94094141768317741, -21.25705176302044208, 2.828734674606458555 ) ) ;
#5830=CARTESIAN_POINT ( 'NONE',  ( -11.02780858231679595, -22.97900456129165647, 3.964901035250747885 ) ) ;
#5831=CARTESIAN_POINT ( 'NONE',  ( -8.409691417683177406, -21.01515356694492098, 6.020995438708349745 ) ) ;
#5833=CARTESIAN_POINT ( 'NONE',  ( 12.62499999999998224, -19.50000000000006040, 4.416666666666682062 ) ) ;
#5834=CARTESIAN_POINT ( 'NONE',  ( -13.10012427866737639, 3.743776072700027324, 6.001983176248468332 ) ) ;
#5840=CARTESIAN_POINT ( 'NONE',  ( 2.623717082130370137, -10.12934627674766830, 2.633169448359191644 ) ) ;
#5842=ORIENTED_EDGE ( 'NONE', *, *, #1216, .T. ) ;
#5847=CARTESIAN_POINT ( 'NONE',  ( -2.340131407102140848, -12.21153219924485889, 2.225301406344140531 ) ) ;
#5851=CARTESIAN_POINT ( 'NONE',  ( 11.59719141768317741, -23.08622137881040359, 5.979004561291654696 ) ) ;
#5852=CARTESIAN_POINT ( 'NONE',  ( -13.10821839766814279, 4.152529082241303904, 5.997503362667785609 ) ) ;
#5853=CARTESIAN_POINT ( 'NONE',  ( -8.690941417683177406, -23.80360840875937001, 5.231925497173365081 ) ) ;
#5855=CARTESIAN_POINT ( 'NONE',  ( 12.52780858231679595, -23.72900456129165647, 4.275561207030568411 ) ) ;
#5857=CARTESIAN_POINT ( 'NONE',  ( -13.38172782443493602, -20.66024486603417643, 5.557997437521964734 ) ) ;
#5859=CARTESIAN_POINT ( 'NONE',  ( 11.12155858231679417, -23.74999999999999645, 3.550687472877651629 ) ) ;
#5863=CARTESIAN_POINT ( 'NONE',  ( 13.37499999999998401, -20.99999999999999645, 3.146526952850934755 ) ) ;
#5865=ORIENTED_EDGE ( 'NONE', *, *, #8911, .F. ) ;
#5868=CARTESIAN_POINT ( 'NONE',  ( -10.84030858231679240, -22.67418626127525982, 5.270995438708342640 ) ) ;
#5870=CARTESIAN_POINT ( 'NONE',  ( 13.12529397354238192, 5.014845663890297622, 3.999999999999981792 ) ) ;
#5871=CARTESIAN_POINT ( 'NONE',  ( 2.226467333542268445, -8.440126719678968215, 1.641959103308203716 ) ) ;
#5873=CARTESIAN_POINT ( 'NONE',  ( -13.09560264576187905, 4.265433610975056133, 4.666666666666618113 ) ) ;
#5876=CARTESIAN_POINT ( 'NONE',  ( -13.83079205777725917, 2.017498917744843023, 6.700359435863729729 ) ) ;
#5878=CARTESIAN_POINT ( 'NONE',  ( 12.99655858231679417, -22.05068747287764452, 1.749999999999998446 ) ) ;
#5879=CARTESIAN_POINT ( 'NONE',  ( 10.19094141768317741, -22.74294823697955081, 4.171265325393542334 ) ) ;
#5880=CARTESIAN_POINT ( 'NONE',  ( -12.34030858231679240, -22.67418626127525982, 5.270995438708342640 ) ) ;
#5882=CARTESIAN_POINT ( 'NONE',  ( 13.09560264576187905, 4.265433610975056133, 4.833333333333343695 ) ) ;
#5888=CARTESIAN_POINT ( 'NONE',  ( -13.09293046926041626, 3.380488697651010011, 5.994170676248444352 ) ) ;
#5889=CARTESIAN_POINT ( 'NONE',  ( -2.567175533087980188, -9.771398394011347577, 2.541241281345096859 ) ) ;
#5890=CARTESIAN_POINT ( 'NONE',  ( -13.39359219590679295, -19.31109410670777038, 5.491647114909025795 ) ) ;
#5896=CARTESIAN_POINT ( 'NONE',  ( -9.809058582316795949, -23.80360840875935935, 1.768074502826626260 ) ) ;
#5897=CARTESIAN_POINT ( 'NONE',  ( -2.916276642307554123, -11.05036367517186058, 2.119705115445599475 ) ) ;
#5899=CARTESIAN_POINT ( 'NONE',  ( -13.83890698502169059, 3.927302743594121903, 5.241364546715693074 ) ) ;
#5901=CARTESIAN_POINT ( 'NONE',  ( 11.69094141768317741, -23.80360840875937001, 5.231925497173365081 ) ) ;
#5902=CARTESIAN_POINT ( 'NONE',  ( -7.565941417683177406, -22.67126532539353789, 2.757051763020445634 ) ) ;
#5904=CARTESIAN_POINT ( 'NONE',  ( 13.40787921250184311, -19.33959976865745389, 6.241060671539915283 ) ) ;
#5911=CARTESIAN_POINT ( 'NONE',  ( -13.87467358130843387, 4.983515856073828409, 5.065827972856573602 ) ) ;
#5919=CARTESIAN_POINT ( 'NONE',  ( 2.532303758294933704, -8.551221675625164664, 1.670490507339845054 ) ) ;
#5925=CARTESIAN_POINT ( 'NONE',  ( 6.159691417683175629, -22.36352608949543352, 2.479004561291652031 ) ) ;
#5926=CARTESIAN_POINT ( 'NONE',  ( -13.11017182064853159, 4.251176942750957366, 5.979809059808775196 ) ) ;
#5927=CARTESIAN_POINT ( 'NONE',  ( -7.652808582316796837, -21.53509896474924901, 4.479004561291659137 ) ) ;
#5928=CARTESIAN_POINT ( 'NONE',  ( -7.565941417683177406, -23.73192549717336064, 1.696391591240623331 ) ) ;
#5930=CARTESIAN_POINT ( 'NONE',  ( 13.12463908936614132, 4.981774012991869505, 5.264611377988129171 ) ) ;
#5931=CARTESIAN_POINT ( 'NONE',  ( -13.11017182064853159, 4.251176942750957366, 5.979809059808775196 ) ) ;
#5936=ORIENTED_EDGE ( 'NONE', *, *, #11266, .T. ) ;
#5937=CARTESIAN_POINT ( 'NONE',  ( 1.866357130655357688, -10.00562759449716133, 2.408781036472938730 ) ) ;
#5941=CARTESIAN_POINT ( 'NONE',  ( -2.124709647372160060, -10.68204274815009924, 1.832497960681391147 ) ) ;
#5946=CARTESIAN_POINT ( 'NONE',  ( 11.22219141768317741, -19.52099543870834353, 4.586221378810406257 ) ) ;
#5947=CARTESIAN_POINT ( 'NONE',  ( -13.12503131243110843, 5.001581277770153378, 5.166347330538456184 ) ) ;
#5948=CARTESIAN_POINT ( 'NONE',  ( -8.034691417683175629, -20.22900456129164581, 2.825813738724747726 ) ) ;
#5950=CARTESIAN_POINT ( 'NONE',  ( 10.93405858231679417, -23.20159541128345992, 4.773278322869455970 ) ) ;
#5952=CARTESIAN_POINT ( 'NONE',  ( -13.37543017851028893, -20.97827598523083026, 4.780017688621249761 ) ) ;
#5954=CARTESIAN_POINT ( 'NONE',  ( 5.777808582316795949, -21.02099543870833998, 3.035098964749253003 ) ) ;
#5956=DIRECTION ( 'NONE',  ( 1.000000000000000000, 0.000000000000000000, 0.000000000000000000 ) ) ;
#5960=CARTESIAN_POINT ( 'NONE',  ( 13.40957725085194241, -19.25384883197511243, 6.242932005802575901 ) ) ;
#5967=CARTESIAN_POINT ( 'NONE',  ( -11.21530858231679417, -23.77099543870833998, 2.825813738724734847 ) ) ;
#5971=CARTESIAN_POINT ( 'NONE',  ( 3.232228556578340850, -13.29361487011126464, 2.695816835751057461 ) ) ;
#5973=CARTESIAN_POINT ( 'NONE',  ( -13.09560264576187905, 4.265433610975056133, 2.999999999999999556 ) ) ;
#5976=CARTESIAN_POINT ( 'NONE',  ( 10.93405858231679417, -23.20159541128345992, 4.773278322869455970 ) ) ;
#5977=CARTESIAN_POINT ( 'NONE',  ( -13.37499999998404299, -20.99999999996810729, 2.793053905886972998 ) ) ;
#5980=CARTESIAN_POINT ( 'NONE',  ( 12.34030858231679240, -22.67418626127525982, 5.270995438708342640 ) ) ;
#5981=CARTESIAN_POINT ( 'NONE',  ( 4.565941417683176518, -23.20159541128344927, 2.226721677130534705 ) ) ;
#5982=CARTESIAN_POINT ( 'NONE',  ( -5.590308582316794173, -21.32581373872472597, 1.729004561291657582 ) ) ;
#5984=CARTESIAN_POINT ( 'NONE',  ( 13.09543520949579865, 4.256978079540234106, 5.067654010725516578 ) ) ;
#5985=CARTESIAN_POINT ( 'NONE',  ( -0.9854920305337621089, -9.114917468222230923, 1.622643865078341463 ) ) ;
#5991=CARTESIAN_POINT ( 'NONE',  ( -12.63943061533661982, -19.52125392549825733, 5.470334935344855154 ) ) ;
#5993=CARTESIAN_POINT ( 'NONE',  ( -2.109407804498405703, -9.207748739546751438, 2.396484790045401603 ) ) ;
#5994=CARTESIAN_POINT ( 'NONE',  ( -13.87406079471522347, 4.952570133121557028, 5.260711232101737522 ) ) ;
#6000=CARTESIAN_POINT ( 'NONE',  ( -1.126276606324276619, -9.114917468222230923, 2.372643865078341019 ) ) ;
#6001=CARTESIAN_POINT ( 'NONE',  ( -7.840308582316795949, -22.98484643305508612, 6.020995438708344416 ) ) ;
#6002=CARTESIAN_POINT ( 'NONE',  ( -2.627360420079438263, -14.25085146736906339, 2.749039333894452763 ) ) ;
#6004=CARTESIAN_POINT ( 'NONE',  ( -13.84485691484488257, 4.227774199669918964, 5.063753864839139140 ) ) ;
#6006=CARTESIAN_POINT ( 'NONE',  ( 11.03469141768317741, -19.47900456129164581, 2.515153566944927199 ) ) ;
#6007=CARTESIAN_POINT ( 'NONE',  ( -13.09030858231679417, -21.63647391050454871, 2.479004561291657804 ) ) ;
#6010=CARTESIAN_POINT ( 'NONE',  ( 13.86693669322925260, 4.592803008081209448, 5.801483467520450077 ) ) ;
#6022=CARTESIAN_POINT ( 'NONE',  ( 3.277163086644854229, -14.76879761173520578, 3.824673233536266537 ) ) ;
#6026=CARTESIAN_POINT ( 'NONE',  ( 1.852280067228949445, -9.126254559850970338, 1.625555456689752321 ) ) ;
#6028=CARTESIAN_POINT ( 'NONE',  ( 13.11145189917479392, 4.315820908324673688, 5.961432613039677086 ) ) ;
#6034=CARTESIAN_POINT ( 'NONE',  ( 13.18405858231679595, -21.32873467460644079, 2.757051763020455404 ) ) ;
#6035=CARTESIAN_POINT ( 'NONE',  ( -13.10624331898488037, 4.052787608736739600, 6.006964772046813117 ) ) ;
#6036=CARTESIAN_POINT ( 'NONE',  ( -8.027808582316795949, -22.97900456129165647, 3.964901035250747885 ) ) ;
#6037=CARTESIAN_POINT ( 'NONE',  ( -5.222191417683177406, -19.52099543870834353, 4.586221378810406257 ) ) ;
#6040=CARTESIAN_POINT ( 'NONE',  ( 13.06641424290328501, 2.791419266617020334, 5.231470106674447784 ) ) ;
#6043=EDGE_CURVE ( 'NONE', #8463, #6462, #6227, .T. ) ;
#6045=SHAPE_REPRESENTATION ( 'spring', ( #18039 ), #12033 ) ;
#6047=CARTESIAN_POINT ( 'NONE',  ( 2.594671182134835163, -9.923034775318452461, 2.580184533305832861 ) ) ;
#6054=CARTESIAN_POINT ( 'NONE',  ( -1.665360951492234287, -9.864914341757378580, 1.622643062139706993 ) ) ;
#6056=DIRECTION ( 'NONE',  ( 0.000000000000000000, 0.2487476929738665354, 0.9685683172808094987 ) ) ;
#6059=CARTESIAN_POINT ( 'NONE',  ( 4.190941417683176518, -23.80360840875937001, 5.231925497173365081 ) ) ;
#6061=CARTESIAN_POINT ( 'NONE',  ( -11.97219141768317563, -23.72900456129165292, 2.724438792969417822 ) ) ;
#6064=CARTESIAN_POINT ( 'NONE',  ( 10.09030858231679595, -21.32581373872472597, 1.729004561291657582 ) ) ;
#6066=CARTESIAN_POINT ( 'NONE',  ( -12.66204031416134335, -19.12946413485185104, 6.260126454156002218 ) ) ;
#6068=CARTESIAN_POINT ( 'NONE',  ( 4.840308582316793284, -22.67418626127525982, 5.270995438708342640 ) ) ;
#6070=ORIENTED_EDGE ( 'NONE', *, *, #17734, .F. ) ;
#6072=CARTESIAN_POINT ( 'NONE',  ( 13.37499999999998224, -20.99999999999998934, 4.291666666666699825 ) ) ;
#6078=CARTESIAN_POINT ( 'NONE',  ( -9.434058582316794173, -23.20159541128345992, 4.773278322869455970 ) ) ;
#6082=CARTESIAN_POINT ( 'NONE',  ( 1.639793706121975614, -8.364901960018411131, 1.622639882261793343 ) ) ;
#6086=CARTESIAN_POINT ( 'NONE',  ( -13.37499999999998224, -19.49999999999991473, 4.333333333333343695 ) ) ;
#6087=CARTESIAN_POINT ( 'NONE',  ( 5.027808582316793284, -23.72900456129165647, 4.275561207030568411 ) ) ;
#6088=CARTESIAN_POINT ( 'NONE',  ( -12.62505438222622622, -20.99725369757571869, 4.613400783263607252 ) ) ;
#6090=CARTESIAN_POINT ( 'NONE',  ( 6.715308582316796837, -23.02099543870833998, 3.136473910504556262 ) ) ;
#6092=CARTESIAN_POINT ( 'NONE',  ( 10.84719141768317741, -21.53509896474923835, 2.520995438708346192 ) ) ;
#6093=CARTESIAN_POINT ( 'NONE',  ( -5.871558582316794173, -20.24999999999999289, 3.449312527122348371 ) ) ;
#6095=CARTESIAN_POINT ( 'NONE',  ( 13.09559422631463654, 4.265008428887424152, 5.017082219073495608 ) ) ;
#6100=CARTESIAN_POINT ( 'NONE',  ( -13.00900269284621302, -0.8578640112522492034, 5.903024842915844062 ) ) ;
#6101=CARTESIAN_POINT ( 'NONE',  ( -0.5631383031621635116, -8.364917468222230923, 2.372643865078341019 ) ) ;
#6102=CARTESIAN_POINT ( 'NONE',  ( -13.87467358130843387, 4.983515856073828409, 5.065827972856573602 ) ) ;
#6109=CARTESIAN_POINT ( 'NONE',  ( -11.40280858231679595, -23.08622137881038938, 1.020995438708339309 ) ) ;
#6110=CARTESIAN_POINT ( 'NONE',  ( -2.195822829018478473, -9.226849102155203042, 1.651390144731336163 ) ) ;
#6112=CARTESIAN_POINT ( 'NONE',  ( -13.82811627091129836, 3.382371681020614584, 5.229645796715683304 ) ) ;
#6114=CARTESIAN_POINT ( 'NONE',  ( 12.06594141768317741, -23.73192549717336064, 1.696391591240623331 ) ) ;
#6115=CARTESIAN_POINT ( 'NONE',  ( -11.96530858231679773, -20.97900456129165647, 3.863526089495444626 ) ) ;
#6117=CARTESIAN_POINT ( 'NONE',  ( 13.87066368810231154, 4.781016249162736820, 5.617237349937618696 ) ) ;
#6125=CARTESIAN_POINT ( 'NONE',  ( -13.54769662923970763, -11.52882022337116119, 5.659013032956382361 ) ) ;
#6126=CARTESIAN_POINT ( 'NONE',  ( 1.717920576997000737, -9.114924032904250240, 2.372645551019823884 ) ) ;
#6131=CARTESIAN_POINT ( 'NONE',  ( 1.819865260185086875, -9.122006307963404836, 1.624464420737683046 ) ) ;
#6133=CARTESIAN_POINT ( 'NONE',  ( 13.10252221513633941, 3.864871864382954048, 6.004587342915129966 ) ) ;
#6137=CARTESIAN_POINT ( 'NONE',  ( 8.034691417683175629, -20.97900456129164581, 3.136473910504570917 ) ) ;
#6138=CARTESIAN_POINT ( 'NONE',  ( -12.64751377014909828, -19.11305460747000495, 5.510446717915143289 ) ) ;
#6139=CARTESIAN_POINT ( 'NONE',  ( -12.80905858231679417, -22.74294823697954016, 2.828734674606448785 ) ) ;
#6140=CARTESIAN_POINT ( 'NONE',  ( -5.409691417683178294, -21.01515356694492098, 6.020995438708349745 ) ) ;
#6142=CARTESIAN_POINT ( 'NONE',  ( 13.09543520949579865, 4.256978079540234106, 5.067654010725516578 ) ) ;
#6148=CARTESIAN_POINT ( 'NONE',  ( 1.716273078461125090, -9.866787073280026021, 2.373124017006284170 ) ) ;
#6154=DIRECTION ( 'NONE',  ( -0.1351665943404259662, -0.9596796555888893465, 0.2464649070825324084 ) ) ;
#6155=CARTESIAN_POINT ( 'NONE',  ( -2.196516900615978152, -11.19187256518208784, 1.963432442569047698 ) ) ;
#6159=CARTESIAN_POINT ( 'NONE',  ( 9.065941417683177406, -23.73192549717336064, 1.696391591240623331 ) ) ;
#6160=CARTESIAN_POINT ( 'NONE',  ( -10.37844141768317741, -23.74999999999999645, 3.449312527122335492 ) ) ;
#6162=ORIENTED_EDGE ( 'NONE', *, *, #15196, .F. ) ;
#6163=CARTESIAN_POINT ( 'NONE',  ( 5.027808582316793284, -23.72900456129165647, 4.275561207030568411 ) ) ;
#6165=CARTESIAN_POINT ( 'NONE',  ( -12.62499999999998401, -20.99999999999999645, 3.666666666666654084 ) ) ;
#6166=CARTESIAN_POINT ( 'NONE',  ( 7.277808582316794173, -20.27099543870833642, 2.724438792969431589 ) ) ;
#6169=FACE_OUTER_BOUND ( 'NONE', #17436, .T. ) ;
#6174=CARTESIAN_POINT ( 'NONE',  ( -10.46530858231679417, -20.22900456129164937, 4.174186261275266929 ) ) ;
#6175=CARTESIAN_POINT ( 'NONE',  ( 12.64195242771744709, -19.39390240027112000, 5.496549442168085164 ) ) ;
#6178=CARTESIAN_POINT ( 'NONE',  ( 3.506783328160878010, -9.991161114504492957, 2.040295720924476530 ) ) ;
#6181=CARTESIAN_POINT ( 'NONE',  ( -13.37500751150753864, -19.49962066887028556, 4.515663405036051792 ) ) ;
#6182=CARTESIAN_POINT ( 'NONE',  ( 7.277808582316794173, -20.27099543870833642, 2.724438792969431589 ) ) ;
#6183=CARTESIAN_POINT ( 'NONE',  ( -12.62499999999998401, -20.99999999999999645, 3.666666666666654084 ) ) ;
#6185=CARTESIAN_POINT ( 'NONE',  ( 5.590308582316794173, -21.32581373872472597, 1.729004561291657582 ) ) ;
#6186=CARTESIAN_POINT ( 'NONE',  ( 6.347191417683176518, -21.53509896474923835, 2.520995438708346192 ) ) ;
#6187=CARTESIAN_POINT ( 'NONE',  ( -11.69094141768317563, -23.27327832286946219, 4.701595411283453707 ) ) ;
#6189=CARTESIAN_POINT ( 'NONE',  ( 13.57153706873194032, -9.574878029060977624, 4.950999963380944280 ) ) ;
#6190=CARTESIAN_POINT ( 'NONE',  ( -1.754777266914451461, -9.116337928146160507, 1.623008667563337726 ) ) ;
#6197=CARTESIAN_POINT ( 'NONE',  ( -3.537356407578672535, -11.36437789272258669, 3.142965222332344766 ) ) ;
#6198=CARTESIAN_POINT ( 'NONE',  ( -13.39542766346049518, -19.21840299524461315, 5.493648449623241170 ) ) ;
#6201=CARTESIAN_POINT ( 'NONE',  ( 13.09030858231679417, -21.32581373872472952, 1.729004561291657138 ) ) ;
#6203=CARTESIAN_POINT ( 'NONE',  ( 13.12035191997235906, 4.015271958632619764, 6.757839745787993735 ) ) ;
#6204=CARTESIAN_POINT ( 'NONE',  ( -6.996558582316795949, -22.05068747287764452, 0.9999999999999978906 ) ) ;
#6205=CARTESIAN_POINT ( 'NONE',  ( -1.744064896197293324, -9.868721669903177229, 1.623620860066563365 ) ) ;
#6207=CARTESIAN_POINT ( 'NONE',  ( -13.84501465882535598, 4.235740270674679842, 5.020612255068622076 ) ) ;
#6209=CARTESIAN_POINT ( 'NONE',  ( 5.597191417683177406, -23.08622137881040359, 5.979004561291654696 ) ) ;
#6210=CARTESIAN_POINT ( 'NONE',  ( -12.71530858231679417, -23.02099543870833998, 3.136473910504556262 ) ) ;
#6212=CARTESIAN_POINT ( 'NONE',  ( 13.37499999999998224, -20.99999999999998934, 4.166666666666637653 ) ) ;
#6225=CARTESIAN_POINT ( 'NONE',  ( 1.652577328807104839, -9.114908150887895744, 1.622641472200749835 ) ) ;
#6227=LINE ( 'NONE', #19207, #86 ) ;
#6231=CARTESIAN_POINT ( 'NONE',  ( -3.047379876266447685, -13.13734219723468755, 3.405682891496055742 ) ) ;
#6232=CARTESIAN_POINT ( 'NONE',  ( 4.659691417683177406, -22.36352608949543352, 2.479004561291652031 ) ) ;
#6233=CARTESIAN_POINT ( 'NONE',  ( -12.62500000000002132, -19.49999999999450040, 3.833333333368183382 ) ) ;
#6234=CARTESIAN_POINT ( 'NONE',  ( -11.77780858231679595, -21.02099543870833998, 3.035098964749253003 ) ) ;
#6235=CARTESIAN_POINT ( 'NONE',  ( -7.097191417683176518, -23.08622137881040359, 5.979004561291654696 ) ) ;
#6237=CARTESIAN_POINT ( 'NONE',  ( 13.08559773465513487, 3.760185600081874746, 5.252303440007609403 ) ) ;
#6242=CARTESIAN_POINT ( 'NONE',  ( 2.579281110863027582, -9.822567596814183233, 2.554382554832406615 ) ) ;
#6244=CARTESIAN_POINT ( 'NONE',  ( 12.53469141768317741, -20.22900456129164581, 2.825813738724748170 ) ) ;
#6246=CARTESIAN_POINT ( 'NONE',  ( -1.857501949683560971, -9.975525523312803955, 2.401050223243493154 ) ) ;
#6248=CARTESIAN_POINT ( 'NONE',  ( -10.55905858231679595, -20.72672167713054137, 4.701595411283463477 ) ) ;
#6251=CARTESIAN_POINT ( 'NONE',  ( 9.159691417683175629, -22.98484643305507191, 0.9790045612916508100 ) ) ;
#6253=CARTESIAN_POINT ( 'NONE',  ( -7.472191417683176518, -23.72900456129165292, 2.724438792969417822 ) ) ;
#6255=CARTESIAN_POINT ( 'NONE',  ( 7.559058582316794173, -20.72672167713054137, 4.701595411283463477 ) ) ;
#6257=CARTESIAN_POINT ( 'NONE',  ( -13.90439735423812273, 5.734566389025032684, 3.666666666666500873 ) ) ;
#6260=CARTESIAN_POINT ( 'NONE',  ( 6.996558582316793284, -22.05068747287764452, 1.749999999999998446 ) ) ;
#6269=CARTESIAN_POINT ( 'NONE',  ( -5.309058582316794173, -23.27327832286945153, 2.298404588716537411 ) ) ;
#6272=CARTESIAN_POINT ( 'NONE',  ( 1.126276606324276619, -9.114917468222230923, 1.622643865078341463 ) ) ;
#6274=( BOUNDED_SURFACE ( )  B_SPLINE_SURFACE ( 3, 3, ( 
 ( #7469, #12371, #18553, #4217, #4432, #1090, #13829, #10815, #12673, #17809, #9753, #19495, #4938, #1705, #17594, #9544, #17906, #16237, #15915, #6300, #19075, #6616, #16138, #3374, #5147, #229, #8400, #9643, #13092, #1592, #1804, #4732, #8190, #6519, #20643, #11525, #16029, #17490, #14556, #3170, #11318, #1903, #4837, #8089, #3573, #11120, #8286, #9852, #14345, #7972, #9952, #14660, #135, #16337, #29, #12882, #11424, #6416, #2011, #12781, #12988, #341, #19183, #6725, #11218, #3267, #14454, #19285, #17702, #19389, #5047, #3475, #18222, #7140, #2211, #20001, #10264, #12038, #10480, #3884, #19904, #4096, #13503, #11621, #3989, #13599 ),
 ( #14963, #19805, #16631, #2517, #18010, #18123, #3682, #10373, #8701, #753, #14767, #2312, #6920, #8496, #2418, #5559, #10066, #644, #16439, #7237, #444, #13289, #11930, #7032, #6823, #14866, #8809, #15072, #5460, #11832, #16747, #18432, #11731, #5667, #15178, #18324, #853, #16849, #13192, #19590, #5244, #3789, #2114, #16536, #541, #19690, #13399, #5353, #10166, #8593, #10993, #12453, #14017, #20213, #17363, #15385, #15692, #4298, #1068, #1377, #17058, #7447, #18534, #17162, #18745, #15276, #9214, #13810, #20426, #18848, #20110, #13910, #8908, #2838, #15585, #9116, #7755, #13705, #10580, #5873, #7547, #5773, #14122, #9013, #4509, #5973 ),
 ( #17257, #7645, #12144, #15485, #4197, #20527, #953, #12243, #6086, #1168, #20311, #16946, #6181, #7343, #2622, #1269, #10686, #2737, #18946, #10794, #12548, #9315, #10893, #2936, #12348, #18636, #4409, #4602, #17677, #7946, #12858, #5124, #14317, #15794, #209, #19260, #1883, #8066, #4817, #3, #12648, #313, #19362, #19054, #9425, #1474, #9729, #4914, #6497, #8264, #3349, #11504, #12758, #16215, #4711, #11291, #7852, #16113, #9617, #3050, #14630, #19161, #20623, #6593, #8168, #6392, #14215, #9520, #9830, #11194, #15892, #6699, #17571, #1572, #11099, #1781, #14534, #6276, #12961, #3243, #5019, #11399, #17470, #14429, #3147, #17784 ),
 ( #15998, #1677, #111, #3452, #13070, #19469, #9930, #13168, #14744, #16311, #420, #8370, #6800, #1983, #19568, #5221, #17884, #3551, #17179, #1393, #18551, #12260, #16967, #1287, #9134, #9335, #5890, #2645, #6198, #16866, #15504, #9231, #7667, #15711, #7564, #2535, #20546, #20130, #7776, #15403, #10705, #7467, #15602, #7363, #17078, #14139, #17273, #10595, #13928, #18653, #12566, #8925, #975, #4322, #15294, #18866, #2955, #18966, #4620, #12161, #13725, #2756, #12472, #5791, #1186, #14036, #4215, #20330, #9033, #1086, #5994, #2856, #20446, #6102, #13826, #20230, #12369, #4526, #18764, #4429, #10813, #10911, #15181, #13506, #10688, #857 ),
 ( #955, #5977, #7240, #7345, #12245, #16750, #18747, #17164, #1070, #17060, #13602, #2739, #2626, #12350, #1170, #9118, #7449, #20112, #2421, #10482, #13912, #15387, #5670, #10582, #2839, #12041, #19908, #18638, #16948, #20313, #5775, #2519, #18435, #10376, #4411, #15487, #8812, #7143, #5562, #13812, #9015, #4199, #10796, #20215, #9216, #16851, #756, #20005, #5876, #11933, #4301, #13707, #18327, #3992, #8910, #4098, #7550, #15278, #12146, #18536, #20529, #18850, #7854, #9318, #7648, #4819, #15694, #10895, #113, #11196, #15796, #6499, #1379, #1477, #6395, #17259, #12860, #11293, #15894, #17573, #7757, #3245, #4511, #2938, #17680, #3351 ),
 ( #14124, #8068, #3052, #6183, #12550, #3149, #4713, #1271, #1574, #18948, #5, #9619, #6088, #20625, #15587, #9522, #7948, #14218, #14432, #20428, #4604, #10996, #6278, #12455, #19262, #17365, #16002, #12652, #9427, #14320, #19056, #11101, #17472, #4916, #14020, #12760, #19163, #1679, #14942, #11401, #5126, #9832, #14843, #1986, #2188, #19472, #16217, #19778, #9731, #8373, #2092, #10038, #18200, #11506, #8572, #19365, #19570, #8170, #11601, #16313, #16116, #620, #17886, #6595, #5223, #12963, #423, #11703, #14632, #5021, #14746, #3454, #1783, #19666, #1885, #17786, #7007, #5329, #9933, #13375, #8266, #6802, #518, #317, #5436, #11809 ),
 ( #18100, #6701, #13072, #14536, #211, #3553, #17985, #3765, #13170, #3656, #8476, #16416, #6899, #13267, #10145, #16516, #7316, #8986, #13888, #16924, #731, #13787, #2710, #4271, #11907, #13576, #4072, #8884, #13677, #12320, #7115, #7214, #13478, #20192, #18513, #10555, #3863, #20084, #16720, #18297, #12221, #2598, #19881, #10458, #5537, #17032, #10240, #2396, #1039, #16827, #2491, #3960, #9092, #16606, #10348, #12121, #19978, #18408, #20289, #5751, #15462, #10658, #5852, #4173, #15253, #8786, #5639, #1147, #15359, #15155, #7425, #5947, #829, #2286, #18611, #7524, #8677, #929, #12012, #15046, #7620, #15972, #14292, #13989, #4385, #10768 ) ),
 .UNSPECIFIED., .T., .F., .F. ) 
 B_SPLINE_SURFACE_WITH_KNOTS ( ( 4, 3, 4 ),
 ( 4, 2, 2, 2, 2, 2, 2, 2, 2, 2, 2, 2, 2, 2, 2, 2, 2, 2, 2, 2, 2, 2, 2, 2, 2, 2, 2, 2, 2, 2, 2, 2, 2, 2, 2, 2, 2, 2, 2, 2, 2, 2, 4 ),
 ( 0.000000000000000000, 0.5000000000000000000, 1.000000000000000000 ),
 ( 0.000000000000000000, 0.03481082764294501225, 0.05122453910963481460, 0.05943139484297971231, 0.06353482270965216117, 0.06763825057632461002, 0.07081696859385246123, 0.07399568661138031245, 0.08035312264643601488, 0.09306799471654741973, 0.1057828667866588246, 0.1121403028217145270, 0.1153190208392423644, 0.1184977388567702156, 0.1214804596100246270, 0.1244631803632790246, 0.1304286218697878197, 0.1423595048828054099, 0.1662212709088405904, 0.2139448029609109514, 0.3093918670650516733, 0.5002859952733331728, 0.6911801234816146167, 0.7866271875857553386, 0.8343507196378256996, 0.8582124856638608801, 0.8701433686768784703, 0.8761088101833873765, 0.8790915309366418295, 0.8820742516898961716, 0.8853411830926052328, 0.8886081144953141830, 0.8951419773007323055, 0.9082097029115685505, 0.9212774285224047954, 0.9278112913278229179, 0.9310782227305318681, 0.9343451541332409294, 0.9384485819999133227, 0.9425520098665858271, 0.9507588655999306138, 0.9671725770666204092, 1.000000000000000000 ),
 .UNSPECIFIED. ) 
 GEOMETRIC_REPRESENTATION_ITEM ( )  RATIONAL_B_SPLINE_SURFACE ( (
 ( 1.000000000000000000, 1.000000000000000000, 1.000000000000000000, 1.000000000000000000, 1.000000000000000000, 1.000000000000000000, 1.000000000000000000, 1.000000000000000000, 1.000000000000000000, 1.000000000000000000, 1.000000000000000000, 1.000000000000000000, 1.000000000000000000, 1.000000000000000000, 1.000000000000000000, 1.000000000000000000, 1.000000000000000000, 1.000000000000000000, 1.000000000000000000, 1.000000000000000000, 1.000000000000000000, 1.000000000000000000, 1.000000000000000000, 1.000000000000000000, 1.000000000000000000, 1.000000000000000000, 1.000000000000000000, 1.000000000000000000, 1.000000000000000000, 1.000000000000000000, 1.000000000000000000, 1.000000000000000000, 1.000000000000000000, 1.000000000000000000, 1.000000000000000000, 1.000000000000000000, 1.000000000000000000, 1.000000000000000000, 1.000000000000000000, 1.000000000000000000, 1.000000000000000000, 1.000000000000000000, 1.000000000000000000, 1.000000000000000000, 1.000000000000000000, 1.000000000000000000, 1.000000000000000000, 1.000000000000000000, 1.000000000000000000, 1.000000000000000000, 1.000000000000000000, 1.000000000000000000, 1.000000000000000000, 1.000000000000000000, 1.000000000000000000, 1.000000000000000000, 1.000000000000000000, 1.000000000000000000, 1.000000000000000000, 1.000000000000000000, 1.000000000000000000, 1.000000000000000000, 1.000000000000000000, 1.000000000000000000, 1.000000000000000000, 1.000000000000000000, 1.000000000000000000, 1.000000000000000000, 1.000000000000000000, 1.000000000000000000, 1.000000000000000000, 1.000000000000000000, 1.000000000000000000, 1.000000000000000000, 1.000000000000000000, 1.000000000000000000, 1.000000000000000000, 1.000000000000000000, 1.000000000000000000, 1.000000000000000000, 1.000000000000000000, 1.000000000000000000, 1.000000000000000000, 1.000000000000000000, 1.000000000000000000, 1.000000000000000000),
 ( 0.3333333333333333703, 0.3333333333333333703, 0.3333333333333333703, 0.3333333333333333703, 0.3333333333333333703, 0.3333333333333333703, 0.3333333333333333703, 0.3333333333333333703, 0.3333333333333333703, 0.3333333333333333703, 0.3333333333333333703, 0.3333333333333333703, 0.3333333333333333703, 0.3333333333333333703, 0.3333333333333333703, 0.3333333333333333703, 0.3333333333333333703, 0.3333333333333333703, 0.3333333333333333703, 0.3333333333333333703, 0.3333333333333333703, 0.3333333333333333703, 0.3333333333333333703, 0.3333333333333333703, 0.3333333333333333703, 0.3333333333333333703, 0.3333333333333333703, 0.3333333333333333703, 0.3333333333333333703, 0.3333333333333333703, 0.3333333333333333703, 0.3333333333333333703, 0.3333333333333333703, 0.3333333333333333703, 0.3333333333333333703, 0.3333333333333333703, 0.3333333333333333703, 0.3333333333333333703, 0.3333333333333333703, 0.3333333333333333703, 0.3333333333333333703, 0.3333333333333333703, 0.3333333333333333703, 0.3333333333333333703, 0.3333333333333333703, 0.3333333333333333703, 0.3333333333333333703, 0.3333333333333333703, 0.3333333333333333703, 0.3333333333333333703, 0.3333333333333333703, 0.3333333333333333703, 0.3333333333333333703, 0.3333333333333333703, 0.3333333333333333703, 0.3333333333333333703, 0.3333333333333333703, 0.3333333333333333703, 0.3333333333333333703, 0.3333333333333333703, 0.3333333333333333703, 0.3333333333333333703, 0.3333333333333333703, 0.3333333333333333703, 0.3333333333333333703, 0.3333333333333333703, 0.3333333333333333703, 0.3333333333333333703, 0.3333333333333333703, 0.3333333333333333703, 0.3333333333333333703, 0.3333333333333333703, 0.3333333333333333703, 0.3333333333333333703, 0.3333333333333333703, 0.3333333333333333703, 0.3333333333333333703, 0.3333333333333333703, 0.3333333333333333703, 0.3333333333333333703, 0.3333333333333333703, 0.3333333333333333703, 0.3333333333333333703, 0.3333333333333333703, 0.3333333333333333703, 0.3333333333333333703),
 ( 0.3333333333333333703, 0.3333333333333333703, 0.3333333333333333703, 0.3333333333333333703, 0.3333333333333333703, 0.3333333333333333703, 0.3333333333333333703, 0.3333333333333333703, 0.3333333333333333703, 0.3333333333333333703, 0.3333333333333333703, 0.3333333333333333703, 0.3333333333333333703, 0.3333333333333333703, 0.3333333333333333703, 0.3333333333333333703, 0.3333333333333333703, 0.3333333333333333703, 0.3333333333333333703, 0.3333333333333333703, 0.3333333333333333703, 0.3333333333333333703, 0.3333333333333333703, 0.3333333333333333703, 0.3333333333333333703, 0.3333333333333333703, 0.3333333333333333703, 0.3333333333333333703, 0.3333333333333333703, 0.3333333333333333703, 0.3333333333333333703, 0.3333333333333333703, 0.3333333333333333703, 0.3333333333333333703, 0.3333333333333333703, 0.3333333333333333703, 0.3333333333333333703, 0.3333333333333333703, 0.3333333333333333703, 0.3333333333333333703, 0.3333333333333333703, 0.3333333333333333703, 0.3333333333333333703, 0.3333333333333333703, 0.3333333333333333703, 0.3333333333333333703, 0.3333333333333333703, 0.3333333333333333703, 0.3333333333333333703, 0.3333333333333333703, 0.3333333333333333703, 0.3333333333333333703, 0.3333333333333333703, 0.3333333333333333703, 0.3333333333333333703, 0.3333333333333333703, 0.3333333333333333703, 0.3333333333333333703, 0.3333333333333333703, 0.3333333333333333703, 0.3333333333333333703, 0.3333333333333333703, 0.3333333333333333703, 0.3333333333333333703, 0.3333333333333333703, 0.3333333333333333703, 0.3333333333333333703, 0.3333333333333333703, 0.3333333333333333703, 0.3333333333333333703, 0.3333333333333333703, 0.3333333333333333703, 0.3333333333333333703, 0.3333333333333333703, 0.3333333333333333703, 0.3333333333333333703, 0.3333333333333333703, 0.3333333333333333703, 0.3333333333333333703, 0.3333333333333333703, 0.3333333333333333703, 0.3333333333333333703, 0.3333333333333333703, 0.3333333333333333703, 0.3333333333333333703, 0.3333333333333333703),
 ( 1.000000000000000000, 1.000000000000000000, 1.000000000000000000, 1.000000000000000000, 1.000000000000000000, 1.000000000000000000, 1.000000000000000000, 1.000000000000000000, 1.000000000000000000, 1.000000000000000000, 1.000000000000000000, 1.000000000000000000, 1.000000000000000000, 1.000000000000000000, 1.000000000000000000, 1.000000000000000000, 1.000000000000000000, 1.000000000000000000, 1.000000000000000000, 1.000000000000000000, 1.000000000000000000, 1.000000000000000000, 1.000000000000000000, 1.000000000000000000, 1.000000000000000000, 1.000000000000000000, 1.000000000000000000, 1.000000000000000000, 1.000000000000000000, 1.000000000000000000, 1.000000000000000000, 1.000000000000000000, 1.000000000000000000, 1.000000000000000000, 1.000000000000000000, 1.000000000000000000, 1.000000000000000000, 1.000000000000000000, 1.000000000000000000, 1.000000000000000000, 1.000000000000000000, 1.000000000000000000, 1.000000000000000000, 1.000000000000000000, 1.000000000000000000, 1.000000000000000000, 1.000000000000000000, 1.000000000000000000, 1.000000000000000000, 1.000000000000000000, 1.000000000000000000, 1.000000000000000000, 1.000000000000000000, 1.000000000000000000, 1.000000000000000000, 1.000000000000000000, 1.000000000000000000, 1.000000000000000000, 1.000000000000000000, 1.000000000000000000, 1.000000000000000000, 1.000000000000000000, 1.000000000000000000, 1.000000000000000000, 1.000000000000000000, 1.000000000000000000, 1.000000000000000000, 1.000000000000000000, 1.000000000000000000, 1.000000000000000000, 1.000000000000000000, 1.000000000000000000, 1.000000000000000000, 1.000000000000000000, 1.000000000000000000, 1.000000000000000000, 1.000000000000000000, 1.000000000000000000, 1.000000000000000000, 1.000000000000000000, 1.000000000000000000, 1.000000000000000000, 1.000000000000000000, 1.000000000000000000, 1.000000000000000000, 1.000000000000000000),
 ( 0.3333333333333333703, 0.3333333333333333703, 0.3333333333333333703, 0.3333333333333333703, 0.3333333333333333703, 0.3333333333333333703, 0.3333333333333333703, 0.3333333333333333703, 0.3333333333333333703, 0.3333333333333333703, 0.3333333333333333703, 0.3333333333333333703, 0.3333333333333333703, 0.3333333333333333703, 0.3333333333333333703, 0.3333333333333333703, 0.3333333333333333703, 0.3333333333333333703, 0.3333333333333333703, 0.3333333333333333703, 0.3333333333333333703, 0.3333333333333333703, 0.3333333333333333703, 0.3333333333333333703, 0.3333333333333333703, 0.3333333333333333703, 0.3333333333333333703, 0.3333333333333333703, 0.3333333333333333703, 0.3333333333333333703, 0.3333333333333333703, 0.3333333333333333703, 0.3333333333333333703, 0.3333333333333333703, 0.3333333333333333703, 0.3333333333333333703, 0.3333333333333333703, 0.3333333333333333703, 0.3333333333333333703, 0.3333333333333333703, 0.3333333333333333703, 0.3333333333333333703, 0.3333333333333333703, 0.3333333333333333703, 0.3333333333333333703, 0.3333333333333333703, 0.3333333333333333703, 0.3333333333333333703, 0.3333333333333333703, 0.3333333333333333703, 0.3333333333333333703, 0.3333333333333333703, 0.3333333333333333703, 0.3333333333333333703, 0.3333333333333333703, 0.3333333333333333703, 0.3333333333333333703, 0.3333333333333333703, 0.3333333333333333703, 0.3333333333333333703, 0.3333333333333333703, 0.3333333333333333703, 0.3333333333333333703, 0.3333333333333333703, 0.3333333333333333703, 0.3333333333333333703, 0.3333333333333333703, 0.3333333333333333703, 0.3333333333333333703, 0.3333333333333333703, 0.3333333333333333703, 0.3333333333333333703, 0.3333333333333333703, 0.3333333333333333703, 0.3333333333333333703, 0.3333333333333333703, 0.3333333333333333703, 0.3333333333333333703, 0.3333333333333333703, 0.3333333333333333703, 0.3333333333333333703, 0.3333333333333333703, 0.3333333333333333703, 0.3333333333333333703, 0.3333333333333333703, 0.3333333333333333703),
 ( 0.3333333333333333703, 0.3333333333333333703, 0.3333333333333333703, 0.3333333333333333703, 0.3333333333333333703, 0.3333333333333333703, 0.3333333333333333703, 0.3333333333333333703, 0.3333333333333333703, 0.3333333333333333703, 0.3333333333333333703, 0.3333333333333333703, 0.3333333333333333703, 0.3333333333333333703, 0.3333333333333333703, 0.3333333333333333703, 0.3333333333333333703, 0.3333333333333333703, 0.3333333333333333703, 0.3333333333333333703, 0.3333333333333333703, 0.3333333333333333703, 0.3333333333333333703, 0.3333333333333333703, 0.3333333333333333703, 0.3333333333333333703, 0.3333333333333333703, 0.3333333333333333703, 0.3333333333333333703, 0.3333333333333333703, 0.3333333333333333703, 0.3333333333333333703, 0.3333333333333333703, 0.3333333333333333703, 0.3333333333333333703, 0.3333333333333333703, 0.3333333333333333703, 0.3333333333333333703, 0.3333333333333333703, 0.3333333333333333703, 0.3333333333333333703, 0.3333333333333333703, 0.3333333333333333703, 0.3333333333333333703, 0.3333333333333333703, 0.3333333333333333703, 0.3333333333333333703, 0.3333333333333333703, 0.3333333333333333703, 0.3333333333333333703, 0.3333333333333333703, 0.3333333333333333703, 0.3333333333333333703, 0.3333333333333333703, 0.3333333333333333703, 0.3333333333333333703, 0.3333333333333333703, 0.3333333333333333703, 0.3333333333333333703, 0.3333333333333333703, 0.3333333333333333703, 0.3333333333333333703, 0.3333333333333333703, 0.3333333333333333703, 0.3333333333333333703, 0.3333333333333333703, 0.3333333333333333703, 0.3333333333333333703, 0.3333333333333333703, 0.3333333333333333703, 0.3333333333333333703, 0.3333333333333333703, 0.3333333333333333703, 0.3333333333333333703, 0.3333333333333333703, 0.3333333333333333703, 0.3333333333333333703, 0.3333333333333333703, 0.3333333333333333703, 0.3333333333333333703, 0.3333333333333333703, 0.3333333333333333703, 0.3333333333333333703, 0.3333333333333333703, 0.3333333333333333703, 0.3333333333333333703),
 ( 1.000000000000000000, 1.000000000000000000, 1.000000000000000000, 1.000000000000000000, 1.000000000000000000, 1.000000000000000000, 1.000000000000000000, 1.000000000000000000, 1.000000000000000000, 1.000000000000000000, 1.000000000000000000, 1.000000000000000000, 1.000000000000000000, 1.000000000000000000, 1.000000000000000000, 1.000000000000000000, 1.000000000000000000, 1.000000000000000000, 1.000000000000000000, 1.000000000000000000, 1.000000000000000000, 1.000000000000000000, 1.000000000000000000, 1.000000000000000000, 1.000000000000000000, 1.000000000000000000, 1.000000000000000000, 1.000000000000000000, 1.000000000000000000, 1.000000000000000000, 1.000000000000000000, 1.000000000000000000, 1.000000000000000000, 1.000000000000000000, 1.000000000000000000, 1.000000000000000000, 1.000000000000000000, 1.000000000000000000, 1.000000000000000000, 1.000000000000000000, 1.000000000000000000, 1.000000000000000000, 1.000000000000000000, 1.000000000000000000, 1.000000000000000000, 1.000000000000000000, 1.000000000000000000, 1.000000000000000000, 1.000000000000000000, 1.000000000000000000, 1.000000000000000000, 1.000000000000000000, 1.000000000000000000, 1.000000000000000000, 1.000000000000000000, 1.000000000000000000, 1.000000000000000000, 1.000000000000000000, 1.000000000000000000, 1.000000000000000000, 1.000000000000000000, 1.000000000000000000, 1.000000000000000000, 1.000000000000000000, 1.000000000000000000, 1.000000000000000000, 1.000000000000000000, 1.000000000000000000, 1.000000000000000000, 1.000000000000000000, 1.000000000000000000, 1.000000000000000000, 1.000000000000000000, 1.000000000000000000, 1.000000000000000000, 1.000000000000000000, 1.000000000000000000, 1.000000000000000000, 1.000000000000000000, 1.000000000000000000, 1.000000000000000000, 1.000000000000000000, 1.000000000000000000, 1.000000000000000000, 1.000000000000000000, 1.000000000000000000) ) ) 
 REPRESENTATION_ITEM ( '' )  SURFACE ( )  );
#6276=CARTESIAN_POINT ( 'NONE',  ( -13.84501469867711698, 4.235742283194553259, 4.833333333333343695 ) ) ;
#6277=CARTESIAN_POINT ( 'NONE',  ( 13.37155858231679595, -19.49999999999998934, 3.449312527122348371 ) ) ;
#6278=CARTESIAN_POINT ( 'NONE',  ( -12.65017171054692113, -19.72882861737994631, 6.192581331858542981 ) ) ;
#6281=CARTESIAN_POINT ( 'NONE',  ( 8.590308582316794173, -21.32581373872472597, 1.729004561291657582 ) ) ;
#6282=CARTESIAN_POINT ( 'NONE',  ( 4.753441417683176518, -21.94931252712233061, 2.499999999999999112 ) ) ;
#6283=CARTESIAN_POINT ( 'NONE',  ( -11.12844141768317741, -20.24999999999999289, 3.550687472877664952 ) ) ;
#6287=CARTESIAN_POINT ( 'NONE',  ( 13.37505992445764136, -19.49697381488866554, 4.539006848837218833 ) ) ;
#6296=CARTESIAN_POINT ( 'NONE',  ( -3.882031223148668886, -13.81156101447257889, 3.771450735391772557 ) ) ;
#6300=CARTESIAN_POINT ( 'NONE',  ( -12.63249216759192350, -19.87164553660301536, 5.297612231341934041 ) ) ;
#6301=CARTESIAN_POINT ( 'NONE',  ( 12.43405858231679417, -23.20159541128345992, 4.773278322869455970 ) ) ;
#6303=CARTESIAN_POINT ( 'NONE',  ( 13.15498530132288479, 5.764257716805535559, 4.833333333333343695 ) ) ;
#6305=CARTESIAN_POINT ( 'NONE',  ( -5.871558582316795949, -19.49999999999998934, 3.449312527122348371 ) ) ;
#6306=CARTESIAN_POINT ( 'NONE',  ( -2.081625295426255295, -10.37614485793134556, 1.753937271548854815 ) ) ;
#6308=CARTESIAN_POINT ( 'NONE',  ( -13.84137125862932649, 4.051748560779529384, 5.236069268230914453 ) ) ;
#6310=CARTESIAN_POINT ( 'NONE',  ( 12.34719141768317563, -21.22443879296941915, 1.770995438708345748 ) ) ;
#6311=CARTESIAN_POINT ( 'NONE',  ( -6.253441417683175629, -21.94931252712233061, 2.499999999999999112 ) ) ;
#6314=CARTESIAN_POINT ( 'NONE',  ( 13.87367531042247748, 4.933103176334663331, 5.324010972534209074 ) ) ;
#6315=CARTESIAN_POINT ( 'NONE',  ( 12.62500000000001954, -20.25000000000274269, 4.083333333315724012 ) ) ;
#6326=CARTESIAN_POINT ( 'NONE',  ( 2.659620708751979645, -10.38426118526329489, 2.698636689302993830 ) ) ;
#6328=CARTESIAN_POINT ( 'NONE',  ( 2.844469389063872811, -10.54053385813977606, 1.988770633557972012 ) ) ;
#6330=CIRCLE ( 'NONE', #9009, 0.3749999999999997224 ) ;
#6336=LINE ( 'NONE', #1735, #17397 ) ;
#6338=CARTESIAN_POINT ( 'NONE',  ( -2.623717082130370137, -10.12934627674766830, 2.633169448359191644 ) ) ;
#6340=CARTESIAN_POINT ( 'NONE',  ( 5.128441417683177406, -20.99999999999999645, 3.550687472877664952 ) ) ;
#6341=CARTESIAN_POINT ( 'NONE',  ( -13.09892531043291086, 3.683228176858501790, 6.000681092915118420 ) ) ;
#6342=CARTESIAN_POINT ( 'NONE',  ( -6.996558582316795949, -22.05068747287764452, 2.499999999999999112 ) ) ;
#6344=CARTESIAN_POINT ( 'NONE',  ( -12.44094141768317741, -20.72672167713052715, 2.298404588716546293 ) ) ;
#6347=CARTESIAN_POINT ( 'NONE',  ( 13.37499999999998224, -19.49999999999998934, 4.166666666666637653 ) ) ;
#6358=CARTESIAN_POINT ( 'NONE',  ( 12.62672070884157804, -20.24999999999983658, 3.550922209436377042 ) ) ;
#6361=CARTESIAN_POINT ( 'NONE',  ( -2.731427961995660958, -10.89409100229510052, 2.829571171190552015 ) ) ;
#6363=CARTESIAN_POINT ( 'NONE',  ( -8.871558582316794173, -20.24999999999999289, 3.449312527122348371 ) ) ;
#6365=CARTESIAN_POINT ( 'NONE',  ( 6.909691417683176518, -21.01515356694492098, 6.020995438708349745 ) ) ;
#6367=CARTESIAN_POINT ( 'NONE',  ( -6.159691417683176518, -22.67418626127524917, 1.729004561291651809 ) ) ;
#6369=CARTESIAN_POINT ( 'NONE',  ( 8.590308582316794173, -21.32581373872472597, 1.729004561291657582 ) ) ;
#6371=CARTESIAN_POINT ( 'NONE',  ( -12.62499999999998224, -20.99999999999998934, 4.166666666666637653 ) ) ;
#6375=CARTESIAN_POINT ( 'NONE',  ( 7.840308582316794173, -22.67418626127525982, 5.270995438708342640 ) ) ;
#6385=CARTESIAN_POINT ( 'NONE',  ( -7.184058582316794173, -20.79840458871652942, 2.226721677130544030 ) ) ;
#6388=CARTESIAN_POINT ( 'NONE',  ( 2.167793999318431197, -10.98794063836983703, 1.911058649813994315 ) ) ;
#6392=CARTESIAN_POINT ( 'NONE',  ( -13.84256985046264710, 4.112277448363203192, 5.213861325540929847 ) ) ;
#6394=CARTESIAN_POINT ( 'NONE',  ( 6.527808582316794173, -23.72900456129165647, 4.275561207030568411 ) ) ;
#6395=CARTESIAN_POINT ( 'NONE',  ( -13.90439706815434739, 5.734551941788608609, 5.045486763335835789 ) ) ;
#6397=CARTESIAN_POINT ( 'NONE',  ( -5.215308582316795949, -24.52099543870834708, 2.515153566944913432 ) ) ;
#6398=CARTESIAN_POINT ( 'NONE',  ( 5.496558582316794173, -22.05068747287764452, 1.749999999999998446 ) ) ;
#6399=CARTESIAN_POINT ( 'NONE',  ( 7.565941417683177406, -22.67126532539353789, 2.757051763020445634 ) ) ;
#6400=CARTESIAN_POINT ( 'NONE',  ( -8.690941417683177406, -23.27327832286946219, 4.701595411283453707 ) ) ;
#6402=CARTESIAN_POINT ( 'NONE',  ( 13.83890698502169059, 3.927302743594121903, 5.241364546715693074 ) ) ;
#6404=CARTESIAN_POINT ( 'NONE',  ( -2.693754455098655409, -10.04853567022903782, 2.237415670251142519 ) ) ;
#6412=CARTESIAN_POINT ( 'NONE',  ( -3.379380450443691952, -10.24275229525297348, 2.854909362179569587 ) ) ;
#6414=EDGE_CURVE ( 'NONE', #8228, #1847, #1561, .T. ) ;
#6415=CARTESIAN_POINT ( 'NONE',  ( 2.309828811027716977, -9.292785183284841821, 1.668323847571005603 ) ) ;
#6416=CARTESIAN_POINT ( 'NONE',  ( -13.10372118337080849, 3.925419760224517329, 6.005889426248455010 ) ) ;
#6417=CARTESIAN_POINT ( 'NONE',  ( 13.18405858231679417, -20.79840458871652942, 2.226721677130544030 ) ) ;
#6420=CARTESIAN_POINT ( 'NONE',  ( 13.11465082267961968, 3.727366545318180791, 6.751662912489328150 ) ) ;
#6422=CARTESIAN_POINT ( 'NONE',  ( -1.857501949683560971, -9.975525523312803955, 2.401050223243493154 ) ) ;
#6424=CARTESIAN_POINT ( 'NONE',  ( -13.85163507668220539, 3.820071372449974412, 5.989091157956555556 ) ) ;
#6426=CARTESIAN_POINT ( 'NONE',  ( 8.315941417683177406, -20.26807450282663225, 5.303608408759377113 ) ) ;
#6427=CARTESIAN_POINT ( 'NONE',  ( -12.05905858231679595, -21.25705176302045274, 4.171265325393551215 ) ) ;
#6429=CARTESIAN_POINT ( 'NONE',  ( 13.90439735423812273, 5.734566389025032684, 3.666666666666500873 ) ) ;
#6430=CARTESIAN_POINT ( 'NONE',  ( 12.66369984131459070, -18.29565801360988075, 5.528024842915327142 ) ) ;
#6439=CARTESIAN_POINT ( 'NONE',  ( -2.601332995093193379, -9.970398767539743190, 2.592349323443654097 ) ) ;
#6442=CARTESIAN_POINT ( 'NONE',  ( 2.022757268986824730, -10.07035769906783784, 1.675405020440470238 ) ) ;
#6448=CARTESIAN_POINT ( 'NONE',  ( -11.30905858231679417, -23.27327832286945153, 2.298404588716537411 ) ) ;
#6449=CARTESIAN_POINT ( 'NONE',  ( -2.659620708751979645, -10.38426118526329489, 2.698636689302993830 ) ) ;
#6450=CARTESIAN_POINT ( 'NONE',  ( 11.68405858231679595, -21.32873467460644079, 2.757051763020455404 ) ) ;
#6451=CARTESIAN_POINT ( 'NONE',  ( -13.08919463935856697, 3.941829287606363863, 5.256209690007596080 ) ) ;
#6452=CARTESIAN_POINT ( 'NONE',  ( -7.184058582316795949, -21.32873467460644079, 2.757051763020455404 ) ) ;
#6454=CARTESIAN_POINT ( 'NONE',  ( -10.37844141768317741, -23.74999999999999645, 3.449312527122335492 ) ) ;
#6456=CARTESIAN_POINT ( 'NONE',  ( 13.09173631808601002, 4.070184063342107805, 5.250510817581989009 ) ) ;
#6457=PRESENTATION_STYLE_ASSIGNMENT (( #70 ) ) ;
#6461=CARTESIAN_POINT ( 'NONE',  ( 13.41115317570721110, -19.17426462678482579, 6.244630269197427808 ) ) ;
#6462=VERTEX_POINT ( 'NONE', #15834 ) ;
#6468=CARTESIAN_POINT ( 'NONE',  ( 10.00344141768317563, -22.05068747287765873, 5.250000000000000888 ) ) ;
#6471=CARTESIAN_POINT ( 'NONE',  ( -2.367358971471363649, -9.400572650371021410, 2.446005822389718087 ) ) ;
#6472=CARTESIAN_POINT ( 'NONE',  ( 2.645259258103298983, -10.28229522185712241, 2.672449792925449596 ) ) ;
#6475=CARTESIAN_POINT ( 'NONE',  ( 6.534691417683176518, -20.22900456129164581, 2.825813738724747726 ) ) ;
#6476=CARTESIAN_POINT ( 'NONE',  ( -5.597191417683179182, -22.77556120703057729, 5.229004561291655584 ) ) ;
#6478=CARTESIAN_POINT ( 'NONE',  ( 9.621558582316794173, -23.74999999999999645, 3.550687472877651629 ) ) ;
#6480=CARTESIAN_POINT ( 'NONE',  ( -12.65017171054692113, -19.72882861737994631, 6.192581331858542981 ) ) ;
#6482=CARTESIAN_POINT ( 'NONE',  ( 5.496558582316794173, -22.05068747287764452, 1.749999999999998446 ) ) ;
#6485=CYLINDRICAL_SURFACE ( 'NONE', #20309, 0.3749999999999997224 ) ;
#6486=ORIENTED_EDGE ( 'NONE', *, *, #1439, .T. ) ;
#6491=CARTESIAN_POINT ( 'NONE',  ( -7.746558582316794173, -21.94931252712234482, 5.250000000000000888 ) ) ;
#6492=CARTESIAN_POINT ( 'NONE',  ( 12.62500016093973620, -20.24999187254239175, 4.532396751752561848 ) ) ;
#6494=CARTESIAN_POINT ( 'NONE',  ( 2.196516900615978152, -11.19187256518208784, 1.963432442569047698 ) ) ;
#6495=CARTESIAN_POINT ( 'NONE',  ( 12.63465172146706728, -19.76258806590802664, 5.372658420469845986 ) ) ;
#6497=CARTESIAN_POINT ( 'NONE',  ( -13.80173896975277437, 2.050317972508536535, 5.200999963382010094 ) ) ;
#6498=CARTESIAN_POINT ( 'NONE',  ( 5.590308582316794173, -21.32581373872472597, 1.729004561291657582 ) ) ;
#6499=CARTESIAN_POINT ( 'NONE',  ( -13.90394305879618386, 5.711624469205903942, 5.287712306078340418 ) ) ;
#6502=CARTESIAN_POINT ( 'NONE',  ( -10.65280858231679595, -20.91377862118960351, 5.979004561291660913 ) ) ;
#6503=CARTESIAN_POINT ( 'NONE',  ( 4.746558582316793284, -21.94931252712234482, 5.250000000000000888 ) ) ;
#6504=CARTESIAN_POINT ( 'NONE',  ( 13.18405858231679595, -21.32873467460644079, 2.757051763020455404 ) ) ;
#6505=CARTESIAN_POINT ( 'NONE',  ( -8.972191417683177406, -23.72900456129164937, 2.724438792969417378 ) ) ;
#6508=CARTESIAN_POINT ( 'NONE',  ( 13.84501469867711698, 4.235742283194553259, 4.333333333333380999 ) ) ;
#6510=DIRECTION ( 'NONE',  ( 0.000000000000000000, 0.2487476929738665354, 0.9685683172808094987 ) ) ;
#6516=CARTESIAN_POINT ( 'NONE',  ( -3.767139617958116471, -12.99583330722436791, 3.561955564372631500 ) ) ;
#6519=CARTESIAN_POINT ( 'NONE',  ( -12.65410809543883985, -18.78004118034163739, 5.517608176248461227 ) ) ;
#6522=CARTESIAN_POINT ( 'NONE',  ( 13.15498566372047762, 5.764276017890828108, 4.942557026581394730 ) ) ;
#6523=CARTESIAN_POINT ( 'NONE',  ( -1.791727654783324741, -9.894249715907907472, 2.380176972254574697 ) ) ;
#6525=CARTESIAN_POINT ( 'NONE',  ( -13.58606361274418184, -9.591287556442823714, 5.700679699621803209 ) ) ;
#6529=CARTESIAN_POINT ( 'NONE',  ( 8.972191417683177406, -24.47900456129165292, 2.413778621189595963 ) ) ;
#6530=CARTESIAN_POINT ( 'NONE',  ( -6.340308582316796837, -22.36352608949544418, 4.520995438708343528 ) ) ;
#6532=CARTESIAN_POINT ( 'NONE',  ( 12.62672826945118665, -20.91272239271162903, 5.058631648758789900 ) ) ;
#6533=CARTESIAN_POINT ( 'NONE',  ( 13.11514659413808737, 4.502403003978772134, 5.887634658581065494 ) ) ;
#6541=CARTESIAN_POINT ( 'NONE',  ( 1.903957340438703572, -10.27085516675799148, 2.476896775482616331 ) ) ;
#6547=CARTESIAN_POINT ( 'NONE',  ( -13.37500000115922383, -20.34836590895906383, 3.448843053848043017 ) ) ;
#6548=CARTESIAN_POINT ( 'NONE',  ( -13.09358652029869141, 4.163619275088517035, 5.207983256689002083 ) ) ;
#6549=CARTESIAN_POINT ( 'NONE',  ( -10.74655858231679417, -21.94931252712234482, 5.250000000000000888 ) ) ;
#6551=CARTESIAN_POINT ( 'NONE',  ( -5.690941417683176518, -23.27327832286946219, 4.701595411283453707 ) ) ;
#6553=CARTESIAN_POINT ( 'NONE',  ( 13.37939227869017600, -19.27818992614120575, 4.741950614318236390 ) ) ;
#6563=CARTESIAN_POINT ( 'NONE',  ( 11.69094141768317563, -23.27327832286946219, 4.701595411283453707 ) ) ;
#6565=CARTESIAN_POINT ( 'NONE',  ( -1.824488249492779879, -9.124319963227819130, 2.375058613629473570 ) ) ;
#6566=CARTESIAN_POINT ( 'NONE',  ( 2.567175533087980188, -9.771398394011347577, 2.541241281345096859 ) ) ;
#6567=CARTESIAN_POINT ( 'NONE',  ( -10.18405858231679417, -20.79840458871652942, 2.226721677130544030 ) ) ;
#6568=CARTESIAN_POINT ( 'NONE',  ( 11.97219141768317563, -23.72900456129165292, 2.724438792969417822 ) ) ;
#6570=CARTESIAN_POINT ( 'NONE',  ( -11.69094141768317741, -22.74294823697955081, 4.171265325393542334 ) ) ;
#6573=CARTESIAN_POINT ( 'NONE',  ( 11.49655858231679595, -22.05068747287764452, 0.9999999999999978906 ) ) ;
#6574=CARTESIAN_POINT ( 'NONE',  ( 12.64751377014909828, -19.11305460747000495, 5.510446717915143289 ) ) ;
#6575=CARTESIAN_POINT ( 'NONE',  ( -12.64131715375063258, -19.42598373559290792, 5.491151580003103660 ) ) ;
#6587=CARTESIAN_POINT ( 'NONE',  ( -4.717959273841178636, -21.72818306014730183, 5.243595146365860771 ) ) ;
#6590=CARTESIAN_POINT ( 'NONE',  ( 1.709849555000590104, -9.864920124259167977, 1.622644547201689713 ) ) ;
#6591=CARTESIAN_POINT ( 'NONE',  ( 13.15498530132288479, 5.764257716805535559, 4.833333333333343695 ) ) ;
#6592=CARTESIAN_POINT ( 'NONE',  ( 4.509702210102194186, -21.62229224690691609, 4.864344626361499557 ) ) ;
#6593=CARTESIAN_POINT ( 'NONE',  ( -13.84137125862932649, 4.051748560779529384, 5.236069268230914453 ) ) ;
#6594=CARTESIAN_POINT ( 'NONE',  ( 8.590308582316797725, -21.01515356694490322, 0.9790045612916562501 ) ) ;
#6595=CARTESIAN_POINT ( 'NONE',  ( -13.12860732321105139, 4.432169822159808703, 6.709107302035562270 ) ) ;
#6599=CARTESIAN_POINT ( 'NONE',  ( 7.934058582316792396, -23.20159541128345992, 4.773278322869455970 ) ) ;
#6600=CARTESIAN_POINT ( 'NONE',  ( 4.003441417683175629, -22.05068747287766229, 4.499999999999999112 ) ) ;
#6601=CARTESIAN_POINT ( 'NONE',  ( -6.534691417683176518, -20.22900456129164581, 2.825813738724748170 ) ) ;
#6604=CARTESIAN_POINT ( 'NONE',  ( 13.84501469867711698, 4.235742283194553259, 4.833333333333343695 ) ) ;
#6613=CARTESIAN_POINT ( 'NONE',  ( -0.2815691515810352374, -8.364917468222230923, 1.622643865078524428 ) ) ;
#6614=CARTESIAN_POINT ( 'NONE',  ( 1.619022621591187150, -9.114917468222230923, 2.372643865078341019 ) ) ;
#6616=CARTESIAN_POINT ( 'NONE',  ( -12.63819864697926754, -19.58346832754827105, 5.450273968536036406 ) ) ;
#6617=CARTESIAN_POINT ( 'NONE',  ( 5.871558582316794173, -20.24999999999999289, 3.449312527122348371 ) ) ;
#6620=CARTESIAN_POINT ( 'NONE',  ( 13.11145189917479392, 4.315820908324673688, 5.961432613039677086 ) ) ;
#6622=CARTESIAN_POINT ( 'NONE',  ( 0.000000000000000000, -9.114917468222230923, 2.372643865078340575 ) ) ;
#6624=CARTESIAN_POINT ( 'NONE',  ( -13.80667376788930056, 1.549525278393783179, 5.940263032956496048 ) ) ;
#6627=CARTESIAN_POINT ( 'NONE',  ( 7.753441417683177406, -21.94931252712233061, 0.9999999999999978906 ) ) ;
#6628=CARTESIAN_POINT ( 'NONE',  ( -5.590308582316795949, -21.63647391050454871, 2.479004561291657804 ) ) ;
#6629=ORIENTED_EDGE ( 'NONE', *, *, #20205, .F. ) ;
#6630=CARTESIAN_POINT ( 'NONE',  ( 13.90439735423812273, 5.734566389025032684, 4.791666666666684726 ) ) ;
#6631=CARTESIAN_POINT ( 'NONE',  ( 13.08573665985359824, 3.017201322601628100, 5.986358176248492313 ) ) ;
#6641=CARTESIAN_POINT ( 'NONE',  ( 1.126276606324276619, -9.864917468222230923, 1.622643865078341907 ) ) ;
#6647=CARTESIAN_POINT ( 'NONE',  ( -1.957016269584227031, -9.152392576945766578, 2.382268221639079364 ) ) ;
#6651=CARTESIAN_POINT ( 'NONE',  ( -12.63958155142659834, -18.76363165295958524, 4.767928440007602298 ) ) ;
#6652=CARTESIAN_POINT ( 'NONE',  ( -5.871558582316795949, -20.99999999999999645, 3.449312527122348371 ) ) ;
#6653=CARTESIAN_POINT ( 'NONE',  ( -6.347191417683176518, -21.22443879296941915, 1.770995438708345748 ) ) ;
#6656=CARTESIAN_POINT ( 'NONE',  ( 13.84137125862932649, 4.051748560779529384, 5.236069268230914453 ) ) ;
#6666=CARTESIAN_POINT ( 'NONE',  ( 8.315941417683177406, -20.79840458871654363, 4.773278322869464851 ) ) ;
#6669=CARTESIAN_POINT ( 'NONE',  ( -1.700193846275138032, -9.865151716929458914, 2.372704024825938340 ) ) ;
#6670=CARTESIAN_POINT ( 'NONE',  ( 3.277163086644854229, -14.76879761173520578, 3.824673233536266537 ) ) ;
#6671=CARTESIAN_POINT ( 'NONE',  ( -11.59030858231679417, -21.32581373872472952, 1.729004561291657138 ) ) ;
#6675=CARTESIAN_POINT ( 'NONE',  ( 6.909691417683177406, -21.32581373872474373, 5.270995438708348857 ) ) ;
#6677=CARTESIAN_POINT ( 'NONE',  ( -4.659691417683178294, -22.67418626127524917, 1.729004561291651809 ) ) ;
#6679=CARTESIAN_POINT ( 'NONE',  ( 10.55905858231679595, -20.19639159124062999, 5.231925497173373074 ) ) ;
#6680=CARTESIAN_POINT ( 'NONE',  ( 12.62499999999998579, -20.24999999999999289, 3.146526952850934755 ) ) ;
#6681=CARTESIAN_POINT ( 'NONE',  ( -12.62499999999998224, -20.24999999999998934, 4.291666666666698937 ) ) ;
#6688=ORIENTED_EDGE ( 'NONE', *, *, #15176, .T. ) ;
#6690=CARTESIAN_POINT ( 'NONE',  ( 12.62499999999998224, -20.20698198228766529, 3.551156945995088243 ) ) ;
#6692=CARTESIAN_POINT ( 'NONE',  ( -11.59030858231679595, -21.01515356694490322, 0.9790045612916562501 ) ) ;
#6693=CARTESIAN_POINT ( 'NONE',  ( 13.12529397354238192, 5.014845663890295846, 4.583333333333296622 ) ) ;
#6696=CARTESIAN_POINT ( 'NONE',  ( 12.64131715375063258, -19.42598373559290792, 5.491151580003103660 ) ) ;
#6699=CARTESIAN_POINT ( 'NONE',  ( -13.84495141469777479, 4.232546442235974204, 5.040078719623224401 ) ) ;
#6700=CARTESIAN_POINT ( 'NONE',  ( 7.371558582316795949, -19.49999999999998934, 3.449312527122348371 ) ) ;
#6701=CARTESIAN_POINT ( 'NONE',  ( -12.62499999998404121, -20.24999999996810729, 2.793053905886972998 ) ) ;
#6702=CARTESIAN_POINT ( 'NONE',  ( -5.309058582316795949, -23.80360840875935935, 1.768074502826626260 ) ) ;
#6707=CARTESIAN_POINT ( 'NONE',  ( 6.902808582316795949, -22.46490103525074034, 2.520995438708341307 ) ) ;
#6708=CARTESIAN_POINT ( 'NONE',  ( -5.878441417683177406, -23.74999999999999645, 3.449312527122335492 ) ) ;
#6711=CARTESIAN_POINT ( 'NONE',  ( 13.37741471237955260, -20.12805702483293757, 4.993653275319895890 ) ) ;
#6713=DIRECTION ( 'NONE',  ( 0.1351665943404306014, -0.9596796555888912339, 0.2464649070825229438 ) ) ;
#6719=CARTESIAN_POINT ( 'NONE',  ( 13.37741471237955260, -20.12805702483293757, 4.993653275319895890 ) ) ;
#6725=CARTESIAN_POINT ( 'NONE',  ( -13.11017182064853159, 4.251176942750957366, 5.979809059808775196 ) ) ;
#6726=CARTESIAN_POINT ( 'NONE',  ( 9.246558582316794173, -21.94931252712234482, 5.250000000000000888 ) ) ;
#6728=CARTESIAN_POINT ( 'NONE',  ( 13.09532840572934376, 3.501584489333809724, 5.996774842915142401 ) ) ;
#6729=CARTESIAN_POINT ( 'NONE',  ( -2.203959450683124377, -9.262433282444222371, 2.410528873095051594 ) ) ;
#6732=CARTESIAN_POINT ( 'NONE',  ( -13.86106797245302147, 4.296432608878145487, 5.947261916831099171 ) ) ;
#6736=CARTESIAN_POINT ( 'NONE',  ( 9.347191417683177406, -21.22443879296941915, 1.770995438708345748 ) ) ;
#6737=CARTESIAN_POINT ( 'NONE',  ( -7.746558582316795949, -21.94931252712234127, 4.499999999999999112 ) ) ;
#6739=CARTESIAN_POINT ( 'NONE',  ( 13.86436316834274329, 3.712840001305938831, 6.736817769197426031 ) ) ;
#6740=CARTESIAN_POINT ( 'NONE',  ( 13.06655316810189227, 2.048434989138931961, 5.965524842914772030 ) ) ;
#6750=CARTESIAN_POINT ( 'NONE',  ( 2.742252025265078608, -15.06657917462210605, 2.958534504914692942 ) ) ;
#6755=CARTESIAN_POINT ( 'NONE',  ( -7.371558582316794173, -20.24999999999999289, 3.449312527122348371 ) ) ;
#6756=CARTESIAN_POINT ( 'NONE',  ( -3.549867680106858714, -10.29705900472337632, 2.118856410057032402 ) ) ;
#6758=CARTESIAN_POINT ( 'NONE',  ( -13.06641424290328501, 2.791419266617020334, 5.231470106674447784 ) ) ;
#6759=CARTESIAN_POINT ( 'NONE',  ( -5.215308582316795949, -23.02099543870833998, 3.136473910504556262 ) ) ;
#6761=CARTESIAN_POINT ( 'NONE',  ( -9.534691417683177406, -20.22900456129164581, 2.825813738724747726 ) ) ;
#6763=CARTESIAN_POINT ( 'NONE',  ( 13.53317008522746434, -11.51241069598931510, 4.909333296715523431 ) ) ;
#6769=ORIENTED_EDGE ( 'NONE', *, *, #14801, .F. ) ;
#6772=CARTESIAN_POINT ( 'NONE',  ( 4.753441417683176518, -21.94931252712233061, 1.749999999999998446 ) ) ;
#6774=CARTESIAN_POINT ( 'NONE',  ( -2.616536356806028696, -10.07836329504444706, 2.620076000170431296 ) ) ;
#6776=CARTESIAN_POINT ( 'NONE',  ( -5.215308582316794173, -23.77099543870833998, 2.825813738724734847 ) ) ;
#6778=CARTESIAN_POINT ( 'NONE',  ( 9.722191417683177406, -20.27099543870833998, 4.275561207030583510 ) ) ;
#6780=CARTESIAN_POINT ( 'NONE',  ( -10.19094141768317741, -22.74294823697955081, 4.171265325393542334 ) ) ;
#6782=CARTESIAN_POINT ( 'NONE',  ( 8.777808582316797725, -19.52099543870833642, 2.413778621189609286 ) ) ;
#6783=CARTESIAN_POINT ( 'NONE',  ( 12.68288333306630378, -17.32689168014509207, 5.548858176248425700 ) ) ;
#6784=CARTESIAN_POINT ( 'NONE',  ( -13.11862022235054503, 3.927821228673052723, 6.755987001683414483 ) ) ;
#6793=CARTESIAN_POINT ( 'NONE',  ( 12.76142888321704305, -19.96053231526083138, 3.532471378156773589 ) ) ;
#6796=CARTESIAN_POINT ( 'NONE',  ( 13.12424783836753228, 4.962015837561366993, 5.328858059679200565 ) ) ;
#6798=CARTESIAN_POINT ( 'NONE',  ( 12.64931222250080545, -19.02223276370786209, 5.512399842915133519 ) ) ;
#6800=CARTESIAN_POINT ( 'NONE',  ( -13.37503071710846925, -20.24844878602346299, 4.564052989354591361 ) ) ;
#6801=CARTESIAN_POINT ( 'NONE',  ( 9.246558582316795949, -21.94931252712234127, 6.000000000000001776 ) ) ;
#6802=CARTESIAN_POINT ( 'NONE',  ( -13.15498530132288479, 5.764257716805535559, 4.333333333333380999 ) ) ;
#6803=CARTESIAN_POINT ( 'NONE',  ( -7.184058582316795949, -20.26807450282662160, 1.696391591240633101 ) ) ;
#6807=CARTESIAN_POINT ( 'NONE',  ( 8.215308582316795949, -23.02099543870833998, 3.136473910504556262 ) ) ;
#6808=CARTESIAN_POINT ( 'NONE',  ( -4.659691417683178294, -22.67418626127524917, 1.729004561291651587 ) ) ;
#6809=ORIENTED_EDGE ( 'NONE', *, *, #8012, .T. ) ;
#6811=CARTESIAN_POINT ( 'NONE',  ( 13.37499999999998579, -20.24999999999999289, 3.146526952850934755 ) ) ;
#6819=CARTESIAN_POINT ( 'NONE',  ( 13.40621837757088564, -18.67347193267085714, 5.505367199623145247 ) ) ;
#6821=CARTESIAN_POINT ( 'NONE',  ( 3.594802210173583035, -11.77224174634763898, 3.247712807842289884 ) ) ;
#6823=CARTESIAN_POINT ( 'NONE',  ( -12.62933427970994238, -19.28111887465110996, 4.754790882998214840 ) ) ;
#6824=CARTESIAN_POINT ( 'NONE',  ( 7.371558582316794173, -20.24999999999999289, 3.449312527122348371 ) ) ;
#6826=CARTESIAN_POINT ( 'NONE',  ( 13.12424783836753228, 4.962015837561366993, 5.328858059679200565 ) ) ;
#6827=CARTESIAN_POINT ( 'NONE',  ( -2.579281110863027582, -9.822567596814183233, 2.554382554832406615 ) ) ;
#6828=CARTESIAN_POINT ( 'NONE',  ( 7.652808582316796837, -21.53509896474924901, 4.479004561291659137 ) ) ;
#6830=CARTESIAN_POINT ( 'NONE',  ( 8.690941417683177406, -23.27327832286946219, 4.701595411283453707 ) ) ;
#6831=CARTESIAN_POINT ( 'NONE',  ( -7.559058582316795949, -21.25705176302045274, 4.171265325393551215 ) ) ;
#6833=CARTESIAN_POINT ( 'NONE',  ( 13.89730118381875279, 5.376209782841177898, 6.083536567043803522 ) ) ;
#6834=CARTESIAN_POINT ( 'NONE',  ( 12.64691428603184242, -19.14332855539073464, 5.509795676248469221 ) ) ;
#6835=CARTESIAN_POINT ( 'NONE',  ( -13.12499999999999467, 5.000000000000047073, 3.999999999999996447 ) ) ;
#6843=CARTESIAN_POINT ( 'NONE',  ( 1.991511895312070957, -10.01421418592441448, 1.660986244685804136 ) ) ;
#6846=CARTESIAN_POINT ( 'NONE',  ( 13.26156167763900307, -20.51872823783367750, 3.464319252107387115 ) ) ;
#6848=CARTESIAN_POINT ( 'NONE',  ( -6.715308582316794173, -23.77099543870833998, 2.825813738724734847 ) ) ;
#6849=CARTESIAN_POINT ( 'NONE',  ( -1.932703420524435112, -8.381852853175612239, 2.376993210252662969 ) ) ;
#6851=CARTESIAN_POINT ( 'NONE',  ( -12.64197948789552051, -18.64253586127677309, 4.770532606674187548 ) ) ;
#6852=CARTESIAN_POINT ( 'NONE',  ( -5.777808582316794173, -20.27099543870833642, 2.724438792969431589 ) ) ;
#6854=CARTESIAN_POINT ( 'NONE',  ( -7.847191417683176518, -21.22443879296941915, 1.770995438708345748 ) ) ;
#6857=CARTESIAN_POINT ( 'NONE',  ( 13.38210008768272630, -19.14144557202113006, 4.745270796715706396 ) ) ;
#6865=VECTOR ( 'NONE', #13859, 1000.000000000000114 ) ;
#6867=CARTESIAN_POINT ( 'NONE',  ( 5.597191417683177406, -22.77556120703057729, 5.229004561291656472 ) ) ;
#6872=CARTESIAN_POINT ( 'NONE',  ( -6.059058582316793284, -20.72672167713054137, 4.701595411283463477 ) ) ;
#6874=CARTESIAN_POINT ( 'NONE',  ( 8.597191417683177406, -22.77556120703057729, 5.229004561291655584 ) ) ;
#6876=CARTESIAN_POINT ( 'NONE',  ( -5.972191417683178294, -22.97900456129165292, 3.035098964749240125 ) ) ;
#6877=CARTESIAN_POINT ( 'NONE',  ( -7.184058582316795949, -20.26807450282662160, 1.696391591240633101 ) ) ;
#6879=CARTESIAN_POINT ( 'NONE',  ( 12.62745083560477966, -20.12623280195927933, 5.001038150054709419 ) ) ;
#6880=CARTESIAN_POINT ( 'NONE',  ( -13.08107971211413378, 2.032025461757085427, 6.715204579155630960 ) ) ;
#6888=CARTESIAN_POINT ( 'NONE',  ( 2.583953725994688533, -9.847075946378776479, 2.560676788604062004 ) ) ;
#6892=CARTESIAN_POINT ( 'NONE',  ( 13.10252221513633941, 3.864871864382954048, 6.004587342915129966 ) ) ;
#6895=CARTESIAN_POINT ( 'NONE',  ( 13.15498530132288479, 5.764257716805535559, 2.999999999999999556 ) ) ;
#6896=CARTESIAN_POINT ( 'NONE',  ( -2.693754455098655409, -9.955255285363838524, 2.600628789231445470 ) ) ;
#6898=CARTESIAN_POINT ( 'NONE',  ( 10.55905858231679595, -20.19639159124062999, 5.231925497173373074 ) ) ;
#6899=CARTESIAN_POINT ( 'NONE',  ( -12.62503117662529739, -20.24842558042254836, 4.565011198945062354 ) ) ;
#6900=CARTESIAN_POINT ( 'NONE',  ( -5.027808582316795949, -24.47900456129166358, 4.586221378810390270 ) ) ;
#6903=CARTESIAN_POINT ( 'NONE',  ( 8.965308582316795949, -20.97900456129165647, 3.863526089495444626 ) ) ;
#6907=CARTESIAN_POINT ( 'NONE',  ( 13.87470602645761986, 4.985154336109792972, 4.791666666666685614 ) ) ;
#6914=CARTESIAN_POINT ( 'NONE',  ( 13.37503071710846925, -20.24844878602346299, 4.564052989354591361 ) ) ;
#6916=CARTESIAN_POINT ( 'NONE',  ( 1.717920576997000737, -9.114924032904250240, 2.372645551019823884 ) ) ;
#6919=CARTESIAN_POINT ( 'NONE',  ( 1.852280067228949445, -9.126254559850970338, 1.625555456689752321 ) ) ;
#6920=CARTESIAN_POINT ( 'NONE',  ( -12.62500797102436678, -19.49959746326937093, 4.516621614626514791 ) ) ;
#6921=CARTESIAN_POINT ( 'NONE',  ( 5.684058582316794173, -20.79840458871652942, 2.226721677130544030 ) ) ;
#6923=CARTESIAN_POINT ( 'NONE',  ( 12.64691428603184242, -19.14332855539073464, 5.509795676248469221 ) ) ;
#6924=CARTESIAN_POINT ( 'NONE',  ( -3.277163086644854229, -14.76879761173520578, 3.824673233536266537 ) ) ;
#6926=CARTESIAN_POINT ( 'NONE',  ( 6.809058582316796837, -22.74294823697954016, 2.828734674606448785 ) ) ;
#6929=CARTESIAN_POINT ( 'NONE',  ( 9.815941417683177406, -20.79840458871654363, 4.773278322869464851 ) ) ;
#6930=CARTESIAN_POINT ( 'NONE',  ( -7.840308582316795949, -22.36352608949544418, 4.520995438708343528 ) ) ;
#6932=CARTESIAN_POINT ( 'NONE',  ( 13.11862022235054503, 3.927821228673052723, 6.755987001683414483 ) ) ;
#6933=CARTESIAN_POINT ( 'NONE',  ( 12.63036675113625407, -19.22897906761645004, 4.757923088130392664 ) ) ;
#6942=CARTESIAN_POINT ( 'NONE',  ( 2.817596665886821672, -11.50588678273290988, 2.986692549455723267 ) ) ;
#6947=( BOUNDED_CURVE ( )  B_SPLINE_CURVE ( 3, ( #5071, #18995, #4651, #11448 ),
 .UNSPECIFIED., .F., .T. ) 
 B_SPLINE_CURVE_WITH_KNOTS ( ( 4, 4 ),
 ( 0.001172421487176120289, 0.001187255941418635012 ),
 .UNSPECIFIED. ) 
 CURVE ( )  GEOMETRIC_REPRESENTATION_ITEM ( )  RATIONAL_B_SPLINE_CURVE ( ( 0.9999999999999996669, 0.9870550161812248202, 0.9743613912715525238, 0.9619191252709827777 ) ) 
 REPRESENTATION_ITEM ( '' )  );
#6948=CARTESIAN_POINT ( 'NONE',  ( 12.69334382635811487, -20.46623033821147786, 3.541734007794558270 ) ) ;
#6950=CARTESIAN_POINT ( 'NONE',  ( -10.37155858231679417, -20.24999999999999289, 3.449312527122348371 ) ) ;
#6951=CARTESIAN_POINT ( 'NONE',  ( -1.884282074604925583, -8.375506800461993251, 2.375363417140690547 ) ) ;
#6953=CARTESIAN_POINT ( 'NONE',  ( -13.40368151590352497, -18.05158344687463412, 4.768708296715732153 ) ) ;
#6954=CARTESIAN_POINT ( 'NONE',  ( -8.027808582316792396, -23.72900456129165647, 4.275561207030568411 ) ) ;
#6955=CARTESIAN_POINT ( 'NONE',  ( -5.128441417683177406, -20.24999999999999289, 3.550687472877664952 ) ) ;
#6957=CARTESIAN_POINT ( 'NONE',  ( 13.42766088059286922, -16.84062553004338625, 4.794749963382423985 ) ) ;
#6966=AXIS2_PLACEMENT_3D ( 'NONE', #19561, #5526, #16408 ) ;
#6969=CARTESIAN_POINT ( 'NONE',  ( 7.190941417683176518, -23.27327832286946219, 4.701595411283453707 ) ) ;
#6975=CARTESIAN_POINT ( 'NONE',  ( 1.126276606324276619, -8.364917468222230923, 2.372643865078341019 ) ) ;
#6977=CARTESIAN_POINT ( 'NONE',  ( 13.90439735423812273, 5.734566389025032684, 4.166666666666765551 ) ) ;
#6979=CARTESIAN_POINT ( 'NONE',  ( 13.50000000000000178, 5.000000000000047962, 2.000000000000000000 ) ) ;
#6981=CARTESIAN_POINT ( 'NONE',  ( 10.56594141768317741, -22.67126532539353789, 2.757051763020445634 ) ) ;
#6983=CARTESIAN_POINT ( 'NONE',  ( -9.065941417683177406, -22.67126532539353789, 2.757051763020445634 ) ) ;
#6984=CARTESIAN_POINT ( 'NONE',  ( -8.215308582316795949, -24.52099543870834708, 2.515153566944913432 ) ) ;
#6986=CARTESIAN_POINT ( 'NONE',  ( 13.09293046926041626, 3.380488697651010011, 5.994170676248444352 ) ) ;
#6987=CARTESIAN_POINT ( 'NONE',  ( -13.15498530132288479, 5.764257716805535559, 3.666666666666500873 ) ) ;
#6996=CARTESIAN_POINT ( 'NONE',  ( 13.12229871761221744, -19.89213912024655784, 3.483647646711293788 ) ) ;
#7000=CARTESIAN_POINT ( 'NONE',  ( 12.66369984131459070, -18.29565801360988075, 5.528024842915327142 ) ) ;
#7001=CARTESIAN_POINT ( 'NONE',  ( -1.731569788986178304, -8.364930642962441709, 1.622647248614820015 ) ) ;
#7002=CARTESIAN_POINT ( 'NONE',  ( 1.126276606324276619, -9.114917468222230923, 2.372643865078341019 ) ) ;
#7004=CARTESIAN_POINT ( 'NONE',  ( 13.10192273101908000, 3.834597916462216816, 6.003936301248457674 ) ) ;
#7006=CARTESIAN_POINT ( 'NONE',  ( 12.52780858231679773, -24.47900456129166358, 4.586221378810390270 ) ) ;
#7007=CARTESIAN_POINT ( 'NONE',  ( -13.15498530132288479, 5.764257716805535559, 4.916666666666649199 ) ) ;
#7008=CARTESIAN_POINT ( 'NONE',  ( -9.722191417683177406, -19.52099543870834353, 4.586221378810406257 ) ) ;
#7015=CARTESIAN_POINT ( 'NONE',  ( 10.37155858231679595, -20.99999999999999645, 3.449312527122348371 ) ) ;
#7019=CARTESIAN_POINT ( 'NONE',  ( 13.85788212999909419, 4.135547564954428879, 5.982801014393342776 ) ) ;
#7027=CARTESIAN_POINT ( 'NONE',  ( 13.85403523778986390, 3.941279508358651817, 5.991705257707216958 ) ) ;
#7029=CARTESIAN_POINT ( 'NONE',  ( 4.181771508648414404, -14.78356139460145968, 3.271079850667843125 ) ) ;
#7032=CARTESIAN_POINT ( 'NONE',  ( -12.62917185724685254, -19.28932120903463598, 4.753410794856941735 ) ) ;
#7033=CARTESIAN_POINT ( 'NONE',  ( 8.402808582316792396, -22.77556120703056308, 1.770995438708340197 ) ) ;
#7035=CARTESIAN_POINT ( 'NONE',  ( 13.09892531043291086, 3.683228176858501790, 6.000681092915118420 ) ) ;
#7036=CARTESIAN_POINT ( 'NONE',  ( -2.616536356806028696, -10.07836329504444706, 2.620076000170431296 ) ) ;
#7037=CARTESIAN_POINT ( 'NONE',  ( 9.246558582316795949, -21.94931252712234127, 4.499999999999999112 ) ) ;
#7038=CARTESIAN_POINT ( 'NONE',  ( 7.097191417683177406, -22.77556120703057729, 5.229004561291655584 ) ) ;
#7039=CARTESIAN_POINT ( 'NONE',  ( -13.27780858231679595, -20.27099543870833642, 2.724438792969431589 ) ) ;
#7042=CARTESIAN_POINT ( 'NONE',  ( 12.66144083004408571, -19.15973808277258073, 6.259475412489329038 ) ) ;
#7043=CARTESIAN_POINT ( 'NONE',  ( 12.62933427970994238, -19.28111887465110996, 4.754790882998214840 ) ) ;
#7055=CARTESIAN_POINT ( 'NONE',  ( 0.000000000000000000, -9.864917468222230923, 2.372643865078341019 ) ) ;
#7059=CARTESIAN_POINT ( 'NONE',  ( 12.79015364697802504, -20.56461506584171062, 3.528352462579536386 ) ) ;
#7061=CARTESIAN_POINT ( 'NONE',  ( -10.27780858231679417, -20.27099543870833642, 2.724438792969431589 ) ) ;
#7063=CARTESIAN_POINT ( 'NONE',  ( -3.996922828336520794, -14.62728872172488437, 3.980945906412841850 ) ) ;
#7065=CARTESIAN_POINT ( 'NONE',  ( -13.38569699238614952, -18.95980188449660986, 4.749177046715717054 ) ) ;
#7066=CARTESIAN_POINT ( 'NONE',  ( -5.496558582316794173, -22.05068747287764452, 1.749999999999998446 ) ) ;
#7067=CARTESIAN_POINT ( 'NONE',  ( -7.284691417683176518, -23.02099543870834353, 3.863526089495429972 ) ) ;
#7069=CARTESIAN_POINT ( 'NONE',  ( 13.85163507668220539, 3.820071372449974412, 5.989091157956555556 ) ) ;
#7081=CARTESIAN_POINT ( 'NONE',  ( 5.409691417683177406, -21.32581373872474373, 5.270995438708348857 ) ) ;
#7084=CARTESIAN_POINT ( 'NONE',  ( 2.616191246582922680, -8.630616848980537270, 2.440880773935528048 ) ) ;
#7085=CARTESIAN_POINT ( 'NONE',  ( -4.717959273841178636, -21.72818306014730183, 5.243595146365860771 ) ) ;
#7086=CARTESIAN_POINT ( 'NONE',  ( 12.65457057572495181, -19.50668592589112293, 6.238308001337955488 ) ) ;
#7088=CARTESIAN_POINT ( 'NONE',  ( 6.159691417683176518, -22.67418626127524917, 1.729004561291651809 ) ) ;
#7090=CARTESIAN_POINT ( 'NONE',  ( -8.597191417683177406, -22.46490103525075810, 4.479004561291653808 ) ) ;
#7092=CARTESIAN_POINT ( 'NONE',  ( -5.496558582316795949, -22.05068747287764452, 0.9999999999999978906 ) ) ;
#7094=CARTESIAN_POINT ( 'NONE',  ( 12.62515856830665584, -19.49199230051052822, 4.565864671500353467 ) ) ;
#7095=CARTESIAN_POINT ( 'NONE',  ( -13.09892531043291086, 3.683228176858501790, 6.000681092915118420 ) ) ;
#7107=CARTESIAN_POINT ( 'NONE',  ( 13.12529397354238192, 5.014845663890295846, 4.833333333333344584 ) ) ;
#7108=CARTESIAN_POINT ( 'NONE',  ( -3.385922596301560894, -9.481287983549590237, 1.909350115156127403 ) ) ;
#7112=CARTESIAN_POINT ( 'NONE',  ( 13.11017182064853159, 4.251176942750957366, 5.979809059808775196 ) ) ;
#7114=CARTESIAN_POINT ( 'NONE',  ( 10.37844141768317741, -24.50000000000000000, 3.449312527122335048 ) ) ;
#7115=CARTESIAN_POINT ( 'NONE',  ( -12.64751377014909828, -19.11305460747000495, 5.510446717915143289 ) ) ;
#7116=CARTESIAN_POINT ( 'NONE',  ( -4.847191417683177406, -20.91377862118959285, 1.020995438708345082 ) ) ;
#7120=CARTESIAN_POINT ( 'NONE',  ( -13.85593616229004610, 4.037276195647738319, 5.992122970672676630 ) ) ;
#7122=CARTESIAN_POINT ( 'NONE',  ( 11.40280858231679595, -22.46490103525074034, 2.520995438708341307 ) ) ;
#7128=CARTESIAN_POINT ( 'NONE',  ( 13.66279757975024722, -5.716222222589476765, 5.784013032957989964 ) ) ;
#7135=CARTESIAN_POINT ( 'NONE',  ( 13.47096266223369376, -15.40388555723029462, 5.575679699623145247 ) ) ;
#7137=CARTESIAN_POINT ( 'NONE',  ( 0.9854920305337622199, -8.364917468222230923, 2.372643865078341019 ) ) ;
#7140=CARTESIAN_POINT ( 'NONE',  ( -13.12526104302547836, 5.013182672784613381, 5.066812735559260261 ) ) ;
#7142=CARTESIAN_POINT ( 'NONE',  ( 12.34030858231679240, -22.67418626127525982, 5.270995438708342640 ) ) ;
#7143=CARTESIAN_POINT ( 'NONE',  ( -13.44712222274167246, -17.35782775154002522, 6.283692769197384287 ) ) ;
#7145=CARTESIAN_POINT ( 'NONE',  ( 7.465308582316796837, -20.97900456129165647, 3.863526089495444626 ) ) ;
#7146=CARTESIAN_POINT ( 'NONE',  ( 6.534691417683176518, -20.22900456129164581, 2.825813738724747726 ) ) ;
#7147=CARTESIAN_POINT ( 'NONE',  ( -9.902808582316794173, -22.77556120703056308, 1.770995438708339975 ) ) ;
#7150=CARTESIAN_POINT ( 'NONE',  ( 13.08107971211413378, 2.032025461757085427, 6.715204579155630960 ) ) ;
#7151=CARTESIAN_POINT ( 'NONE',  ( 13.09455366754861139, 4.212460211200554916, 5.160171780694988719 ) ) ;
#7159=CARTESIAN_POINT ( 'NONE',  ( 1.619022621591186928, -9.864917468222230923, 2.372643865078341019 ) ) ;
#7163=CARTESIAN_POINT ( 'NONE',  ( 12.67201297282924344, -20.43364036046235555, 3.544560889254710023 ) ) ;
#7165=CARTESIAN_POINT ( 'NONE',  ( -9.809058582316794173, -23.27327832286945153, 2.298404588716537411 ) ) ;
#7166=CARTESIAN_POINT ( 'NONE',  ( -4.181771508648414404, -14.78356139460145968, 3.271079850667843125 ) ) ;
#7168=CARTESIAN_POINT ( 'NONE',  ( -13.37499999998404299, -19.49999999996810729, 2.793053905886972998 ) ) ;
#7169=CARTESIAN_POINT ( 'NONE',  ( -7.277808582316794173, -20.27099543870833642, 2.724438792969431589 ) ) ;
#7170=CARTESIAN_POINT ( 'NONE',  ( 12.34030858231679773, -22.98484643305508612, 6.020995438708344416 ) ) ;
#7171=CARTESIAN_POINT ( 'NONE',  ( -8.878441417683177406, -22.99999999999999645, 3.449312527122335048 ) ) ;
#7173=CARTESIAN_POINT ( 'NONE',  ( 13.37883250981221472, -20.05645825448334563, 5.102688967256983510 ) ) ;
#7174=DIRECTION ( 'NONE',  ( 0.000000000000000000, -0.000000000000000000, -1.000000000000000000 ) ) ;
#7179=CARTESIAN_POINT ( 'NONE',  ( -13.37499999999998224, -20.25000000000006395, 4.416666666666681174 ) ) ;
#7185=CARTESIAN_POINT ( 'NONE',  ( 3.951988298270009636, -13.15210598010094323, 2.852089508627633219 ) ) ;
#7186=CARTESIAN_POINT ( 'NONE',  ( -6.621558582316794173, -23.74999999999999645, 3.550687472877651629 ) ) ;
#7188=CARTESIAN_POINT ( 'NONE',  ( 13.86796007304617717, 3.894483688830428836, 6.740724019197413597 ) ) ;
#7190=CARTESIAN_POINT ( 'NONE',  ( 11.12844141768317741, -20.99999999999999645, 3.550687472877664952 ) ) ;
#7192=CARTESIAN_POINT ( 'NONE',  ( -3.974842109207560537, -21.92432777746334693, 4.506404853634142782 ) ) ;
#7193=CARTESIAN_POINT ( 'NONE',  ( -10.19094141768317741, -23.80360840875937001, 5.231925497173365081 ) ) ;
#7196=CARTESIAN_POINT ( 'NONE',  ( 12.62500004114794372, -19.49999792202770621, 4.520295319612473328 ) ) ;
#7197=CARTESIAN_POINT ( 'NONE',  ( -13.12529397354238192, 5.014845663890295846, 4.333333333333382775 ) ) ;
#7208=CARTESIAN_POINT ( 'NONE',  ( -1.652577328807104839, -9.114908150887895744, 1.622641472200749835 ) ) ;
#7213=CARTESIAN_POINT ( 'NONE',  ( 11.69094141768317741, -23.80360840875937001, 5.231925497173365081 ) ) ;
#7214=CARTESIAN_POINT ( 'NONE',  ( -12.64931222250080545, -19.02223276370786209, 5.512399842915133519 ) ) ;
#7215=CARTESIAN_POINT ( 'NONE',  ( -9.534691417683177406, -19.47900456129164581, 2.515153566944927199 ) ) ;
#7217=CARTESIAN_POINT ( 'NONE',  ( 10.46530858231679417, -20.22900456129164937, 4.174186261275266929 ) ) ;
#7219=CARTESIAN_POINT ( 'NONE',  ( -13.37923893525309715, -20.78593376972237650, 5.366589449429977954 ) ) ;
#7220=CARTESIAN_POINT ( 'NONE',  ( 13.09030858231679417, -21.32581373872472597, 1.729004561291657582 ) ) ;
#7224=CARTESIAN_POINT ( 'NONE',  ( 13.84983662433050178, 3.729249528687784920, 5.987138032956566214 ) ) ;
#7233=CARTESIAN_POINT ( 'NONE',  ( 1.824488249492779879, -9.124319963227819130, 2.375058613629473570 ) ) ;
#7237=CARTESIAN_POINT ( 'NONE',  ( -12.62691554569741648, -19.40326494227377907, 4.703927990036796736 ) ) ;
#7239=CARTESIAN_POINT ( 'NONE',  ( 12.80905858231679417, -23.27327832286945153, 2.298404588716537411 ) ) ;
#7240=CARTESIAN_POINT ( 'NONE',  ( -13.37499999999998401, -20.99999999999999645, 3.146526952850934755 ) ) ;
#7243=CARTESIAN_POINT ( 'NONE',  ( 11.21530858231679417, -23.77099543870833998, 2.825813738724734847 ) ) ;
#7244=CARTESIAN_POINT ( 'NONE',  ( 9.065941417683177406, -22.67126532539353789, 2.757051763020445634 ) ) ;
#7245=CARTESIAN_POINT ( 'NONE',  ( -4.746558582316795061, -21.94931252712234127, 4.499999999999999112 ) ) ;
#7247=CARTESIAN_POINT ( 'NONE',  ( 12.85087781109329974, -9.593170539812428288, 6.465204579154565145 ) ) ;
#7248=CARTESIAN_POINT ( 'NONE',  ( 12.62499999999998224, -19.50000000000006040, 4.416666666666682062 ) ) ;
#7258=CARTESIAN_POINT ( 'NONE',  ( 2.659620708751979645, -10.38426118526329489, 2.698636689302993830 ) ) ;
#7263=CARTESIAN_POINT ( 'NONE',  ( -11.87155858231679595, -19.49999999999998934, 3.449312527122348371 ) ) ;
#7264=CARTESIAN_POINT ( 'NONE',  ( -1.754777266914451461, -9.116337928146160507, 1.623008667563337726 ) ) ;
#7267=CARTESIAN_POINT ( 'NONE',  ( -13.37939227869017600, -19.27818992614120575, 4.741950614318236390 ) ) ;
#7268=CARTESIAN_POINT ( 'NONE',  ( -9.996558582316794173, -22.05068747287764452, 1.749999999999998446 ) ) ;
#7269=CARTESIAN_POINT ( 'NONE',  ( 10.56594141768317741, -23.73192549717336064, 1.696391591240623331 ) ) ;
#7270=CARTESIAN_POINT ( 'NONE',  ( -11.78469141768317741, -23.02099543870834353, 3.863526089495429972 ) ) ;
#7272=CARTESIAN_POINT ( 'NONE',  ( 13.77789853026076550, 0.09637577819625635367, 5.909013032956687006 ) ) ;
#7284=CARTESIAN_POINT ( 'NONE',  ( 2.076833265075072266, -8.407161531158021006, 2.383492984350220389 ) ) ;
#7286=CARTESIAN_POINT ( 'NONE',  ( 12.62543384439201510, -20.97809085820452424, 4.782403934559678937 ) ) ;
#7289=CARTESIAN_POINT ( 'NONE',  ( 6.065941417683177406, -23.20159541128344927, 2.226721677130534705 ) ) ;
#7291=CARTESIAN_POINT ( 'NONE',  ( -6.065941417683177406, -22.67126532539353789, 2.757051763020445634 ) ) ;
#7292=CARTESIAN_POINT ( 'NONE',  ( -10.00344141768317741, -22.05068747287766229, 6.000000000000001776 ) ) ;
#7295=CARTESIAN_POINT ( 'NONE',  ( 13.12529380813666435, 5.014837310896125722, 5.033295791462342628 ) ) ;
#7296=CARTESIAN_POINT ( 'NONE',  ( -13.05696142222617695, 1.564051822406025583, 5.955108176248398166 ) ) ;
#7309=CARTESIAN_POINT ( 'NONE',  ( -2.506848361495492394, -9.459347215042898327, 1.711100304737409150 ) ) ;
#7315=CARTESIAN_POINT ( 'NONE',  ( 10.56594141768317741, -23.73192549717336064, 1.696391591240623331 ) ) ;
#7316=CARTESIAN_POINT ( 'NONE',  ( -12.62599079447150885, -20.19996487918709249, 4.820256282269618886 ) ) ;
#7317=CARTESIAN_POINT ( 'NONE',  ( -6.909691417683176518, -21.01515356694492098, 6.020995438708349745 ) ) ;
#7319=CARTESIAN_POINT ( 'NONE',  ( 12.05905858231679417, -20.72672167713054137, 4.701595411283463477 ) ) ;
#7321=CARTESIAN_POINT ( 'NONE',  ( -13.90258797164900884, 5.643192568275169130, 5.568788873356017355 ) ) ;
#7323=CARTESIAN_POINT ( 'NONE',  ( 11.68405858231679417, -20.79840458871652942, 2.226721677130544030 ) ) ;
#7328=CARTESIAN_POINT ( 'NONE',  ( 13.87470602645761986, 4.985154336109792972, 4.833333333333344584 ) ) ;
#7334=CARTESIAN_POINT ( 'NONE',  ( -11.49655858231679417, -22.05068747287764452, 1.749999999999998446 ) ) ;
#7335=CARTESIAN_POINT ( 'NONE',  ( 13.87470602645761986, 4.985154336109792972, 4.666666666666619889 ) ) ;
#7339=CARTESIAN_POINT ( 'NONE',  ( 2.844469389063872811, -10.54053385813977606, 1.988770633557972012 ) ) ;
#7343=CARTESIAN_POINT ( 'NONE',  ( -13.37503747255156306, -19.49810763614315690, 4.531249681074674740 ) ) ;
#7344=CARTESIAN_POINT ( 'NONE',  ( 11.87155858231679417, -20.24999999999999289, 3.449312527122348371 ) ) ;
#7345=CARTESIAN_POINT ( 'NONE',  ( -13.37499999999998401, -20.99999999999999645, 3.666666666666654084 ) ) ;
#7348=CARTESIAN_POINT ( 'NONE',  ( 10.46530858231679417, -20.22900456129164937, 4.174186261275266929 ) ) ;
#7349=CARTESIAN_POINT ( 'NONE',  ( 10.94094141768317741, -21.25705176302044208, 2.828734674606458555 ) ) ;
#7350=CARTESIAN_POINT ( 'NONE',  ( -11.59030858231679417, -21.32581373872472597, 1.729004561291657582 ) ) ;
#7352=CARTESIAN_POINT ( 'NONE',  ( 12.62500000000002132, -19.50000000000273559, 4.083333333315724012 ) ) ;
#7361=CARTESIAN_POINT ( 'NONE',  ( -12.66849571425264287, -18.05346643024382303, 5.533233176248494978 ) ) ;
#7363=CARTESIAN_POINT ( 'NONE',  ( -13.66279757975024722, -5.716222222589476765, 5.784013032957989964 ) ) ;
#7365=CARTESIAN_POINT ( 'NONE',  ( 1.857501949683560971, -9.975525523312803955, 2.401050223243493154 ) ) ;
#7370=CARTESIAN_POINT ( 'NONE',  ( -8.684058582316795949, -20.26807450282662160, 1.696391591240633101 ) ) ;
#7371=CARTESIAN_POINT ( 'NONE',  ( -2.340131407102140848, -12.21153219924485889, 2.225301406344140531 ) ) ;
#7372=ORIENTED_EDGE ( 'NONE', *, *, #492, .T. ) ;
#7373=CARTESIAN_POINT ( 'NONE',  ( -13.37930517931174634, -19.28258844475809042, 4.742233558278135419 ) ) ;
#7377=CARTESIAN_POINT ( 'NONE',  ( 6.246558582316795949, -21.94931252712234127, 6.000000000000001776 ) ) ;
#7378=CARTESIAN_POINT ( 'NONE',  ( -10.19094141768317741, -22.74294823697955081, 4.171265325393542334 ) ) ;
#7380=CARTESIAN_POINT ( 'NONE',  ( 13.37500000000002132, -20.25000000000274269, 4.083333333315724012 ) ) ;
#7381=CARTESIAN_POINT ( 'NONE',  ( -13.12500000000000178, 5.000000000000047962, 2.000000000000000000 ) ) ;
#7388=CARTESIAN_POINT ( 'NONE',  ( -13.85223456079946303, 3.850345320370711644, 5.989742199623227847 ) ) ;
#7394=AXIS2_PLACEMENT_3D ( 'NONE', #9642, #19182, #4836 ) ;
#7396=CARTESIAN_POINT ( 'NONE',  ( 1.619022621591187150, -9.114917468222230923, 2.372643865078341019 ) ) ;
#7399=CARTESIAN_POINT ( 'NONE',  ( 12.66024186180961308, -19.22028597861421417, 6.258173329156003106 ) ) ;
#7403=CARTESIAN_POINT ( 'NONE',  ( 5.597191417683179182, -22.77556120703057729, 5.229004561291655584 ) ) ;
#7404=CARTESIAN_POINT ( 'NONE',  ( -12.62524871736568954, -20.23743977303344010, 4.661898514667671023 ) ) ;
#7405=CARTESIAN_POINT ( 'NONE',  ( -10.09030858231679595, -21.63647391050454871, 2.479004561291657804 ) ) ;
#7406=CARTESIAN_POINT ( 'NONE',  ( -9.159691417683175629, -22.98484643305507191, 0.9790045612916508100 ) ) ;
#7408=CARTESIAN_POINT ( 'NONE',  ( 12.82182472306881671, -9.560351485048736109, 4.965845106672846399 ) ) ;
#7409=CARTESIAN_POINT ( 'NONE',  ( -13.11514659413808737, 4.502403003978772134, 5.887634658581065494 ) ) ;
#7415=CARTESIAN_POINT ( 'NONE',  ( 1.742625132518061504, -9.872369070458363538, 2.374557585393312298 ) ) ;
#7420=CARTESIAN_POINT ( 'NONE',  ( -1.709849555000590104, -9.864920124259167977, 1.622644547201689713 ) ) ;
#7424=CARTESIAN_POINT ( 'NONE',  ( 10.28469141768317741, -24.52099543870834708, 4.484846433055073689 ) ) ;
#7425=CARTESIAN_POINT ( 'NONE',  ( -13.12463908936614132, 4.981774012991869505, 5.264611377988129171 ) ) ;
#7426=CARTESIAN_POINT ( 'NONE',  ( -5.503441417683177406, -22.05068747287766229, 6.000000000000001776 ) ) ;
#7429=CARTESIAN_POINT ( 'NONE',  ( 10.27780858231679417, -20.27099543870833642, 2.724438792969431589 ) ) ;
#7431=CARTESIAN_POINT ( 'NONE',  ( -13.37526900345969771, -20.98641532528209908, 4.724331462949078464 ) ) ;
#7432=CARTESIAN_POINT ( 'NONE',  ( 11.30905858231679417, -23.27327832286945153, 2.298404588716537411 ) ) ;
#7436=CARTESIAN_POINT ( 'NONE',  ( 13.37499999999998224, -20.99999999999991829, 4.333333333333343695 ) ) ;
#7438=VERTEX_POINT ( 'NONE', #11416 ) ;
#7442=CARTESIAN_POINT ( 'NONE',  ( -10.93405858231679417, -23.20159541128345992, 4.773278322869455970 ) ) ;
#7445=CARTESIAN_POINT ( 'NONE',  ( 2.506848361495492394, -9.459347215042898327, 1.711100304737409150 ) ) ;
#7447=CARTESIAN_POINT ( 'NONE',  ( -13.09106898171683930, 4.036483576700608644, 5.256123545019964816 ) ) ;
#7449=CARTESIAN_POINT ( 'NONE',  ( -13.37671366598624800, -20.91345986769124465, 5.053911344471881506 ) ) ;
#7453=CARTESIAN_POINT ( 'NONE',  ( 11.12155858231679417, -23.74999999999999645, 3.550687472877651629 ) ) ;
#7454=CARTESIAN_POINT ( 'NONE',  ( 10.65969141768317741, -22.36352608949543352, 2.479004561291652031 ) ) ;
#7455=CARTESIAN_POINT ( 'NONE',  ( -11.77780858231679417, -20.27099543870833642, 2.724438792969431589 ) ) ;
#7458=CARTESIAN_POINT ( 'NONE',  ( 13.40368151590352497, -18.05158344687463412, 4.768708296715732153 ) ) ;
#7465=CARTESIAN_POINT ( 'NONE',  ( -12.62500000000001954, -20.25000000000274269, 4.083333333315724012 ) ) ;
#7466=CARTESIAN_POINT ( 'NONE',  ( -2.594671182134835163, -9.923034775318452461, 2.580184533305832861 ) ) ;
#7467=CARTESIAN_POINT ( 'NONE',  ( -13.54769662923970763, -11.52882022337116119, 5.659013032956382361 ) ) ;
#7469=CARTESIAN_POINT ( 'NONE',  ( -12.62499999999998401, -20.24999999999998934, 2.439580858552613751 ) ) ;
#7473=CARTESIAN_POINT ( 'NONE',  ( 4.687312169500630787, -21.49117650933202128, 5.277475135490085734 ) ) ;
#7474=CARTESIAN_POINT ( 'NONE',  ( -12.34030858231679773, -22.98484643305508612, 6.020995438708344416 ) ) ;
#7475=CARTESIAN_POINT ( 'NONE',  ( -2.830107938415192148, -10.43856789473369950, 1.962583737180462418 ) ) ;
#7477=CARTESIAN_POINT ( 'NONE',  ( -13.37499999999998224, -20.24999999999998934, 4.291666666666698937 ) ) ;
#7479=CARTESIAN_POINT ( 'NONE',  ( 5.402808582316795949, -23.08622137881038938, 1.020995438708339309 ) ) ;
#7480=CARTESIAN_POINT ( 'NONE',  ( -11.12844141768317741, -20.99999999999999645, 3.550687472877664952 ) ) ;
#7482=CARTESIAN_POINT ( 'NONE',  ( 13.37500000000002132, -20.99999999999450395, 3.833333333368183382 ) ) ;
#7488=CARTESIAN_POINT ( 'NONE',  ( -13.70116456325478893, -3.778689555664588973, 5.825679699621801433 ) ) ;
#7491=CARTESIAN_POINT ( 'NONE',  ( 1.743623630681728542, -9.116095536440919744, 2.372946416531167557 ) ) ;
#7496=CARTESIAN_POINT ( 'NONE',  ( 2.808565762442263303, -10.28561894962424716, 1.923303392614186924 ) ) ;
#7504=CARTESIAN_POINT ( 'NONE',  ( 8.222191417683175629, -21.02099543870834353, 3.964901035250761208 ) ) ;
#7505=CARTESIAN_POINT ( 'NONE',  ( -12.68288333306630378, -17.32689168014509207, 5.548858176248425700 ) ) ;
#7506=CARTESIAN_POINT ( 'NONE',  ( -13.09030858231679417, -21.63647391050454871, 2.479004561291657804 ) ) ;
#7507=CARTESIAN_POINT ( 'NONE',  ( -12.06594141768317741, -23.73192549717336064, 1.696391591240623331 ) ) ;
#7509=CARTESIAN_POINT ( 'NONE',  ( 13.12529397354238192, 5.014845663890295846, 4.916666666666650087 ) ) ;
#7510=CARTESIAN_POINT ( 'NONE',  ( -13.10372118337080849, 3.925419760224517329, 6.005889426248455010 ) ) ;
#7514=CARTESIAN_POINT ( 'NONE',  ( 0.5631383031621635116, -9.864917468222230923, 2.372643865078341019 ) ) ;
#7519=CARTESIAN_POINT ( 'NONE',  ( -2.031432063436913182, -10.08997855658269671, 1.680444048616273722 ) ) ;
#7523=CARTESIAN_POINT ( 'NONE',  ( 12.44094141768317741, -20.19639159124061933, 1.768074502826635586 ) ) ;
#7524=CARTESIAN_POINT ( 'NONE',  ( -13.12529418130016445, 5.014856155665242454, 4.958178834604180629 ) ) ;
#7525=CARTESIAN_POINT ( 'NONE',  ( -10.09719141768317741, -22.77556120703057729, 5.229004561291655584 ) ) ;
#7529=CARTESIAN_POINT ( 'NONE',  ( -13.37499964066394043, -21.00001814646822496, 4.442866346476199269 ) ) ;
#7530=CARTESIAN_POINT ( 'NONE',  ( 9.809058582316794173, -23.27327832286945153, 2.298404588716537411 ) ) ;
#7534=CARTESIAN_POINT ( 'NONE',  ( 13.41834698511420676, -18.81097725173551893, 6.252442769197418926 ) ) ;
#7538=FILL_AREA_STYLE_COLOUR ( '', #19400 ) ;
#7543=CARTESIAN_POINT ( 'NONE',  ( 13.87470602645761986, 4.985154336109792972, 4.166666666666758445 ) ) ;
#7545=CARTESIAN_POINT ( 'NONE',  ( 2.780192134145684779, -10.08406280675441735, 1.871539748636713130 ) ) ;
#7547=CARTESIAN_POINT ( 'NONE',  ( -13.09560264576187905, 4.265433610975056133, 4.583333333333295734 ) ) ;
#7550=CARTESIAN_POINT ( 'NONE',  ( -13.86676110481170632, 3.833935792988865110, 6.739421935864088553 ) ) ;
#7552=CARTESIAN_POINT ( 'NONE',  ( 11.02780858231679595, -23.72900456129165647, 4.275561207030568411 ) ) ;
#7553=CARTESIAN_POINT ( 'NONE',  ( 11.78469141768317741, -23.02099543870834353, 3.863526089495429972 ) ) ;
#7554=CARTESIAN_POINT ( 'NONE',  ( -12.15969141768317563, -22.67418626127524917, 1.729004561291651587 ) ) ;
#7556=CARTESIAN_POINT ( 'NONE',  ( 13.74418849449709512, -0.8559810278826442964, 5.138499963383082125 ) ) ;
#7558=ORIENTED_EDGE ( 'NONE', *, *, #7997, .F. ) ;
#7561=EDGE_CURVE ( 'NONE', #11536, #7887, #18815, .T. ) ;
#7562=CARTESIAN_POINT ( 'NONE',  ( -13.08573665985359824, 3.017201322601628100, 5.986358176248492313 ) ) ;
#7563=CARTESIAN_POINT ( 'NONE',  ( -2.367358971471363649, -9.400572650371021410, 2.446005822389718087 ) ) ;
#7564=CARTESIAN_POINT ( 'NONE',  ( -13.40621837757088564, -18.67347193267085714, 5.505367199623145247 ) ) ;
#7572=CARTESIAN_POINT ( 'NONE',  ( -9.715308582316795949, -24.52099543870834708, 2.515153566944913432 ) ) ;
#7573=CARTESIAN_POINT ( 'NONE',  ( -2.739050625766161762, -9.875938058683834342, 1.818089155622620412 ) ) ;
#7575=CARTESIAN_POINT ( 'NONE',  ( -13.37499979530394967, -20.25001033714808329, 4.458488164327452097 ) ) ;
#7577=CARTESIAN_POINT ( 'NONE',  ( 6.621558582316796837, -24.50000000000000000, 3.550687472877651629 ) ) ;
#7578=CARTESIAN_POINT ( 'NONE',  ( -4.190941417683176518, -22.74294823697955081, 4.171265325393542334 ) ) ;
#7580=CARTESIAN_POINT ( 'NONE',  ( 13.87406079471522347, 4.952570133121557028, 5.260711232101737522 ) ) ;
#7586=CARTESIAN_POINT ( 'NONE',  ( -13.87470586348985258, 4.985146106231644225, 5.033049509202228933 ) ) ;
#7593=CARTESIAN_POINT ( 'NONE',  ( 2.506848361495492394, -9.459347215042898327, 1.711100304737409150 ) ) ;
#7599=CARTESIAN_POINT ( 'NONE',  ( 3.974842109207560537, -21.92432777746334693, 4.506404853634142782 ) ) ;
#7600=CARTESIAN_POINT ( 'NONE',  ( -13.12526104302547836, 5.013182672784613381, 5.066812735559260261 ) ) ;
#7602=CARTESIAN_POINT ( 'NONE',  ( -9.809058582316795949, -22.74294823697954016, 2.828734674606448785 ) ) ;
#7603=CARTESIAN_POINT ( 'NONE',  ( -8.784691417683177406, -24.52099543870834708, 4.484846433055073689 ) ) ;
#7605=CARTESIAN_POINT ( 'NONE',  ( 13.01365964058540037, 0.1273118495903458325, 5.174178440007729307 ) ) ;
#7609=CARTESIAN_POINT ( 'NONE',  ( 2.011668220304084542, -11.03559989230542193, 2.673298498313999794 ) ) ;
#7612=ORIENTED_EDGE ( 'NONE', *, *, #20355, .T. ) ;
#7615=CARTESIAN_POINT ( 'NONE',  ( -1.991511895312070957, -10.01421418592441448, 1.660986244685804136 ) ) ;
#7619=CARTESIAN_POINT ( 'NONE',  ( 4.565941417683176518, -23.73192549717336064, 1.696391591240623331 ) ) ;
#7620=CARTESIAN_POINT ( 'NONE',  ( -13.12529397354238192, 5.014845663890295846, 4.583333333333296622 ) ) ;
#7622=CARTESIAN_POINT ( 'NONE',  ( -11.50344141768317563, -22.05068747287765873, 5.250000000000000888 ) ) ;
#7623=( BOUNDED_CURVE ( )  B_SPLINE_CURVE ( 3, ( #6835, #17719, #13204, #8300 ),
 .UNSPECIFIED., .F., .F. ) 
 B_SPLINE_CURVE_WITH_KNOTS ( ( 4, 4 ),
 ( 1.468430546537837468E-05, 0.001172421487176120289 ),
 .UNSPECIFIED. ) 
 CURVE ( )  GEOMETRIC_REPRESENTATION_ITEM ( )  RATIONAL_B_SPLINE_CURVE ( ( 0.9619191252709937690, 0.3335846922424353656, 0.3462783171521043313, 1.000000000000000222 ) ) 
 REPRESENTATION_ITEM ( '' )  );
#7625=CARTESIAN_POINT ( 'NONE',  ( 9.340308582316794173, -22.67418626127525982, 5.270995438708342640 ) ) ;
#7627=CARTESIAN_POINT ( 'NONE',  ( -13.90439735423812273, 5.734566389025032684, 4.166666666666765551 ) ) ;
#7628=CARTESIAN_POINT ( 'NONE',  ( 8.309058582316792396, -23.27327832286945153, 2.298404588716537411 ) ) ;
#7632=CARTESIAN_POINT ( 'NONE',  ( 13.37607268932110038, -20.94582918928111681, 4.945564004704174010 ) ) ;
#7640=CARTESIAN_POINT ( 'NONE',  ( -9.527808582316792396, -23.72900456129165647, 4.275561207030568411 ) ) ;
#7643=CARTESIAN_POINT ( 'NONE',  ( 3.486710468562268961, -9.848741751643258269, 2.003719583429115492 ) ) ;
#7645=CARTESIAN_POINT ( 'NONE',  ( -13.37499999998404299, -19.49999999996810729, 2.793053905886972998 ) ) ;
#7647=CARTESIAN_POINT ( 'NONE',  ( 6.809058582316794173, -23.27327832286945153, 2.298404588716537411 ) ) ;
#7648=CARTESIAN_POINT ( 'NONE',  ( -13.88045627189955233, 4.525541730927888473, 6.662882075361062029 ) ) ;
#7652=CARTESIAN_POINT ( 'NONE',  ( 12.71530858231679240, -23.77099543870833998, 2.825813738724734847 ) ) ;
#7654=CARTESIAN_POINT ( 'NONE',  ( 9.628441417683177406, -20.99999999999999645, 3.550687472877664952 ) ) ;
#7655=CARTESIAN_POINT ( 'NONE',  ( -10.00344141768317563, -22.05068747287765873, 5.250000000000000888 ) ) ;
#7657=CARTESIAN_POINT ( 'NONE',  ( 13.37499999999998224, -19.49999999999991473, 4.333333333333343695 ) ) ;
#7658=CARTESIAN_POINT ( 'NONE',  ( -2.682825141213236009, -9.727160171598653093, 1.779880022082258373 ) ) ;
#7666=CARTESIAN_POINT ( 'NONE',  ( -1.337453470010121714, -8.364917468222230923, 2.372643865078341019 ) ) ;
#7667=CARTESIAN_POINT ( 'NONE',  ( -13.40022353639839103, -18.97621141187856608, 5.498856782956575984 ) ) ;
#7672=CARTESIAN_POINT ( 'NONE',  ( -11.96530858231679773, -19.47900456129164937, 4.484846433055089676 ) ) ;
#7673=CARTESIAN_POINT ( 'NONE',  ( -0.9854920305337622199, -8.364917468222230923, 1.622643865078341907 ) ) ;
#7676=CARTESIAN_POINT ( 'NONE',  ( -13.84501469867711698, 4.235742283194553259, 4.583333333333295734 ) ) ;
#7679=CARTESIAN_POINT ( 'NONE',  ( 4.687312169500634340, -21.32903648725300272, 5.908812401261035241 ) ) ;
#7680=CARTESIAN_POINT ( 'NONE',  ( -12.43405858231679595, -22.67126532539354855, 4.242948236979545484 ) ) ;
#7683=CARTESIAN_POINT ( 'NONE',  ( 13.40995420747273670, -19.23481252262645924, 6.243328185864100988 ) ) ;
#7690=CARTESIAN_POINT ( 'NONE',  ( -13.85593616229004610, 4.037276195647738319, 5.992122970672676630 ) ) ;
#7698=CARTESIAN_POINT ( 'NONE',  ( 1.126276606324276619, -8.364917468222230923, 1.622643865078341907 ) ) ;
#7704=CARTESIAN_POINT ( 'NONE',  ( 13.12529397354238192, 5.014845663890295846, 4.583333333333296622 ) ) ;
#7705=CARTESIAN_POINT ( 'NONE',  ( 5.034691417683177406, -20.97900456129164581, 3.136473910504570917 ) ) ;
#7706=CARTESIAN_POINT ( 'NONE',  ( -13.09293046926041626, 3.380488697651010011, 5.994170676248444352 ) ) ;
#7707=CARTESIAN_POINT ( 'NONE',  ( -9.059058582316795949, -21.25705176302045274, 4.171265325393551215 ) ) ;
#7709=CARTESIAN_POINT ( 'NONE',  ( -5.878441417683177406, -24.50000000000000000, 3.449312527122335048 ) ) ;
#7710=ORIENTED_EDGE ( 'NONE', *, *, #18846, .T. ) ;
#7711=CARTESIAN_POINT ( 'NONE',  ( 13.37499999999998224, -19.49999999999998934, 4.291666666666699825 ) ) ;
#7716=CARTESIAN_POINT ( 'NONE',  ( 1.337453470010121714, -9.864917468222230923, 2.372643865078341019 ) ) ;
#7726=CARTESIAN_POINT ( 'NONE',  ( -2.057814715640970515, -10.20705538578787852, 1.710511717200805304 ) ) ;
#7731=CARTESIAN_POINT ( 'NONE',  ( 7.097191417683176518, -23.08622137881040359, 5.979004561291654696 ) ) ;
#7733=CARTESIAN_POINT ( 'NONE',  ( -7.659691417683177406, -22.67418626127524917, 1.729004561291651809 ) ) ;
#7737=CARTESIAN_POINT ( 'NONE',  ( 9.996558582316794173, -22.05068747287764452, 1.749999999999998446 ) ) ;
#7739=CARTESIAN_POINT ( 'NONE',  ( -13.90439771357353038, 5.734584535470497180, 4.942866369314573127 ) ) ;
#7741=VECTOR ( 'NONE', #18144, 1000.000000000000000 ) ;
#7742=CARTESIAN_POINT ( 'NONE',  ( 6.809058582316794173, -23.27327832286945153, 2.298404588716537411 ) ) ;
#7750=CARTESIAN_POINT ( 'NONE',  ( -12.34030858231679240, -22.67418626127525982, 5.270995438708342640 ) ) ;
#7751=CARTESIAN_POINT ( 'NONE',  ( 12.63819864697926754, -19.58346832754827105, 5.450273968536036406 ) ) ;
#7753=CARTESIAN_POINT ( 'NONE',  ( 1.548630333695928618, -8.364917468222230923, 1.622643865078341907 ) ) ;
#7755=CARTESIAN_POINT ( 'NONE',  ( -13.09560264576187905, 4.265433610975056133, 4.916666666666649199 ) ) ;
#7756=CARTESIAN_POINT ( 'NONE',  ( 5.965308582316793284, -20.22900456129164937, 4.174186261275266929 ) ) ;
#7757=CARTESIAN_POINT ( 'NONE',  ( -13.90439735423812273, 5.734566389025032684, 4.583333333333295734 ) ) ;
#7760=CARTESIAN_POINT ( 'NONE',  ( -13.15332036705482466, 5.722234611034569873, 3.999999999999985345 ) ) ;
#7761=CARTESIAN_POINT ( 'NONE',  ( 7.840308582316794173, -22.67418626127525982, 5.270995438708342640 ) ) ;
#7763=CARTESIAN_POINT ( 'NONE',  ( 12.71530858231679417, -23.02099543870833998, 3.136473910504556262 ) ) ;
#7764=CARTESIAN_POINT ( 'NONE',  ( -6.902808582316793284, -22.77556120703056308, 1.770995438708339975 ) ) ;
#7766=CARTESIAN_POINT ( 'NONE',  ( 13.38007464613909470, -19.24373036997283037, 4.743072998953621777 ) ) ;
#7774=CARTESIAN_POINT ( 'NONE',  ( -12.62503117662529739, -20.24842558042254836, 4.565011198945062354 ) ) ;
#7775=CARTESIAN_POINT ( 'NONE',  ( -1.619022621591187150, -9.114917468222230923, 2.372643865078341019 ) ) ;
#7776=CARTESIAN_POINT ( 'NONE',  ( -13.44218742460511073, -16.85703505742523234, 5.544429699623282914 ) ) ;
#7782=CARTESIAN_POINT ( 'NONE',  ( 13.13084019862132479, 4.544930030374419339, 6.677052771569639944 ) ) ;
#7783=CARTESIAN_POINT ( 'NONE',  ( -10.84719141768317741, -20.91377862118959285, 1.020995438708345082 ) ) ;
#7784=CARTESIAN_POINT ( 'NONE',  ( -2.155282726790247239, -12.05525952636828357, 2.935167462089139256 ) ) ;
#7786=CARTESIAN_POINT ( 'NONE',  ( -13.39359219590679295, -19.31109410670777038, 5.491647114909025795 ) ) ;
#7788=CARTESIAN_POINT ( 'NONE',  ( 8.034691417683175629, -19.47900456129164581, 2.515153566944927199 ) ) ;
#7789=CARTESIAN_POINT ( 'NONE',  ( -12.24655858231679595, -21.94931252712234127, 4.499999999999999112 ) ) ;
#7791=CARTESIAN_POINT ( 'NONE',  ( 13.39169349927020569, -20.15697828685464188, 6.009339318877812808 ) ) ;
#7792=CARTESIAN_POINT ( 'NONE',  ( 12.63465172146706728, -19.76258806590802664, 5.372658420469845986 ) ) ;
#7797=CARTESIAN_POINT ( 'NONE',  ( -13.87215786865436762, 4.856472367046606564, 5.506273593909547515 ) ) ;
#7799=CARTESIAN_POINT ( 'NONE',  ( 1.957016269584227031, -9.152392576945766578, 2.382268221639079364 ) ) ;
#7804=CARTESIAN_POINT ( 'NONE',  ( 1.548630333695928396, -9.114917468222230923, 1.622643865078341463 ) ) ;
#7810=CARTESIAN_POINT ( 'NONE',  ( 8.784691417683177406, -23.02099543870834353, 3.863526089495429972 ) ) ;
#7811=CARTESIAN_POINT ( 'NONE',  ( -12.72125031657057015, -15.38935901321805133, 5.590524842915047365 ) ) ;
#7812=CARTESIAN_POINT ( 'NONE',  ( -12.34030858231679773, -22.36352608949544418, 4.520995438708343528 ) ) ;
#7813=CARTESIAN_POINT ( 'NONE',  ( -4.940941417683177406, -20.19639159124061933, 1.768074502826635586 ) ) ;
#7815=CARTESIAN_POINT ( 'NONE',  ( 13.09560264576187905, 4.265433610975056133, 3.666666666666500873 ) ) ;
#7820=CARTESIAN_POINT ( 'NONE',  ( 1.548630333695928618, -9.864917468222230923, 2.372643865078341019 ) ) ;
#7822=CARTESIAN_POINT ( 'NONE',  ( 12.06594141768317563, -23.20159541128344927, 2.226721677130534705 ) ) ;
#7825=CARTESIAN_POINT ( 'NONE',  ( -1.863950040896528604, -9.995453039732266731, 2.406168007552154098 ) ) ;
#7827=CARTESIAN_POINT ( 'NONE',  ( -8.684058582316794173, -20.79840458871652942, 2.226721677130544030 ) ) ;
#7830=CARTESIAN_POINT ( 'NONE',  ( 8.222191417683175629, -19.52099543870834353, 4.586221378810406257 ) ) ;
#7832=CARTESIAN_POINT ( 'NONE',  ( -8.128441417683175629, -20.24999999999999289, 3.550687472877664952 ) ) ;
#7834=CARTESIAN_POINT ( 'NONE',  ( 9.715308582316794173, -23.77099543870833998, 2.825813738724734847 ) ) ;
#7836=CARTESIAN_POINT ( 'NONE',  ( -12.62499999999998224, -20.99999999999991829, 4.333333333333343695 ) ) ;
#7838=CARTESIAN_POINT ( 'NONE',  ( 9.246558582316794173, -21.94931252712234482, 5.250000000000000888 ) ) ;
#7842=CARTESIAN_POINT ( 'NONE',  ( -2.693754455098655409, -10.04853567022903782, 2.237415670251142519 ) ) ;
#7843=ORIENTED_EDGE ( 'NONE', *, *, #1187, .T. ) ;
#7846=CARTESIAN_POINT ( 'NONE',  ( -11.30905858231679595, -23.80360840875935935, 1.768074502826626260 ) ) ;
#7849=CARTESIAN_POINT ( 'NONE',  ( 13.87499999999999467, 5.734882735235988349, 3.999999999999984901 ) ) ;
#7850=CARTESIAN_POINT ( 'NONE',  ( 1.744064896197293324, -9.868721669903177229, 1.623620860066563365 ) ) ;
#7852=CARTESIAN_POINT ( 'NONE',  ( -13.83770801678722329, 3.866754847752558621, 5.240062463382368030 ) ) ;
#7853=CARTESIAN_POINT ( 'NONE',  ( 8.309058582316792396, -23.27327832286945153, 2.298404588716537411 ) ) ;
#7854=CARTESIAN_POINT ( 'NONE',  ( -13.87486364728600208, 4.243114187942282456, 6.725269602253773016 ) ) ;
#7859=CARTESIAN_POINT ( 'NONE',  ( 4.940941417683177406, -21.25705176302044208, 2.828734674606458555 ) ) ;
#7860=CARTESIAN_POINT ( 'NONE',  ( -6.527808582316794173, -23.72900456129165647, 4.275561207030568411 ) ) ;
#7862=CARTESIAN_POINT ( 'NONE',  ( 13.37523871602689596, -19.48794484064217514, 4.577160611493482634 ) ) ;
#7871=CARTESIAN_POINT ( 'NONE',  ( -3.211992482548209349, -9.366834950279640637, 2.629956289783360823 ) ) ;
#7874=CARTESIAN_POINT ( 'NONE',  ( 2.682825141213236009, -9.727160171598653093, 1.779880022082258373 ) ) ;
#7876=CARTESIAN_POINT ( 'NONE',  ( 11.59030858231679417, -21.32581373872472952, 1.729004561291657138 ) ) ;
#7878=CARTESIAN_POINT ( 'NONE',  ( 12.73577686058281344, -15.40576854059989920, 6.340204579155907183 ) ) ;
#7879=CARTESIAN_POINT ( 'NONE',  ( -7.371558582316795949, -19.49999999999998934, 3.449312527122348371 ) ) ;
#7880=CARTESIAN_POINT ( 'NONE',  ( -2.049450250860079592, -10.15122911285664564, 1.696174415070213382 ) ) ;
#7882=CARTESIAN_POINT ( 'NONE',  ( -13.84500676459759383, 4.235341612176667603, 5.016097456370799179 ) ) ;
#7885=CARTESIAN_POINT ( 'NONE',  ( 12.53469141768317741, -20.22900456129164581, 2.825813738724747726 ) ) ;
#7886=CARTESIAN_POINT ( 'NONE',  ( -4.472191417683178294, -22.97900456129165292, 3.035098964749240125 ) ) ;
#7887=VERTEX_POINT ( 'NONE', #20419 ) ;
#7888=CARTESIAN_POINT ( 'NONE',  ( 13.45671396861735403, -16.87344458480707843, 6.294109435864141844 ) ) ;
#7896=CARTESIAN_POINT ( 'NONE',  ( -3.984239023773645805, -21.65718589142769446, 5.016651699346909687 ) ) ;
#7899=CARTESIAN_POINT ( 'NONE',  ( 2.226467333542268445, -8.440126719678968215, 1.641959103308203716 ) ) ;
#7904=CARTESIAN_POINT ( 'NONE',  ( -12.71530858231679240, -23.77099543870833998, 2.825813738724734847 ) ) ;
#7906=CARTESIAN_POINT ( 'NONE',  ( 5.784691417683178294, -23.02099543870834353, 3.863526089495429972 ) ) ;
#7907=CARTESIAN_POINT ( 'NONE',  ( -12.62499999999998224, -19.49999999999998934, 4.291666666666699825 ) ) ;
#7908=CARTESIAN_POINT ( 'NONE',  ( -13.27780858231679595, -20.27099543870833642, 2.724438792969431589 ) ) ;
#7910=CARTESIAN_POINT ( 'NONE',  ( -3.944195004867014909, -21.42722504787766624, 5.934029185143018914 ) ) ;
#7912=CARTESIAN_POINT ( 'NONE',  ( 13.37499999998404299, -19.49999999996810729, 2.793053905886972998 ) ) ;
#7918=ORIENTED_EDGE ( 'NONE', *, *, #19649, .T. ) ;
#7919=CARTESIAN_POINT ( 'NONE',  ( 12.44094141768317741, -20.72672167713052715, 2.298404588716546293 ) ) ;
#7921=CARTESIAN_POINT ( 'NONE',  ( -1.548630333695928396, -9.114917468222230923, 2.372643865078341019 ) ) ;
#7923=CARTESIAN_POINT ( 'NONE',  ( -12.05905858231679417, -20.72672167713054137, 4.701595411283463477 ) ) ;
#7925=CARTESIAN_POINT ( 'NONE',  ( 6.065941417683177406, -23.73192549717336064, 1.696391591240623331 ) ) ;
#7926=CARTESIAN_POINT ( 'NONE',  ( -12.06594141768317563, -23.20159541128344927, 2.226721677130534705 ) ) ;
#7928=CARTESIAN_POINT ( 'NONE',  ( 5.215308582316793284, -23.77099543870833998, 2.825813738724734847 ) ) ;
#7930=CARTESIAN_POINT ( 'NONE',  ( -13.90394305879618386, 5.711624469205903942, 5.287712306078340418 ) ) ;
#7933=CARTESIAN_POINT ( 'NONE',  ( 6.715308582316794173, -23.77099543870833998, 2.825813738724734847 ) ) ;
#7941=CARTESIAN_POINT ( 'NONE',  ( -12.90280858231679595, -23.08622137881038938, 1.020995438708339309 ) ) ;
#7942=CARTESIAN_POINT ( 'NONE',  ( 12.63249216759192350, -19.87164553660301536, 5.297612231341934041 ) ) ;
#7944=CARTESIAN_POINT ( 'NONE',  ( 1.797685059409938280, -9.880079706704160358, 1.626537830816663588 ) ) ;
#7946=CARTESIAN_POINT ( 'NONE',  ( -13.38210008768272630, -19.14144557202113006, 4.745270796715706396 ) ) ;
#7947=CARTESIAN_POINT ( 'NONE',  ( 8.777808582316792396, -20.27099543870833642, 2.724438792969431589 ) ) ;
#7948=CARTESIAN_POINT ( 'NONE',  ( -12.62672826945118665, -20.91272239271162903, 5.058631648758789900 ) ) ;
#7950=CARTESIAN_POINT ( 'NONE',  ( -9.527808582316795949, -24.47900456129166358, 4.586221378810390270 ) ) ;
#7951=CARTESIAN_POINT ( 'NONE',  ( 8.027808582316792396, -23.72900456129165647, 4.275561207030568411 ) ) ;
#7953=CARTESIAN_POINT ( 'NONE',  ( 4.847191417683177406, -21.53509896474923835, 2.520995438708346192 ) ) ;
#7954=CARTESIAN_POINT ( 'NONE',  ( -10.28469141768317741, -23.77099543870834353, 4.174186261275251830 ) ) ;
#7957=CARTESIAN_POINT ( 'NONE',  ( 13.84501469867711698, 4.235742283194553259, 4.666666666666618113 ) ) ;
#7965=CARTESIAN_POINT ( 'NONE',  ( -13.12463908936614132, 4.981774012991869505, 5.264611377988129171 ) ) ;
#7968=CARTESIAN_POINT ( 'NONE',  ( -1.513434189748285696, -9.114917468222230923, 2.372643865078341019 ) ) ;
#7972=CARTESIAN_POINT ( 'NONE',  ( -13.08094078691552831, 2.775009739235173356, 5.981149842915306714 ) ) ;
#7973=CARTESIAN_POINT ( 'NONE',  ( 9.996558582316794173, -22.05068747287764452, 1.749999999999998446 ) ) ;
#7975=CARTESIAN_POINT ( 'NONE',  ( 12.75496035233418013, -14.43700220713569138, 6.361037912489419632 ) ) ;
#7976=CARTESIAN_POINT ( 'NONE',  ( -1.866357130655357688, -10.00562759449716133, 2.408781036472938730 ) ) ;
#7978=CARTESIAN_POINT ( 'NONE',  ( -13.40382044110196347, -18.79456772435387890, 5.502763032956559108 ) ) ;
#7981=CARTESIAN_POINT ( 'NONE',  ( 7.847191417683175629, -20.91377862118959285, 1.020995438708345082 ) ) ;
#7982=CARTESIAN_POINT ( 'NONE',  ( -11.68405858231679595, -21.32873467460644079, 2.757051763020455404 ) ) ;
#7986=CARTESIAN_POINT ( 'NONE',  ( 13.89075858682503650, 5.045808634669852744, 6.406973581600956535 ) ) ;
#7987=CARTESIAN_POINT ( 'NONE',  ( 13.09892531043291086, 3.683228176858501790, 6.000681092915118420 ) ) ;
#7991=CIRCLE ( 'NONE', #1648, 0.3750000000000003331 ) ;
#7997=EDGE_CURVE ( 'NONE', #8562, #13563, #1643, .T. ) ;
#8000=CARTESIAN_POINT ( 'NONE',  ( 2.442511739767545098, -14.09457879449248807, 3.458905389639174821 ) ) ;
#8006=CARTESIAN_POINT ( 'NONE',  ( -12.05905858231679417, -20.72672167713054137, 4.701595411283463477 ) ) ;
#8007=CARTESIAN_POINT ( 'NONE',  ( -1.743623630681728542, -9.116095536440919744, 2.372946416531167557 ) ) ;
#8008=CARTESIAN_POINT ( 'NONE',  ( 11.21530858231679595, -23.02099543870833998, 3.136473910504556262 ) ) ;
#8009=CARTESIAN_POINT ( 'NONE',  ( -12.62868952012632207, -19.31367923361656480, 4.748088538831167327 ) ) ;
#8010=CARTESIAN_POINT ( 'NONE',  ( -5.965308582316795949, -20.97900456129165647, 3.863526089495444626 ) ) ;
#8012=EDGE_CURVE ( 'NONE', #13542, #13028, #17604, .T. ) ;
#8013=CARTESIAN_POINT ( 'NONE',  ( -3.974842109207560537, -21.73478823434188456, 6.006404853634143670 ) ) ;
#8016=CARTESIAN_POINT ( 'NONE',  ( 13.37500000000002132, -19.49999999999450040, 3.833333333368183382 ) ) ;
#8021=CARTESIAN_POINT ( 'NONE',  ( 13.86436316834274329, 3.712840001305938831, 6.736817769197426031 ) ) ;
#8027=COLOUR_RGB ( '', 0.66274510, 0.83137255, 0.94901961) ;
#8028=CARTESIAN_POINT ( 'NONE',  ( 10.84719141768317741, -21.22443879296941915, 1.770995438708345748 ) ) ;
#8032=CARTESIAN_POINT ( 'NONE',  ( -2.817596665886821672, -11.50588678273290988, 2.986692549455723267 ) ) ;
#8034=CARTESIAN_POINT ( 'NONE',  ( -11.49655858231679417, -22.05068747287764452, 1.749999999999998446 ) ) ;
#8037=CARTESIAN_POINT ( 'NONE',  ( 5.597191417683177406, -23.08622137881040359, 5.979004561291654696 ) ) ;
#8039=CARTESIAN_POINT ( 'NONE',  ( -5.503441417683176518, -22.05068747287765873, 5.250000000000000888 ) ) ;
#8042=CARTESIAN_POINT ( 'NONE',  ( 4.687312169500632564, -21.51559725698341197, 5.182386163300427562 ) ) ;
#8044=CARTESIAN_POINT ( 'NONE',  ( -12.62499963760179256, -21.00001830110826972, 4.442557003548452066 ) ) ;
#8049=CARTESIAN_POINT ( 'NONE',  ( 5.965308582316793284, -20.22900456129164937, 4.174186261275266929 ) ) ;
#8057=CARTESIAN_POINT ( 'NONE',  ( -6.621558582316794173, -23.74999999999999645, 3.550687472877651629 ) ) ;
#8058=CARTESIAN_POINT ( 'NONE',  ( 12.62500000000001954, -20.24999999999506173, 3.850307403176420618 ) ) ;
#8061=CARTESIAN_POINT ( 'NONE',  ( 1.548630333695928396, -9.114917468222230923, 1.622643865078341463 ) ) ;
#8064=AXIS2_PLACEMENT_3D ( 'NONE', #16969, #2857, #2646 ) ;
#8066=CARTESIAN_POINT ( 'NONE',  ( -13.41806913471718588, -17.32500869677464550, 4.784333296715663764 ) ) ;
#8067=CARTESIAN_POINT ( 'NONE',  ( 6.434058582316794173, -23.20159541128345992, 4.773278322869455970 ) ) ;
#8068=CARTESIAN_POINT ( 'NONE',  ( -12.62499999998404299, -20.99999999996810729, 2.793053905886972998 ) ) ;
#8070=CARTESIAN_POINT ( 'NONE',  ( -11.02780858231679595, -24.47900456129166358, 4.586221378810390270 ) ) ;
#8071=CARTESIAN_POINT ( 'NONE',  ( 5.871558582316794173, -20.24999999999999289, 3.449312527122348371 ) ) ;
#8072=CARTESIAN_POINT ( 'NONE',  ( 7.284691417683176518, -23.02099543870834353, 3.863526089495429972 ) ) ;
#8073=CARTESIAN_POINT ( 'NONE',  ( -8.128441417683175629, -20.24999999999999289, 3.550687472877664952 ) ) ;
#8076=CARTESIAN_POINT ( 'NONE',  ( 13.84500676459759383, 4.235341612176667603, 5.016097456370799179 ) ) ;
#8084=CARTESIAN_POINT ( 'NONE',  ( -13.10756170493883310, 4.119366099410778581, 6.001761809183453700 ) ) ;
#8085=CARTESIAN_POINT ( 'NONE',  ( -2.445888733774860935, -8.532121313016713060, 2.415585152653916712 ) ) ;
#8089=CARTESIAN_POINT ( 'NONE',  ( -12.91308523408712183, -5.701695678577235249, 5.798858176249892082 ) ) ;
#8090=CARTESIAN_POINT ( 'NONE',  ( 12.99655858231679417, -22.05068747287764452, 1.749999999999998446 ) ) ;
#8092=CARTESIAN_POINT ( 'NONE',  ( 13.11345185444515415, 3.666818649476655700, 6.750360829155977349 ) ) ;
#8094=CARTESIAN_POINT ( 'NONE',  ( -1.963707630584672570, -9.980492102769451535, 1.652325740065381909 ) ) ;
#8098=CARTESIAN_POINT ( 'NONE',  ( -13.47096266223369376, -15.40388555723029462, 5.575679699623145247 ) ) ;
#8100=CARTESIAN_POINT ( 'NONE',  ( 4.190941417683176518, -23.80360840875937001, 5.231925497173365081 ) ) ;
#8101=CARTESIAN_POINT ( 'NONE',  ( -9.340308582316795949, -22.36352608949544418, 4.520995438708343528 ) ) ;
#8103=CARTESIAN_POINT ( 'NONE',  ( 13.86833701876684088, 3.913519447696059750, 6.741146579470268740 ) ) ;
#8104=CARTESIAN_POINT ( 'NONE',  ( 13.12119116326504908, 4.807653744879115010, 5.626470997801169105 ) ) ;
#8113=CARTESIAN_POINT ( 'NONE',  ( 1.925499516411631973, -10.42380411186744382, 2.516177120048874283 ) ) ;
#8118=CARTESIAN_POINT ( 'NONE',  ( -11.21530858231679417, -23.77099543870833998, 2.825813738724734847 ) ) ;
#8119=CARTESIAN_POINT ( 'NONE',  ( -1.337453470010121714, -9.114917468222230923, 2.372643865078341019 ) ) ;
#8120=CARTESIAN_POINT ( 'NONE',  ( 8.121558582316795949, -22.99999999999999645, 3.550687472877652073 ) ) ;
#8121=CARTESIAN_POINT ( 'NONE',  ( -12.62499999999998224, -19.50000000000006040, 4.416666666666682062 ) ) ;
#8122=CARTESIAN_POINT ( 'NONE',  ( -10.93405858231679417, -23.20159541128345992, 4.773278322869455970 ) ) ;
#8124=CARTESIAN_POINT ( 'NONE',  ( -6.909691417683176518, -21.01515356694492098, 6.020995438708349745 ) ) ;
#8126=CARTESIAN_POINT ( 'NONE',  ( 13.83411111208379474, 3.685111160228107252, 5.236156213382356484 ) ) ;
#8141=CARTESIAN_POINT ( 'NONE',  ( -1.513434189748285696, -9.114917468222230923, 2.372643865078341019 ) ) ;
#8142=CARTESIAN_POINT ( 'NONE',  ( 2.594671182134835163, -9.923034775318452461, 2.580184533305832861 ) ) ;
#8143=CARTESIAN_POINT ( 'NONE',  ( -12.43405858231679417, -23.20159541128345992, 4.773278322869455970 ) ) ;
#8145=CARTESIAN_POINT ( 'NONE',  ( 11.31594141768317741, -20.79840458871654363, 4.773278322869464851 ) ) ;
#8147=CARTESIAN_POINT ( 'NONE',  ( -6.347191417683176518, -21.22443879296941915, 1.770995438708345748 ) ) ;
#8150=CARTESIAN_POINT ( 'NONE',  ( 9.715308582316795949, -24.52099543870834708, 2.515153566944913432 ) ) ;
#8151=CARTESIAN_POINT ( 'NONE',  ( 12.62499999999998224, -20.24999999999998934, 4.291666666666698937 ) ) ;
#8152=CARTESIAN_POINT ( 'NONE',  ( -13.15498530132288479, 5.764257716805535559, 4.833333333333343695 ) ) ;
#8162=CARTESIAN_POINT ( 'NONE',  ( -5.027808582316793284, -23.72900456129165647, 4.275561207030568411 ) ) ;
#8165=CARTESIAN_POINT ( 'NONE',  ( 2.044552395631970665, -10.13052631352519306, 1.690857522621936226 ) ) ;
#8166=CARTESIAN_POINT ( 'NONE',  ( 13.15498530132288479, 5.764257716805535559, 4.791666666666684726 ) ) ;
#8168=CARTESIAN_POINT ( 'NONE',  ( -13.84167967300649238, 4.067323486828401613, 5.231641758301140754 ) ) ;
#8169=CARTESIAN_POINT ( 'NONE',  ( 9.340308582316795949, -22.98484643305508612, 6.020995438708344416 ) ) ;
#8170=CARTESIAN_POINT ( 'NONE',  ( -13.11824772738305356, 3.909010232842670796, 6.755569162489314827 ) ) ;
#8172=CARTESIAN_POINT ( 'NONE',  ( 8.965308582316794173, -20.22900456129164937, 4.174186261275266929 ) ) ;
#8174=CARTESIAN_POINT ( 'NONE',  ( 7.003441417683177406, -22.05068747287766229, 4.499999999999999112 ) ) ;
#8175=CARTESIAN_POINT ( 'NONE',  ( -7.097191417683177406, -22.77556120703057729, 5.229004561291656472 ) ) ;
#8177=ORIENTED_EDGE ( 'NONE', *, *, #8012, .F. ) ;
#8178=CARTESIAN_POINT ( 'NONE',  ( 13.37500015856764435, -20.24999199233421265, 4.532157119432948633 ) ) ;
#8180=DIRECTION ( 'NONE',  ( 1.000000000000000000, 0.000000000000000000, 0.000000000000000000 ) ) ;
#8186=CARTESIAN_POINT ( 'NONE',  ( -1.407845757905374695, -8.364917468222230923, 1.622643865078341907 ) ) ;
#8190=CARTESIAN_POINT ( 'NONE',  ( -12.65051119073526564, -18.96168486786632457, 5.513701926248478102 ) ) ;
#8191=CARTESIAN_POINT ( 'NONE',  ( 8.121558582316792396, -23.74999999999999645, 3.550687472877651629 ) ) ;
#8193=CARTESIAN_POINT ( 'NONE',  ( 13.15498530131898214, 5.764257716805535559, 3.333333333333075466 ) ) ;
#8194=CARTESIAN_POINT ( 'NONE',  ( -1.859341899742023463, -9.902476528685241419, 1.632289782122827271 ) ) ;
#8196=CARTESIAN_POINT ( 'NONE',  ( -13.41341218697771609, -18.31018455762212227, 5.513179699623425023 ) ) ;
#8199=CARTESIAN_POINT ( 'NONE',  ( 6.722191417683176518, -19.52099543870834353, 4.586221378810406257 ) ) ;
#8200=CARTESIAN_POINT ( 'NONE',  ( -7.277808582316795061, -21.02099543870833998, 3.035098964749253003 ) ) ;
#8202=CARTESIAN_POINT ( 'NONE',  ( 12.62499999999998224, -20.99999999999991829, 4.333333333333343695 ) ) ;
#8203=CARTESIAN_POINT ( 'NONE',  ( 13.12526104302547836, 5.013182672784613381, 5.066812735559260261 ) ) ;
#8214=CARTESIAN_POINT ( 'NONE',  ( 0.9854920305337621089, -9.114917468222230923, 1.622643865078341463 ) ) ;
#8219=DIRECTION ( 'NONE',  ( -0.1351665943404306014, -0.9596796555888911229, 0.2464649070825229160 ) ) ;
#8220=CARTESIAN_POINT ( 'NONE',  ( -2.702705060698113115, -10.69015907548275379, 2.777197378435510622 ) ) ;
#8222=CARTESIAN_POINT ( 'NONE',  ( -12.62933427970994238, -19.28111887465110996, 4.754790882998214840 ) ) ;
#8223=CARTESIAN_POINT ( 'NONE',  ( -11.21530858231679417, -23.77099543870833998, 2.825813738724734847 ) ) ;
#8224=CARTESIAN_POINT ( 'NONE',  ( -4.472191417683177406, -23.72900456129165292, 2.724438792969417822 ) ) ;
#8226=CARTESIAN_POINT ( 'NONE',  ( 13.84090061271218985, 4.027980941966571748, 5.240332426532912535 ) ) ;
#8228=VERTEX_POINT ( 'NONE', #13009 ) ;
#8236=CARTESIAN_POINT ( 'NONE',  ( 8.784691417683177406, -23.77099543870834353, 4.174186261275251830 ) ) ;
#8238=CARTESIAN_POINT ( 'NONE',  ( -2.659620708751979645, -10.38426118526329489, 2.698636689302993830 ) ) ;
#8240=CARTESIAN_POINT ( 'NONE',  ( -10.84030858231679240, -22.67418626127525982, 5.270995438708342640 ) ) ;
#8241=CARTESIAN_POINT ( 'NONE',  ( 10.94094141768317741, -20.72672167713052715, 2.298404588716546293 ) ) ;
#8243=CARTESIAN_POINT ( 'NONE',  ( -5.222191417683178294, -20.27099543870833998, 4.275561207030583510 ) ) ;
#8245=CARTESIAN_POINT ( 'NONE',  ( 10.18405858231679595, -20.26807450282662160, 1.696391591240633101 ) ) ;
#8246=CARTESIAN_POINT ( 'NONE',  ( 12.62599079447150885, -20.19996487918709249, 4.820256282269618886 ) ) ;
#8247=CARTESIAN_POINT ( 'NONE',  ( -13.15498530132288479, 5.764257716805535559, 2.999999999999999556 ) ) ;
#8256=VERTEX_POINT ( 'NONE', #19409 ) ;
#8257=CARTESIAN_POINT ( 'NONE',  ( 2.601332995093193379, -9.970398767539743190, 2.592349323443654097 ) ) ;
#8259=CARTESIAN_POINT ( 'NONE',  ( -5.965308582316793284, -20.22900456129164937, 4.174186261275266929 ) ) ;
#8260=CARTESIAN_POINT ( 'NONE',  ( 13.11017182064853159, 4.251176942750957366, 5.979809059808775196 ) ) ;
#8262=CARTESIAN_POINT ( 'NONE',  ( 12.62499999999998224, -20.24999999999998934, 4.291666666666698937 ) ) ;
#8264=CARTESIAN_POINT ( 'NONE',  ( -13.81612658856640863, 2.776892722604777930, 5.216624963382545666 ) ) ;
#8265=CARTESIAN_POINT ( 'NONE',  ( 7.652808582316796837, -20.91377862118960351, 5.979004561291660913 ) ) ;
#8266=CARTESIAN_POINT ( 'NONE',  ( -13.15498530132288479, 5.764257716805535559, 4.583333333333295734 ) ) ;
#8267=CARTESIAN_POINT ( 'NONE',  ( -7.652808582316796837, -20.91377862118960351, 5.979004561291660913 ) ) ;
#8270=CARTESIAN_POINT ( 'NONE',  ( 7.184058582316795949, -21.32873467460644079, 2.757051763020455404 ) ) ;
#8271=CARTESIAN_POINT ( 'NONE',  ( -9.534691417683177406, -20.22900456129164581, 2.825813738724748170 ) ) ;
#8275=CARTESIAN_POINT ( 'NONE',  ( 13.37499999999998579, -20.24999999999999289, 3.666666666666653640 ) ) ;
#8282=CARTESIAN_POINT ( 'NONE',  ( -13.12529397354238192, 5.014845663890297622, 3.999999999999981792 ) ) ;
#8286=CARTESIAN_POINT ( 'NONE',  ( -13.02818618459764188, 0.1109023222084986743, 5.923858176248589125 ) ) ;
#8287=CARTESIAN_POINT ( 'NONE',  ( 6.809058582316794173, -23.27327832286945153, 2.298404588716537411 ) ) ;
#8289=CARTESIAN_POINT ( 'NONE',  ( 13.08094078691552831, 2.775009739235173356, 5.981149842915306714 ) ) ;
#8291=CARTESIAN_POINT ( 'NONE',  ( -1.126276606324276619, -9.864917468222230923, 2.372643865078341019 ) ) ;
#8293=CARTESIAN_POINT ( 'NONE',  ( -13.84504075139246915, 3.487057945321567765, 5.981929699623240282 ) ) ;
#8295=CARTESIAN_POINT ( 'NONE',  ( 8.409691417683177406, -21.32581373872474373, 5.270995438708348857 ) ) ;
#8296=CARTESIAN_POINT ( 'NONE',  ( -9.246558582316795949, -21.94931252712234127, 4.499999999999999112 ) ) ;
#8298=CARTESIAN_POINT ( 'NONE',  ( 13.56222317325195093, -11.54522975075300728, 6.408692769197242178 ) ) ;
#8299=CARTESIAN_POINT ( 'NONE',  ( 13.11145189917479392, 4.315820908324673688, 5.961432613039677086 ) ) ;
#8300=CARTESIAN_POINT ( 'NONE',  ( -13.87470602645761808, 4.985154336109792972, 4.000000000000000000 ) ) ;
#8308=LINE ( 'NONE', #5265, #1319 ) ;
#8309=CARTESIAN_POINT ( 'NONE',  ( 2.088806020750596737, -10.42712783963456857, 1.767030719737609168 ) ) ;
#8313=DIRECTION ( 'NONE',  ( 1.000000000000000000, 0.000000000000000000, 0.000000000000000000 ) ) ;
#8316=CARTESIAN_POINT ( 'NONE',  ( -3.187906586576829682, -9.105473976199601083, 1.812833570429532859 ) ) ;
#8319=CARTESIAN_POINT ( 'NONE',  ( -12.62691554569741648, -19.40326494227377907, 4.703927990036796736 ) ) ;
#8320=CARTESIAN_POINT ( 'NONE',  ( -10.65280858231679240, -21.22443879296942626, 5.229004561291659137 ) ) ;
#8321=CARTESIAN_POINT ( 'NONE',  ( -8.503441417683177406, -22.05068747287765873, 5.250000000000000888 ) ) ;
#8324=CARTESIAN_POINT ( 'NONE',  ( 13.84501469867711698, 4.235742283194553259, 4.666666666666618113 ) ) ;
#8333=CARTESIAN_POINT ( 'NONE',  ( 5.503441417683176518, -22.05068747287765873, 5.250000000000000888 ) ) ;
#8336=CARTESIAN_POINT ( 'NONE',  ( -1.126276606324276619, -9.864917468222230923, 2.372643865078341019 ) ) ;
#8338=CARTESIAN_POINT ( 'NONE',  ( -7.559058582316794173, -20.72672167713054137, 4.701595411283463477 ) ) ;
#8342=CARTESIAN_POINT ( 'NONE',  ( 10.28469141768318096, -23.77099543870834353, 4.174186261275252718 ) ) ;
#8344=CARTESIAN_POINT ( 'NONE',  ( -4.003441417683176518, -22.05068747287765873, 5.250000000000000888 ) ) ;
#8346=CARTESIAN_POINT ( 'NONE',  ( 8.965308582316795949, -19.47900456129164937, 4.484846433055089676 ) ) ;
#8348=CARTESIAN_POINT ( 'NONE',  ( 13.08573665985359824, 3.017201322601628100, 5.986358176248492313 ) ) ;
#8349=CARTESIAN_POINT ( 'NONE',  ( -13.15498501280115917, 5.764243146453090105, 5.045733045595949484 ) ) ;
#8360=CARTESIAN_POINT ( 'NONE',  ( 13.26926852418574754, -19.98898271615830424, 3.463267919252106974 ) ) ;
#8367=CARTESIAN_POINT ( 'NONE',  ( 13.15492785973632017, 5.761356916681801721, 5.116543252045025802 ) ) ;
#8370=CARTESIAN_POINT ( 'NONE',  ( -13.37500015856764435, -20.24999199233421265, 4.532157119432948633 ) ) ;
#8372=CARTESIAN_POINT ( 'NONE',  ( 9.809058582316795949, -23.80360840875935935, 1.768074502826626260 ) ) ;
#8373=CARTESIAN_POINT ( 'NONE',  ( -13.09546733092777160, 2.758600211853326822, 6.730829579156167419 ) ) ;
#8374=CARTESIAN_POINT ( 'NONE',  ( -7.090308582316795061, -21.01515356694490322, 0.9790045612916562501 ) ) ;
#8378=CARTESIAN_POINT ( 'NONE',  ( 9.246558582316795949, -21.94931252712234127, 4.499999999999999112 ) ) ;
#8379=CARTESIAN_POINT ( 'NONE',  ( -4.847191417683178294, -21.22443879296941915, 1.770995438708345748 ) ) ;
#8382=CARTESIAN_POINT ( 'NONE',  ( 13.38921792038197900, -19.53199502070850357, 5.456033026503027017 ) ) ;
#8391=CARTESIAN_POINT ( 'NONE',  ( 13.84504075139246915, 3.487057945321567765, 5.981929699623240282 ) ) ;
#8392=B_SPLINE_CURVE_WITH_KNOTS ( 'NONE', 3,
 ( #12367, #17271, #13723, #7465, #12159, #17177, #4318, #4523, #1084, #18548, #7774, #12060, #10703, #4425, #2854, #10909, #2754, #18450, #2952, #14137, #5991, #20444, #20542, #10811, #4113, #10496, #16965, #16864, #9229, #1183, #9332, #17074, #13824, #15401, #7361, #15709, #14034, #5789, #2533, #8923, #18762, #15292, #20227, #6100, #4213, #10593, #1285, #2642, #7562, #5888, #12258, #18651, #15600, #12468, #18863, #9132, #15502, #13926, #20328, #8084, #17588, #1588, #5042, #17383, #14552, #17696, #4727, #3370, #7965, #16234, #19381, #11420, #17804, #12666, #3470, #224, #9637, #17485, #16131, #3166, #9848, #8282 ),
 .UNSPECIFIED., .F., .F.,
 ( 4, 2, 2, 2, 2, 2, 2, 2, 2, 2, 2, 2, 2, 2, 2, 2, 2, 2, 2, 2, 2, 2, 2, 2, 2, 2, 2, 2, 2, 2, 2, 2, 2, 2, 2, 2, 2, 2, 2, 2, 4 ),
 ( 0.03648247254878290990, 0.05122453910963482848, 0.05943139484297973313, 0.06353482270965218892, 0.06763825057632463778, 0.07081696859385248899, 0.07399568661138034020, 0.08035312264643605651, 0.09306799471654747524, 0.1057828667866588801, 0.1121403028217145964, 0.1153190208392424337, 0.1184977388567702850, 0.1214804596100246964, 0.1244631803632790940, 0.1304286218697879030, 0.1423595048828055210, 0.1662212709088407014, 0.2139448029609111179, 0.3093918670650518954, 0.5002859952733336169, 0.6911801234816151718, 0.7866271875857560048, 0.8343507196378263657, 0.8582124856638615462, 0.8701433686768791365, 0.8761088101833880426, 0.8790915309366424957, 0.8820742516898969487, 0.8853411830926060100, 0.8886081144953148492, 0.8951419773007329717, 0.9082097029115692166, 0.9212774285224054616, 0.9278112913278236951, 0.9310782227305326453, 0.9343451541332417065, 0.9384485819999140999, 0.9425520098665866042, 0.9507588655999313909, 0.9671725770666211863 ),
 .UNSPECIFIED. ) ;
#8395=CARTESIAN_POINT ( 'NONE',  ( 3.951988298270009636, -13.15210598010094323, 2.852089508627633219 ) ) ;
#8399=CARTESIAN_POINT ( 'NONE',  ( 1.619022621591187150, -9.114917468222230923, 1.622643865078341463 ) ) ;
#8400=CARTESIAN_POINT ( 'NONE',  ( -12.64387510712649565, -19.29680709011273976, 5.506486987317513737 ) ) ;
#8401=CARTESIAN_POINT ( 'NONE',  ( 9.434058582316794173, -23.20159541128345992, 4.773278322869455970 ) ) ;
#8403=CARTESIAN_POINT ( 'NONE',  ( 13.11740841389447709, 4.616624901677048420, 5.813473370769506765 ) ) ;
#8405=CARTESIAN_POINT ( 'NONE',  ( -1.717920576997000737, -9.114924032904250240, 2.372645551019823884 ) ) ;
#8408=CARTESIAN_POINT ( 'NONE',  ( 7.472191417683176518, -23.72900456129165292, 2.724438792969417822 ) ) ;
#8409=CARTESIAN_POINT ( 'NONE',  ( -8.496558582316795949, -22.05068747287764452, 2.499999999999999112 ) ) ;
#8411=CARTESIAN_POINT ( 'NONE',  ( 13.79242507427300879, 0.07996625081441015304, 6.658692769197546824 ) ) ;
#8412=CARTESIAN_POINT ( 'NONE',  ( 13.08094078691552831, 2.775009739235173356, 5.981149842915306714 ) ) ;
#8415=ADVANCED_FACE ( 'NONE', ( #19922 ), #5685, .T. ) ;
#8422=CARTESIAN_POINT ( 'NONE',  ( 2.167793999318431197, -10.98794063836983703, 1.911058649813994315 ) ) ;
#8425=( BOUNDED_SURFACE ( )  B_SPLINE_SURFACE ( 3, 3, ( 
 ( #15619, #1302, #10722, #20658, #11133, #6315, #9152, #17502, #14053, #9458, #2772, #12489, #17404, #12277, #10927, #17095, #15929, #1411, #14155, #15520, #7792, #3084, #15830, #1507, #14248, #1606, #19403, #19602, #11538, #6834, #14569, #13203, #2022, #5061, #14779, #6430, #353, #12894, #9658, #16153, #14359, #1720, #16347, #16045, #242, #17607, #13105, #4951, #6740, #8412, #6631, #17822, #11632, #7987, #13000, #3389, #14468, #456, #1817, #147, #3279, #16249, #3489, #45, #8299, #6533, #19508, #8104, #11438, #19298, #9865, #1918, #14673, #8203, #5255, #12794, #11330, #17718, #5159, #19196, #18022, #9767, #3584, #17917, #9965, #3693 ),
 ( #10077, #16451, #4849, #11230, #2429, #7352, #3799, #18233, #2222, #7248, #4001, #10275, #654, #5678, #12152, #2125, #15083, #15188, #13610, #15285, #13514, #19701, #19916, #4106, #7043, #19816, #8821, #6933, #8506, #12050, #16546, #18134, #13714, #11842, #13411, #16644, #18337, #14877, #10588, #5470, #3896, #18543, #865, #18445, #8606, #2323, #8917, #10176, #5570, #11941, #10386, #20014, #10489, #8712, #16758, #16859, #765, #20121, #2526, #5783, #4206, #963, #554, #13300, #5364, #14977, #11742, #7151, #4419, #4310, #5984, #17172, #1277, #6095, #4720, #20221, #20321, #5882, #12557, #10903, #2945, #16956, #20436, #9126, #10695, #4611 ),
 ( #12252, #9433, #2635, #15495, #14131, #2848, #9223, #18644, #7657, #15593, #2746, #11004, #12359, #10803, #6287, #18857, #7862, #17373, #18956, #17265, #12659, #4518, #15806, #17066, #9022, #20632, #3059, #7766, #1178, #15393, #20536, #12463, #1483, #14027, #18753, #13919, #7458, #9325, #15701, #1385, #1078, #13819, #6189, #14224, #19062, #7556, #11410, #19578, #123, #3562, #14, #218, #9530, #12972, #17689, #11109, #14754, #6402, #15902, #17480, #17895, #1581, #3462, #16013, #12769, #19272, #3158, #4826, #19482, #19172, #3360, #11207, #16227, #8076, #9840, #11514, #9740, #6604, #432, #7957, #16124, #6508, #17580, #9942, #4924, #3254 ),
 ( #14546, #1894, #6811, #8275, #9628, #19375, #16323, #11303, #1691, #12870, #1791, #8178, #5030, #14330, #14441, #17796, #14646, #6711, #326, #13080, #5136, #1997, #8382, #13180, #13587, #3974, #2101, #11817, #529, #18420, #11610, #3774, #2407, #18210, #3872, #8484, #16618, #5448, #11715, #19988, #631, #19790, #15263, #7128, #16837, #5652, #841, #5547, #941, #13490, #4082, #19676, #17996, #8897, #7224, #16734, #10153, #3667, #8798, #15060, #10470, #10250, #7019, #2198, #16424, #2298, #8689, #8581, #10051, #14853, #11917, #742, #19891, #2503, #18308, #13689, #14950, #7328, #6907, #10360, #13275, #15166, #12024, #5232, #5340, #18111 ),
 ( #16524, #13386, #5863, #18624, #2827, #18524, #20098, #6072, #7436, #9103, #12232, #20410, #75, #5761, #13900, #7632, #14005, #9303, #12334, #12132, #2722, #4184, #15475, #4397, #20300, #1258, #16936, #5960, #18730, #6461, #1640, #4284, #17150, #7534, #10569, #15370, #15679, #1157, #10780, #13798, #2608, #8999, #1054, #9200, #20202, #12440, #10671, #15574, #18834, #17044, #17245, #4497, #2925, #10882, #8021, #14391, #3735, #7188, #16799, #10430, #11780, #5723, #19952, #8757, #8953, #901, #16897, #3934, #2568, #12093, #15130, #4145, #16489, #2468, #2259, #19748, #5505, #10115, #18170, #18484, #5406, #10320, #6977, #8859, #15020, #15227 ),
 ( #1008, #18069, #2369, #13451, #3835, #10528, #11880, #10214, #13347, #5610, #13551, #2161, #18384, #16582, #7286, #8646, #804, #700, #11984, #4046, #13648, #18272, #15327, #8545, #7086, #19855, #16690, #14915, #7399, #20060, #13760, #20163, #5824, #592, #3173, #17493, #3072, #3377, #232, #7878, #7975, #12784, #17705, #14145, #14237, #12572, #17597, #14348, #1595, #12191, #15716, #15819, #1399, #8092, #6420, #19186, #18583, #15918, #4627, #6203, #138, #11221, #9340, #19079, #7782, #4941, #4532, #11021, #9646, #4735, #11123, #20552, #9547, #12676, #18972, #6522, #20645, #6303, #1808, #32, #9756, #12885, #14458, #4840, #8193, #3270 ),
 ( #10916, #16032, #1708, #16141, #19288, #17390, #11321, #14559, #17279, #2963, #9448, #1497, #14770, #17812, #13402, #3887, #19808, #1906, #11835, #2014, #2214, #16240, #13195, #19693, #5050, #11624, #19392, #8704, #19593, #6923, #12991, #16442, #5356, #11734, #344, #14966, #8499, #18014, #18225, #10169, #5463, #5247, #10267, #647, #3685, #16634, #11427, #18126, #11528, #8289, #447, #3478, #6728, #7035, #14664, #10069, #13095, #3792, #3576, #16539, #2314, #2117, #14869, #15075, #6620, #544, #8403, #19498, #9855, #6826, #5150, #17909, #13292, #8596, #9955, #16340, #15331, #2571, #1011, #17112, #7704, #2683, #8956, #4249, #15441, #20265 ) ),
 .UNSPECIFIED., .T., .F., .T. ) 
 B_SPLINE_SURFACE_WITH_KNOTS ( ( 4, 3, 4 ),
 ( 4, 2, 2, 2, 2, 2, 2, 2, 2, 2, 2, 2, 2, 2, 2, 2, 2, 2, 2, 2, 2, 2, 2, 2, 2, 2, 2, 2, 2, 2, 2, 2, 2, 2, 2, 2, 2, 2, 2, 2, 2, 2, 4 ),
 ( 0.000000000000000000, 0.5000000000000000000, 1.000000000000000000 ),
 ( 0.000000000000000000, 0.03481082764294501225, 0.05122453910963481460, 0.05943139484297971231, 0.06353482270965216117, 0.06763825057632461002, 0.07081696859385246123, 0.07399568661138031245, 0.08035312264643601488, 0.09306799471654741973, 0.1057828667866588246, 0.1121403028217145270, 0.1153190208392423644, 0.1184977388567702156, 0.1214804596100246270, 0.1244631803632790246, 0.1304286218697878197, 0.1423595048828054099, 0.1662212709088405904, 0.2139448029609109514, 0.3093918670650516733, 0.5002859952733331728, 0.6911801234816146167, 0.7866271875857553386, 0.8343507196378256996, 0.8582124856638608801, 0.8701433686768784703, 0.8761088101833873765, 0.8790915309366418295, 0.8820742516898961716, 0.8853411830926052328, 0.8886081144953141830, 0.8951419773007323055, 0.9082097029115685505, 0.9212774285224047954, 0.9278112913278229179, 0.9310782227305318681, 0.9343451541332409294, 0.9384485819999133227, 0.9425520098665858271, 0.9507588655999306138, 0.9671725770666204092, 1.000000000000000000 ),
 .UNSPECIFIED. ) 
 GEOMETRIC_REPRESENTATION_ITEM ( )  RATIONAL_B_SPLINE_SURFACE ( (
 ( 1.000000000000000000, 1.000000000000000000, 1.000000000000000000, 1.000000000000000000, 1.000000000000000000, 1.000000000000000000, 1.000000000000000000, 1.000000000000000000, 1.000000000000000000, 1.000000000000000000, 1.000000000000000000, 1.000000000000000000, 1.000000000000000000, 1.000000000000000000, 1.000000000000000000, 1.000000000000000000, 1.000000000000000000, 1.000000000000000000, 1.000000000000000000, 1.000000000000000000, 1.000000000000000000, 1.000000000000000000, 1.000000000000000000, 1.000000000000000000, 1.000000000000000000, 1.000000000000000000, 1.000000000000000000, 1.000000000000000000, 1.000000000000000000, 1.000000000000000000, 1.000000000000000000, 1.000000000000000000, 1.000000000000000000, 1.000000000000000000, 1.000000000000000000, 1.000000000000000000, 1.000000000000000000, 1.000000000000000000, 1.000000000000000000, 1.000000000000000000, 1.000000000000000000, 1.000000000000000000, 1.000000000000000000, 1.000000000000000000, 1.000000000000000000, 1.000000000000000000, 1.000000000000000000, 1.000000000000000000, 1.000000000000000000, 1.000000000000000000, 1.000000000000000000, 1.000000000000000000, 1.000000000000000000, 1.000000000000000000, 1.000000000000000000, 1.000000000000000000, 1.000000000000000000, 1.000000000000000000, 1.000000000000000000, 1.000000000000000000, 1.000000000000000000, 1.000000000000000000, 1.000000000000000000, 1.000000000000000000, 1.000000000000000000, 1.000000000000000000, 1.000000000000000000, 1.000000000000000000, 1.000000000000000000, 1.000000000000000000, 1.000000000000000000, 1.000000000000000000, 1.000000000000000000, 1.000000000000000000, 1.000000000000000000, 1.000000000000000000, 1.000000000000000000, 1.000000000000000000, 1.000000000000000000, 1.000000000000000000, 1.000000000000000000, 1.000000000000000000, 1.000000000000000000, 1.000000000000000000, 1.000000000000000000, 1.000000000000000000),
 ( 0.3333333333333333703, 0.3333333333333333703, 0.3333333333333333703, 0.3333333333333333703, 0.3333333333333333703, 0.3333333333333333703, 0.3333333333333333703, 0.3333333333333333703, 0.3333333333333333703, 0.3333333333333333703, 0.3333333333333333703, 0.3333333333333333703, 0.3333333333333333703, 0.3333333333333333703, 0.3333333333333333703, 0.3333333333333333703, 0.3333333333333333703, 0.3333333333333333703, 0.3333333333333333703, 0.3333333333333333703, 0.3333333333333333703, 0.3333333333333333703, 0.3333333333333333703, 0.3333333333333333703, 0.3333333333333333703, 0.3333333333333333703, 0.3333333333333333703, 0.3333333333333333703, 0.3333333333333333703, 0.3333333333333333703, 0.3333333333333333703, 0.3333333333333333703, 0.3333333333333333703, 0.3333333333333333703, 0.3333333333333333703, 0.3333333333333333703, 0.3333333333333333703, 0.3333333333333333703, 0.3333333333333333703, 0.3333333333333333703, 0.3333333333333333703, 0.3333333333333333703, 0.3333333333333333703, 0.3333333333333333703, 0.3333333333333333703, 0.3333333333333333703, 0.3333333333333333703, 0.3333333333333333703, 0.3333333333333333703, 0.3333333333333333703, 0.3333333333333333703, 0.3333333333333333703, 0.3333333333333333703, 0.3333333333333333703, 0.3333333333333333703, 0.3333333333333333703, 0.3333333333333333703, 0.3333333333333333703, 0.3333333333333333703, 0.3333333333333333703, 0.3333333333333333703, 0.3333333333333333703, 0.3333333333333333703, 0.3333333333333333703, 0.3333333333333333703, 0.3333333333333333703, 0.3333333333333333703, 0.3333333333333333703, 0.3333333333333333703, 0.3333333333333333703, 0.3333333333333333703, 0.3333333333333333703, 0.3333333333333333703, 0.3333333333333333703, 0.3333333333333333703, 0.3333333333333333703, 0.3333333333333333703, 0.3333333333333333703, 0.3333333333333333703, 0.3333333333333333703, 0.3333333333333333703, 0.3333333333333333703, 0.3333333333333333703, 0.3333333333333333703, 0.3333333333333333703, 0.3333333333333333703),
 ( 0.3333333333333333703, 0.3333333333333333703, 0.3333333333333333703, 0.3333333333333333703, 0.3333333333333333703, 0.3333333333333333703, 0.3333333333333333703, 0.3333333333333333703, 0.3333333333333333703, 0.3333333333333333703, 0.3333333333333333703, 0.3333333333333333703, 0.3333333333333333703, 0.3333333333333333703, 0.3333333333333333703, 0.3333333333333333703, 0.3333333333333333703, 0.3333333333333333703, 0.3333333333333333703, 0.3333333333333333703, 0.3333333333333333703, 0.3333333333333333703, 0.3333333333333333703, 0.3333333333333333703, 0.3333333333333333703, 0.3333333333333333703, 0.3333333333333333703, 0.3333333333333333703, 0.3333333333333333703, 0.3333333333333333703, 0.3333333333333333703, 0.3333333333333333703, 0.3333333333333333703, 0.3333333333333333703, 0.3333333333333333703, 0.3333333333333333703, 0.3333333333333333703, 0.3333333333333333703, 0.3333333333333333703, 0.3333333333333333703, 0.3333333333333333703, 0.3333333333333333703, 0.3333333333333333703, 0.3333333333333333703, 0.3333333333333333703, 0.3333333333333333703, 0.3333333333333333703, 0.3333333333333333703, 0.3333333333333333703, 0.3333333333333333703, 0.3333333333333333703, 0.3333333333333333703, 0.3333333333333333703, 0.3333333333333333703, 0.3333333333333333703, 0.3333333333333333703, 0.3333333333333333703, 0.3333333333333333703, 0.3333333333333333703, 0.3333333333333333703, 0.3333333333333333703, 0.3333333333333333703, 0.3333333333333333703, 0.3333333333333333703, 0.3333333333333333703, 0.3333333333333333703, 0.3333333333333333703, 0.3333333333333333703, 0.3333333333333333703, 0.3333333333333333703, 0.3333333333333333703, 0.3333333333333333703, 0.3333333333333333703, 0.3333333333333333703, 0.3333333333333333703, 0.3333333333333333703, 0.3333333333333333703, 0.3333333333333333703, 0.3333333333333333703, 0.3333333333333333703, 0.3333333333333333703, 0.3333333333333333703, 0.3333333333333333703, 0.3333333333333333703, 0.3333333333333333703, 0.3333333333333333703),
 ( 1.000000000000000000, 1.000000000000000000, 1.000000000000000000, 1.000000000000000000, 1.000000000000000000, 1.000000000000000000, 1.000000000000000000, 1.000000000000000000, 1.000000000000000000, 1.000000000000000000, 1.000000000000000000, 1.000000000000000000, 1.000000000000000000, 1.000000000000000000, 1.000000000000000000, 1.000000000000000000, 1.000000000000000000, 1.000000000000000000, 1.000000000000000000, 1.000000000000000000, 1.000000000000000000, 1.000000000000000000, 1.000000000000000000, 1.000000000000000000, 1.000000000000000000, 1.000000000000000000, 1.000000000000000000, 1.000000000000000000, 1.000000000000000000, 1.000000000000000000, 1.000000000000000000, 1.000000000000000000, 1.000000000000000000, 1.000000000000000000, 1.000000000000000000, 1.000000000000000000, 1.000000000000000000, 1.000000000000000000, 1.000000000000000000, 1.000000000000000000, 1.000000000000000000, 1.000000000000000000, 1.000000000000000000, 1.000000000000000000, 1.000000000000000000, 1.000000000000000000, 1.000000000000000000, 1.000000000000000000, 1.000000000000000000, 1.000000000000000000, 1.000000000000000000, 1.000000000000000000, 1.000000000000000000, 1.000000000000000000, 1.000000000000000000, 1.000000000000000000, 1.000000000000000000, 1.000000000000000000, 1.000000000000000000, 1.000000000000000000, 1.000000000000000000, 1.000000000000000000, 1.000000000000000000, 1.000000000000000000, 1.000000000000000000, 1.000000000000000000, 1.000000000000000000, 1.000000000000000000, 1.000000000000000000, 1.000000000000000000, 1.000000000000000000, 1.000000000000000000, 1.000000000000000000, 1.000000000000000000, 1.000000000000000000, 1.000000000000000000, 1.000000000000000000, 1.000000000000000000, 1.000000000000000000, 1.000000000000000000, 1.000000000000000000, 1.000000000000000000, 1.000000000000000000, 1.000000000000000000, 1.000000000000000000, 1.000000000000000000),
 ( 0.3333333333333333703, 0.3333333333333333703, 0.3333333333333333703, 0.3333333333333333703, 0.3333333333333333703, 0.3333333333333333703, 0.3333333333333333703, 0.3333333333333333703, 0.3333333333333333703, 0.3333333333333333703, 0.3333333333333333703, 0.3333333333333333703, 0.3333333333333333703, 0.3333333333333333703, 0.3333333333333333703, 0.3333333333333333703, 0.3333333333333333703, 0.3333333333333333703, 0.3333333333333333703, 0.3333333333333333703, 0.3333333333333333703, 0.3333333333333333703, 0.3333333333333333703, 0.3333333333333333703, 0.3333333333333333703, 0.3333333333333333703, 0.3333333333333333703, 0.3333333333333333703, 0.3333333333333333703, 0.3333333333333333703, 0.3333333333333333703, 0.3333333333333333703, 0.3333333333333333703, 0.3333333333333333703, 0.3333333333333333703, 0.3333333333333333703, 0.3333333333333333703, 0.3333333333333333703, 0.3333333333333333703, 0.3333333333333333703, 0.3333333333333333703, 0.3333333333333333703, 0.3333333333333333703, 0.3333333333333333703, 0.3333333333333333703, 0.3333333333333333703, 0.3333333333333333703, 0.3333333333333333703, 0.3333333333333333703, 0.3333333333333333703, 0.3333333333333333703, 0.3333333333333333703, 0.3333333333333333703, 0.3333333333333333703, 0.3333333333333333703, 0.3333333333333333703, 0.3333333333333333703, 0.3333333333333333703, 0.3333333333333333703, 0.3333333333333333703, 0.3333333333333333703, 0.3333333333333333703, 0.3333333333333333703, 0.3333333333333333703, 0.3333333333333333703, 0.3333333333333333703, 0.3333333333333333703, 0.3333333333333333703, 0.3333333333333333703, 0.3333333333333333703, 0.3333333333333333703, 0.3333333333333333703, 0.3333333333333333703, 0.3333333333333333703, 0.3333333333333333703, 0.3333333333333333703, 0.3333333333333333703, 0.3333333333333333703, 0.3333333333333333703, 0.3333333333333333703, 0.3333333333333333703, 0.3333333333333333703, 0.3333333333333333703, 0.3333333333333333703, 0.3333333333333333703, 0.3333333333333333703),
 ( 0.3333333333333333703, 0.3333333333333333703, 0.3333333333333333703, 0.3333333333333333703, 0.3333333333333333703, 0.3333333333333333703, 0.3333333333333333703, 0.3333333333333333703, 0.3333333333333333703, 0.3333333333333333703, 0.3333333333333333703, 0.3333333333333333703, 0.3333333333333333703, 0.3333333333333333703, 0.3333333333333333703, 0.3333333333333333703, 0.3333333333333333703, 0.3333333333333333703, 0.3333333333333333703, 0.3333333333333333703, 0.3333333333333333703, 0.3333333333333333703, 0.3333333333333333703, 0.3333333333333333703, 0.3333333333333333703, 0.3333333333333333703, 0.3333333333333333703, 0.3333333333333333703, 0.3333333333333333703, 0.3333333333333333703, 0.3333333333333333703, 0.3333333333333333703, 0.3333333333333333703, 0.3333333333333333703, 0.3333333333333333703, 0.3333333333333333703, 0.3333333333333333703, 0.3333333333333333703, 0.3333333333333333703, 0.3333333333333333703, 0.3333333333333333703, 0.3333333333333333703, 0.3333333333333333703, 0.3333333333333333703, 0.3333333333333333703, 0.3333333333333333703, 0.3333333333333333703, 0.3333333333333333703, 0.3333333333333333703, 0.3333333333333333703, 0.3333333333333333703, 0.3333333333333333703, 0.3333333333333333703, 0.3333333333333333703, 0.3333333333333333703, 0.3333333333333333703, 0.3333333333333333703, 0.3333333333333333703, 0.3333333333333333703, 0.3333333333333333703, 0.3333333333333333703, 0.3333333333333333703, 0.3333333333333333703, 0.3333333333333333703, 0.3333333333333333703, 0.3333333333333333703, 0.3333333333333333703, 0.3333333333333333703, 0.3333333333333333703, 0.3333333333333333703, 0.3333333333333333703, 0.3333333333333333703, 0.3333333333333333703, 0.3333333333333333703, 0.3333333333333333703, 0.3333333333333333703, 0.3333333333333333703, 0.3333333333333333703, 0.3333333333333333703, 0.3333333333333333703, 0.3333333333333333703, 0.3333333333333333703, 0.3333333333333333703, 0.3333333333333333703, 0.3333333333333333703, 0.3333333333333333703),
 ( 1.000000000000000000, 1.000000000000000000, 1.000000000000000000, 1.000000000000000000, 1.000000000000000000, 1.000000000000000000, 1.000000000000000000, 1.000000000000000000, 1.000000000000000000, 1.000000000000000000, 1.000000000000000000, 1.000000000000000000, 1.000000000000000000, 1.000000000000000000, 1.000000000000000000, 1.000000000000000000, 1.000000000000000000, 1.000000000000000000, 1.000000000000000000, 1.000000000000000000, 1.000000000000000000, 1.000000000000000000, 1.000000000000000000, 1.000000000000000000, 1.000000000000000000, 1.000000000000000000, 1.000000000000000000, 1.000000000000000000, 1.000000000000000000, 1.000000000000000000, 1.000000000000000000, 1.000000000000000000, 1.000000000000000000, 1.000000000000000000, 1.000000000000000000, 1.000000000000000000, 1.000000000000000000, 1.000000000000000000, 1.000000000000000000, 1.000000000000000000, 1.000000000000000000, 1.000000000000000000, 1.000000000000000000, 1.000000000000000000, 1.000000000000000000, 1.000000000000000000, 1.000000000000000000, 1.000000000000000000, 1.000000000000000000, 1.000000000000000000, 1.000000000000000000, 1.000000000000000000, 1.000000000000000000, 1.000000000000000000, 1.000000000000000000, 1.000000000000000000, 1.000000000000000000, 1.000000000000000000, 1.000000000000000000, 1.000000000000000000, 1.000000000000000000, 1.000000000000000000, 1.000000000000000000, 1.000000000000000000, 1.000000000000000000, 1.000000000000000000, 1.000000000000000000, 1.000000000000000000, 1.000000000000000000, 1.000000000000000000, 1.000000000000000000, 1.000000000000000000, 1.000000000000000000, 1.000000000000000000, 1.000000000000000000, 1.000000000000000000, 1.000000000000000000, 1.000000000000000000, 1.000000000000000000, 1.000000000000000000, 1.000000000000000000, 1.000000000000000000, 1.000000000000000000, 1.000000000000000000, 1.000000000000000000, 1.000000000000000000) ) ) 
 REPRESENTATION_ITEM ( '' )  SURFACE ( )  );
#8428=CARTESIAN_POINT ( 'NONE',  ( -7.090308582316794173, -21.32581373872472597, 1.729004561291657582 ) ) ;
#8429=CARTESIAN_POINT ( 'NONE',  ( -3.343476823822036259, -9.987837386737346890, 2.789442121235767402 ) ) ;
#8431=CARTESIAN_POINT ( 'NONE',  ( -12.78345773956433895, -11.49788415197707181, 4.924178440007425550 ) ) ;
#8432=CARTESIAN_POINT ( 'NONE',  ( -6.621558582316794173, -23.74999999999999645, 3.550687472877651629 ) ) ;
#8433=CARTESIAN_POINT ( 'NONE',  ( -7.659691417683177406, -22.67418626127524917, 1.729004561291651809 ) ) ;
#8435=CARTESIAN_POINT ( 'NONE',  ( 13.83051420738022763, 3.503467472703414742, 5.232249963382380464 ) ) ;
#8443=CARTESIAN_POINT ( 'NONE',  ( -13.39482594849551944, -19.24878960097397140, 5.493002502378098839 ) ) ;
#8445=CARTESIAN_POINT ( 'NONE',  ( 5.784691417683177406, -23.77099543870834353, 4.174186261275251830 ) ) ;
#8452=CARTESIAN_POINT ( 'NONE',  ( 7.847191417683176518, -21.22443879296941915, 1.770995438708345748 ) ) ;
#8454=CARTESIAN_POINT ( 'NONE',  ( -4.472191417683177406, -23.72900456129165292, 2.724438792969417822 ) ) ;
#8455=CARTESIAN_POINT ( 'NONE',  ( -7.277808582316795061, -19.52099543870833642, 2.413778621189609286 ) ) ;
#8457=CARTESIAN_POINT ( 'NONE',  ( 12.62499979224180180, -20.25001049178813162, 4.458178821399696012 ) ) ;
#8458=CARTESIAN_POINT ( 'NONE',  ( -13.14123030749026277, 5.069630528265579805, 6.418963484850015000 ) ) ;
#8463=VERTEX_POINT ( 'NONE', #10083 ) ;
#8466=CARTESIAN_POINT ( 'NONE',  ( 12.66943601481756687, -20.06596378382619150, 3.544869486356359456 ) ) ;
#8467=EDGE_LOOP ( 'NONE', ( #12493, #16157, #12641, #3870, #5865 ) ) ;
#8469=CARTESIAN_POINT ( 'NONE',  ( 13.00900269284621302, -0.8578640112522492034, 5.903024842915844062 ) ) ;
#8473=CARTESIAN_POINT ( 'NONE',  ( 12.63943061533661982, -19.52125392549825733, 5.470334935344855154 ) ) ;
#8475=CARTESIAN_POINT ( 'NONE',  ( 11.21530858231679595, -24.52099543870834708, 2.515153566944913432 ) ) ;
#8476=CARTESIAN_POINT ( 'NONE',  ( -12.62499979224180180, -20.25001049178813162, 4.458178821399696012 ) ) ;
#8477=CARTESIAN_POINT ( 'NONE',  ( -6.902808582316795949, -23.08622137881038938, 1.020995438708339309 ) ) ;
#8480=CARTESIAN_POINT ( 'NONE',  ( 9.152808582316795949, -21.53509896474924901, 4.479004561291659137 ) ) ;
#8481=CARTESIAN_POINT ( 'NONE',  ( -7.940941417683176518, -20.72672167713052715, 2.298404588716546293 ) ) ;
#8484=CARTESIAN_POINT ( 'NONE',  ( 13.41341218697771609, -18.31018455762212227, 5.513179699623425023 ) ) ;
#8492=CARTESIAN_POINT ( 'NONE',  ( 13.39662663169496781, -19.15785509940297615, 5.494950532956567102 ) ) ;
#8494=CARTESIAN_POINT ( 'NONE',  ( 1.884282074604925583, -8.375506800461993251, 2.375363417140690547 ) ) ;
#8496=CARTESIAN_POINT ( 'NONE',  ( -12.62503976493681535, -19.49799187068907713, 4.533161381885315144 ) ) ;
#8497=CARTESIAN_POINT ( 'NONE',  ( 5.496558582316794173, -22.05068747287764452, 1.749999999999998446 ) ) ;
#8499=CARTESIAN_POINT ( 'NONE',  ( 12.66849571425264287, -18.05346643024382303, 5.533233176248494978 ) ) ;
#8500=CARTESIAN_POINT ( 'NONE',  ( -1.904508877737772998, -9.138371295333994837, 2.378667276417936627 ) ) ;
#8501=CARTESIAN_POINT ( 'NONE',  ( 8.684058582316795949, -21.32873467460644079, 2.757051763020455404 ) ) ;
#8502=CARTESIAN_POINT ( 'NONE',  ( 10.47219141768317563, -23.72900456129165292, 2.724438792969417822 ) ) ;
#8503=CARTESIAN_POINT ( 'NONE',  ( -9.902808582316795949, -22.46490103525074034, 2.520995438708341307 ) ) ;
#8505=CARTESIAN_POINT ( 'NONE',  ( 12.63806878948643231, -20.34002613093225520, 5.891296472647073124 ) ) ;
#8506=CARTESIAN_POINT ( 'NONE',  ( 12.63118877378512828, -19.18746692385052555, 4.758813856674282583 ) ) ;
#8516=CARTESIAN_POINT ( 'NONE',  ( 1.668644041176298387, -9.864915931696323526, 2.372643470467795890 ) ) ;
#8521=CARTESIAN_POINT ( 'NONE',  ( -2.513306525444908512, -9.622685169956881168, 2.503048754562789746 ) ) ;
#8522=CARTESIAN_POINT ( 'NONE',  ( -5.965308582316793284, -20.22900456129164937, 4.174186261275266929 ) ) ;
#8523=CARTESIAN_POINT ( 'NONE',  ( -0.5631383031621635116, -8.364917468222230923, 2.372643865078341019 ) ) ;
#8525=CARTESIAN_POINT ( 'NONE',  ( -13.64827103573800571, -5.699812695207630675, 5.034333296717131034 ) ) ;
#8526=CARTESIAN_POINT ( 'NONE',  ( -4.746558582316793284, -21.94931252712234482, 5.250000000000000888 ) ) ;
#8527=CARTESIAN_POINT ( 'NONE',  ( -9.909691417683179182, -21.32581373872474373, 5.270995438708348857 ) ) ;
#8529=CARTESIAN_POINT ( 'NONE',  ( 13.84501469867365131, 4.235742283194553259, 3.333333333332063386 ) ) ;
#8536=CARTESIAN_POINT ( 'NONE',  ( -13.37500000000002132, -20.25000000000274269, 4.083333333315724012 ) ) ;
#8537=B_SPLINE_CURVE_WITH_KNOTS ( 'NONE', 3,
 ( #16349, #3490, #16250, #1919, #10078, #16452, #19703, #2126, #14878, #11743 ),
 .UNSPECIFIED., .F., .F.,
 ( 4, 2, 2, 2, 4 ),
 ( 0.001177954577779514490, 0.001472373510017591655, 0.001766792442255668821, 0.002061211374493746203, 0.002355630306731823151 ),
 .UNSPECIFIED. ) ;
#8539=CARTESIAN_POINT ( 'NONE',  ( 3.944195004867014909, -21.61378581760806128, 5.207602947182413011 ) ) ;
#8542=CARTESIAN_POINT ( 'NONE',  ( 3.343476823822036259, -9.987837386737346890, 2.789442121235767402 ) ) ;
#8543=CARTESIAN_POINT ( 'NONE',  ( -6.527808582316794173, -23.72900456129165292, 4.275561207030568411 ) ) ;
#8544=EDGE_CURVE ( 'NONE', #10614, #12628, #8392, .T. ) ;
#8545=CARTESIAN_POINT ( 'NONE',  ( 12.65346245025441263, -19.56264626215117275, 6.228892365149262922 ) ) ;
#8547=CARTESIAN_POINT ( 'NONE',  ( 9.534691417683177406, -20.22900456129164581, 2.825813738724747726 ) ) ;
#8549=CARTESIAN_POINT ( 'NONE',  ( -4.847191417683177406, -21.53509896474923835, 2.520995438708346192 ) ) ;
#8550=CARTESIAN_POINT ( 'NONE',  ( -6.809058582316796837, -23.80360840875935935, 1.768074502826626260 ) ) ;
#8552=CARTESIAN_POINT ( 'NONE',  ( 12.62500016093973620, -20.24999187254239175, 4.532396751752561848 ) ) ;
#8553=CARTESIAN_POINT ( 'NONE',  ( -12.62499999999998579, -20.24999999999999289, 3.666666666666653640 ) ) ;
#8561=CARTESIAN_POINT ( 'NONE',  ( 13.33984198047847514, -20.08950154656911380, 3.453859469323321552 ) ) ;
#8562=VERTEX_POINT ( 'NONE', #14338 ) ;
#8564=CARTESIAN_POINT ( 'NONE',  ( 13.12529397354238192, 5.014845663890295846, 4.166666666666749563 ) ) ;
#8565=CARTESIAN_POINT ( 'NONE',  ( -1.819865260185086875, -9.122006307963404836, 1.624464420737683046 ) ) ;
#8568=CARTESIAN_POINT ( 'NONE',  ( 13.12529397354238192, 5.014845663890295846, 3.666666666666500873 ) ) ;
#8569=CARTESIAN_POINT ( 'NONE',  ( 4.687312169500631676, -21.54001800463478133, 5.087297191110758732 ) ) ;
#8571=CARTESIAN_POINT ( 'NONE',  ( 10.84030858231679595, -22.98484643305508612, 6.020995438708344416 ) ) ;
#8572=CARTESIAN_POINT ( 'NONE',  ( -13.11465082267961968, 3.727366545318180791, 6.751662912489328150 ) ) ;
#8573=CARTESIAN_POINT ( 'NONE',  ( -8.222191417683175629, -19.52099543870834353, 4.586221378810406257 ) ) ;
#8577=CARTESIAN_POINT ( 'NONE',  ( 7.934058582316796837, -22.67126532539354855, 4.242948236979545484 ) ) ;
#8581=CARTESIAN_POINT ( 'NONE',  ( 13.87066368810231154, 4.781016249162736820, 5.617237349937618696 ) ) ;
#8589=CARTESIAN_POINT ( 'NONE',  ( 13.85788212999909419, 4.135547564954428879, 5.982801014393342776 ) ) ;
#8591=CARTESIAN_POINT ( 'NONE',  ( 0.2815691515810352374, -8.364917468222230923, 2.372643865078523540 ) ) ;
#8593=CARTESIAN_POINT ( 'NONE',  ( -13.06641424290328501, 2.791419266617020334, 5.231470106674447784 ) ) ;
#8594=CARTESIAN_POINT ( 'NONE',  ( 6.152808582316794173, -21.22443879296942626, 5.229004561291660025 ) ) ;
#8596=CARTESIAN_POINT ( 'NONE',  ( 13.12526104302547836, 5.013182672784613381, 5.066812735559260261 ) ) ;
#8598=CARTESIAN_POINT ( 'NONE',  ( -0.9854920305337621089, -9.114917468222230923, 2.372643865078341019 ) ) ;
#8599=CARTESIAN_POINT ( 'NONE',  ( 10.84030858231679595, -22.36352608949544418, 4.520995438708343528 ) ) ;
#8601=CARTESIAN_POINT ( 'NONE',  ( 7.190941417683176518, -23.27327832286946219, 4.701595411283453707 ) ) ;
#8602=CARTESIAN_POINT ( 'NONE',  ( -9.434058582316794173, -23.20159541128345992, 4.773278322869455970 ) ) ;
#8604=CARTESIAN_POINT ( 'NONE',  ( 12.70700162295422864, -16.85891804079483691, 6.308954579156044851 ) ) ;
#8606=CARTESIAN_POINT ( 'NONE',  ( 12.93692567357942202, -3.747753484270499591, 5.090845106672844622 ) ) ;
#8615=CARTESIAN_POINT ( 'NONE',  ( -3.944195004867014909, -21.58936506995667770, 5.302691919372072960 ) ) ;
#8616=CARTESIAN_POINT ( 'NONE',  ( 1.743623630681728542, -9.116095536440919744, 2.372946416531167557 ) ) ;
#8623=CARTESIAN_POINT ( 'NONE',  ( -9.621558582316794173, -23.74999999999999645, 3.550687472877651629 ) ) ;
#8625=CARTESIAN_POINT ( 'NONE',  ( -3.173374397671306912, -9.279487642487616483, 2.607523756204581211 ) ) ;
#8627=CARTESIAN_POINT ( 'NONE',  ( -13.09560264575884503, 4.265433610975056133, 3.333333333333364568 ) ) ;
#8628=CARTESIAN_POINT ( 'NONE',  ( -4.934058582316793284, -23.20159541128345992, 4.773278322869455970 ) ) ;
#8629=CARTESIAN_POINT ( 'NONE',  ( -8.690941417683177406, -23.27327832286946219, 4.701595411283453707 ) ) ;
#8630=ORIENTED_EDGE ( 'NONE', *, *, #15176, .F. ) ;
#8631=CARTESIAN_POINT ( 'NONE',  ( 13.84504075139246915, 3.487057945321567765, 5.981929699623240282 ) ) ;
#8638=CARTESIAN_POINT ( 'NONE',  ( -13.37561105820882013, -20.21914156045197686, 4.753815841436231260 ) ) ;
#8640=CARTESIAN_POINT ( 'NONE',  ( 6.253441417683176518, -21.94931252712233061, 1.749999999999998446 ) ) ;
#8642=CARTESIAN_POINT ( 'NONE',  ( -13.87470602645761808, 4.985154336109792972, 4.000000000000000000 ) ) ;
#8643=CARTESIAN_POINT ( 'NONE',  ( 3.996922828336520794, -14.62728872172488437, 3.980945906412841850 ) ) ;
#8644=CARTESIAN_POINT ( 'NONE',  ( -7.652808582316794173, -21.22443879296942626, 5.229004561291660025 ) ) ;
#8646=CARTESIAN_POINT ( 'NONE',  ( 12.62608183053121458, -20.94536755816881168, 4.949360998036265613 ) ) ;
#8649=EDGE_CURVE ( 'NONE', #8562, #17561, #16132, .T. ) ;
#8650=CARTESIAN_POINT ( 'NONE',  ( 4.940941417683177406, -20.72672167713052715, 2.298404588716546293 ) ) ;
#8651=CARTESIAN_POINT ( 'NONE',  ( -12.62499999999998224, -20.24999999999998934, 4.291666666666698937 ) ) ;
#8652=CARTESIAN_POINT ( 'NONE',  ( -5.503441417683177406, -22.05068747287766229, 4.499999999999999112 ) ) ;
#8653=CARTESIAN_POINT ( 'NONE',  ( -5.777808582316795949, -19.52099543870833642, 2.413778621189609286 ) ) ;
#8655=CARTESIAN_POINT ( 'NONE',  ( 13.12529397354238192, 5.014845663890295846, 4.833333333333344584 ) ) ;
#8656=CARTESIAN_POINT ( 'NONE',  ( -12.64511805349267526, -19.23403829861753422, 5.507852591554869726 ) ) ;
#8668=DIRECTION ( 'NONE',  ( 0.000000000000000000, -0.2487476929738665354, -0.9685683172808094987 ) ) ;
#8669=CARTESIAN_POINT ( 'NONE',  ( 12.79798428357658047, -11.51429367935891790, 5.673858176248284479 ) ) ;
#8670=CARTESIAN_POINT ( 'NONE',  ( -2.739050625766161762, -9.875938058683834342, 1.818089155622620412 ) ) ;
#8676=CARTESIAN_POINT ( 'NONE',  ( 10.94094141768317741, -20.19639159124061933, 1.768074502826635586 ) ) ;
#8677=CARTESIAN_POINT ( 'NONE',  ( -13.12529397354238192, 5.014845663890295846, 4.916666666666650087 ) ) ;
#8678=CARTESIAN_POINT ( 'NONE',  ( -5.972191417683178294, -24.47900456129165292, 2.413778621189595963 ) ) ;
#8683=CARTESIAN_POINT ( 'NONE',  ( -13.83065313257865370, 2.760483195222930952, 5.966304699623404595 ) ) ;
#8685=CARTESIAN_POINT ( 'NONE',  ( 10.18405858231679595, -21.32873467460644079, 2.757051763020455404 ) ) ;
#8686=CARTESIAN_POINT ( 'NONE',  ( 4.687312169500630787, -21.51559725698340131, 5.182386163300424009 ) ) ;
#8689=CARTESIAN_POINT ( 'NONE',  ( 13.86693669322925260, 4.592803008081209448, 5.801483467520450077 ) ) ;
#8696=CARTESIAN_POINT ( 'NONE',  ( 13.38238173943565990, -19.87722215849730034, 5.285856107751903288 ) ) ;
#8698=CARTESIAN_POINT ( 'NONE',  ( 1.643076795806035717, -8.364903549957356077, 2.372640290589878909 ) ) ;
#8701=CARTESIAN_POINT ( 'NONE',  ( -12.62499999999998224, -19.49999999999991473, 4.333333333333343695 ) ) ;
#8704=CARTESIAN_POINT ( 'NONE',  ( 12.64511805349267526, -19.23403829861753422, 5.507852591554869726 ) ) ;
#8705=CARTESIAN_POINT ( 'NONE',  ( -2.436080212393455735, -9.483920418190111334, 2.467411194204634839 ) ) ;
#8706=CARTESIAN_POINT ( 'NONE',  ( 10.65280858231679595, -21.53509896474924901, 4.479004561291659137 ) ) ;
#8707=CARTESIAN_POINT ( 'NONE',  ( 10.94094141768317741, -20.72672167713052715, 2.298404588716546293 ) ) ;
#8708=CARTESIAN_POINT ( 'NONE',  ( -7.746558582316794173, -21.94931252712234482, 5.250000000000000888 ) ) ;
#8711=CARTESIAN_POINT ( 'NONE',  ( 13.15469878640066526, 5.749788713235649773, 5.232478742873432509 ) ) ;
#8712=CARTESIAN_POINT ( 'NONE',  ( 13.08439876642066935, 3.699637704240349656, 5.251001356674258602 ) ) ;
#8726=CARTESIAN_POINT ( 'NONE',  ( 2.645259258103298983, -10.28229522185712241, 2.672449792925449596 ) ) ;
#8734=CARTESIAN_POINT ( 'NONE',  ( -5.027808582316793284, -23.72900456129165647, 4.275561207030568411 ) ) ;
#8735=CARTESIAN_POINT ( 'NONE',  ( -3.594802210173583035, -11.77224174634763898, 3.247712807842289884 ) ) ;
#8737=CARTESIAN_POINT ( 'NONE',  ( -13.09560264576187905, 4.265433610975056133, 2.999999999999999556 ) ) ;
#8738=CARTESIAN_POINT ( 'NONE',  ( -7.840308582316794173, -22.67418626127525982, 5.270995438708342640 ) ) ;
#8739=CARTESIAN_POINT ( 'NONE',  ( 7.746558582316795949, -21.94931252712234127, 6.000000000000001776 ) ) ;
#8740=CARTESIAN_POINT ( 'NONE',  ( -7.472191417683177406, -22.97900456129165292, 3.035098964749240125 ) ) ;
#8742=CARTESIAN_POINT ( 'NONE',  ( 13.40382044110196347, -18.79456772435387890, 5.502763032956559108 ) ) ;
#8748=CARTESIAN_POINT ( 'NONE',  ( -13.37499999999998224, -20.24999999999998934, 4.166666666666636765 ) ) ;
#8755=CARTESIAN_POINT ( 'NONE',  ( 1.337453470010121714, -9.114917468222230923, 2.372643865078341019 ) ) ;
#8756=CARTESIAN_POINT ( 'NONE',  ( -6.152808582316794173, -21.22443879296942626, 5.229004561291660025 ) ) ;
#8757=CARTESIAN_POINT ( 'NONE',  ( 13.87824226375436965, 4.413734319597230282, 6.694665752684481497 ) ) ;
#8759=CARTESIAN_POINT ( 'NONE',  ( 5.878441417683177406, -23.74999999999999645, 3.449312527122335492 ) ) ;
#8762=CARTESIAN_POINT ( 'NONE',  ( -5.222191417683177406, -21.02099543870834353, 3.964901035250761208 ) ) ;
#8764=CARTESIAN_POINT ( 'NONE',  ( -11.97219141768317918, -24.47900456129165292, 2.413778621189595963 ) ) ;
#8766=CARTESIAN_POINT ( 'NONE',  ( 12.63958155142659834, -18.76363165295958524, 4.767928440007602298 ) ) ;
#8767=CARTESIAN_POINT ( 'NONE',  ( -13.12424783836753228, 4.962015837561366993, 5.328858059679200565 ) ) ;
#8780=CARTESIAN_POINT ( 'NONE',  ( -2.195822829018478473, -9.226849102155203042, 1.651390144731336163 ) ) ;
#8785=CARTESIAN_POINT ( 'NONE',  ( 9.347191417683177406, -20.91377862118959285, 1.020995438708345082 ) ) ;
#8786=CARTESIAN_POINT ( 'NONE',  ( -13.11514659413808737, 4.502403003978772134, 5.887634658581065494 ) ) ;
#8788=CARTESIAN_POINT ( 'NONE',  ( -8.597191417683177406, -23.08622137881040359, 5.979004561291654696 ) ) ;
#8790=CARTESIAN_POINT ( 'NONE',  ( 13.37155858231679417, -20.24999999999999289, 3.449312527122348371 ) ) ;
#8792=CARTESIAN_POINT ( 'NONE',  ( -13.45671396861735403, -16.87344458480707843, 6.294109435864141844 ) ) ;
#8794=CARTESIAN_POINT ( 'NONE',  ( 5.027808582316795949, -22.97900456129165647, 3.964901035250747885 ) ) ;
#8798=CARTESIAN_POINT ( 'NONE',  ( 13.85403523778986390, 3.941279508358651817, 5.991705257707216958 ) ) ;
#8805=CARTESIAN_POINT ( 'NONE',  ( 13.58606361274418184, -9.591287556442823714, 5.700679699621803209 ) ) ;
#8807=CARTESIAN_POINT ( 'NONE',  ( 3.336296098497695262, -9.936854405034125648, 2.776348673047012383 ) ) ;
#8809=CARTESIAN_POINT ( 'NONE',  ( -12.62958809053144549, -19.26830142816300295, 4.757073430686623361 ) ) ;
#8811=CARTESIAN_POINT ( 'NONE',  ( 11.30905858231679417, -23.27327832286945153, 2.298404588716537411 ) ) ;
#8812=CARTESIAN_POINT ( 'NONE',  ( -13.43273460392801155, -18.08440250163749496, 6.268067769197452677 ) ) ;
#8815=CARTESIAN_POINT ( 'NONE',  ( 12.80905858231679417, -23.27327832286945153, 2.298404588716537411 ) ) ;
#8816=CARTESIAN_POINT ( 'NONE',  ( 10.37844141768317741, -22.99999999999999645, 3.449312527122335048 ) ) ;
#8817=CARTESIAN_POINT ( 'NONE',  ( -9.809058582316794173, -23.27327832286945153, 2.298404588716537411 ) ) ;
#8820=CARTESIAN_POINT ( 'NONE',  ( 12.66383876651304874, -19.03864229108970463, 6.262079579155994224 ) ) ;
#8821=CARTESIAN_POINT ( 'NONE',  ( 12.62958809053144549, -19.26830142816300295, 4.757073430686623361 ) ) ;
#8831=CARTESIAN_POINT ( 'NONE',  ( 1.548630333695928396, -9.114917468222230923, 2.372643865078341019 ) ) ;
#8835=CARTESIAN_POINT ( 'NONE',  ( -12.05905858231679595, -20.19639159124062999, 5.231925497173373074 ) ) ;
#8836=CARTESIAN_POINT ( 'NONE',  ( -2.589709240944451096, -9.559844081062008669, 1.736909907557668165 ) ) ;
#8838=CARTESIAN_POINT ( 'NONE',  ( -13.37908441539295801, -19.29373702265862889, 4.740102594697787275 ) ) ;
#8839=CARTESIAN_POINT ( 'NONE',  ( -9.527808582316792396, -23.72900456129165647, 4.275561207030568411 ) ) ;
#8841=CARTESIAN_POINT ( 'NONE',  ( 7.840308582316795949, -22.98484643305508612, 6.020995438708344416 ) ) ;
#8842=CARTESIAN_POINT ( 'NONE',  ( -10.00344141768317741, -22.05068747287766229, 4.499999999999999112 ) ) ;
#8844=CARTESIAN_POINT ( 'NONE',  ( 13.37499999999998579, -20.24999999999999289, 3.666666666666653640 ) ) ;
#8850=CARTESIAN_POINT ( 'NONE',  ( -13.37515323800563039, -20.24226148071262799, 4.627790572011877934 ) ) ;
#8856=CARTESIAN_POINT ( 'NONE',  ( 3.317048600639548095, -9.800042196285016161, 2.741212564741740465 ) ) ;
#8859=CARTESIAN_POINT ( 'NONE',  ( 13.90439735423812273, 5.734566389025032684, 3.666666666666500873 ) ) ;
#8861=CARTESIAN_POINT ( 'NONE',  ( 10.47219141768317741, -22.97900456129165292, 3.035098964749240125 ) ) ;
#8863=CARTESIAN_POINT ( 'NONE',  ( -7.565941417683177406, -22.67126532539353789, 2.757051763020445634 ) ) ;
#8865=CARTESIAN_POINT ( 'NONE',  ( -8.034691417683175629, -19.47900456129164581, 2.515153566944927199 ) ) ;
#8867=CARTESIAN_POINT ( 'NONE',  ( 13.12526104302547836, 5.013182672784613381, 5.066812735559260261 ) ) ;
#8868=CARTESIAN_POINT ( 'NONE',  ( -13.12529397354238192, 5.014845663890295846, 3.666666666666500873 ) ) ;
#8879=CARTESIAN_POINT ( 'NONE',  ( -2.682825141213236009, -9.727160171598653093, 1.779880022082258373 ) ) ;
#8883=CARTESIAN_POINT ( 'NONE',  ( 6.059058582316795949, -20.19639159124062999, 5.231925497173373074 ) ) ;
#8884=CARTESIAN_POINT ( 'NONE',  ( -12.64511805349267526, -19.23403829861753422, 5.507852591554869726 ) ) ;
#8885=CARTESIAN_POINT ( 'NONE',  ( -6.722191417683176518, -19.52099543870834353, 4.586221378810406257 ) ) ;
#8891=CARTESIAN_POINT ( 'NONE',  ( -13.41834698511420676, -18.81097725173551893, 6.252442769197418926 ) ) ;
#8893=CARTESIAN_POINT ( 'NONE',  ( 12.80905858231679417, -23.27327832286945153, 2.298404588716537411 ) ) ;
#8897=CARTESIAN_POINT ( 'NONE',  ( 13.84863765609603625, 3.668701632846259830, 5.985835949623216301 ) ) ;
#8904=CARTESIAN_POINT ( 'NONE',  ( 13.87470602645761986, 4.985154336109792972, 4.583333333333296622 ) ) ;
#8906=CARTESIAN_POINT ( 'NONE',  ( 1.906542528716098417, -8.376716462152538512, 1.625674082428238298 ) ) ;
#8908=CARTESIAN_POINT ( 'NONE',  ( -13.09556065010287362, 4.263312830196960057, 5.034075356110313315 ) ) ;
#8910=CARTESIAN_POINT ( 'NONE',  ( -13.86436316834274329, 3.712840001305938831, 6.736817769197426031 ) ) ;
#8911=EDGE_CURVE ( 'NONE', #13563, #2750, #2382, .T. ) ;
#8913=CARTESIAN_POINT ( 'NONE',  ( 12.43405858231679417, -23.20159541128345992, 4.773278322869455970 ) ) ;
#8914=CARTESIAN_POINT ( 'NONE',  ( 4.003441417683176518, -22.05068747287765873, 5.250000000000000888 ) ) ;
#8915=CARTESIAN_POINT ( 'NONE',  ( -12.43405858231679417, -23.20159541128345992, 4.773278322869455970 ) ) ;
#8917=CARTESIAN_POINT ( 'NONE',  ( 13.01365964058540037, 0.1273118495903458325, 5.174178440007729307 ) ) ;
#8923=CARTESIAN_POINT ( 'NONE',  ( -12.79798428357658047, -11.51429367935891790, 5.673858176248284479 ) ) ;
#8924=CARTESIAN_POINT ( 'NONE',  ( -3.162271481458107658, -13.95306990448253437, 3.615178062515473911 ) ) ;
#8925=CARTESIAN_POINT ( 'NONE',  ( -13.84264281492353987, 3.365962153638767607, 5.979325532956542233 ) ) ;
#8927=CARTESIAN_POINT ( 'NONE',  ( 2.436080212393455735, -9.483920418190111334, 2.467411194204634839 ) ) ;
#8930=CARTESIAN_POINT ( 'NONE',  ( -0.5631383031621635116, -9.114917468222230923, 2.372643865078341019 ) ) ;
#8931=CARTESIAN_POINT ( 'NONE',  ( -8.965308582316795949, -19.47900456129164937, 4.484846433055089676 ) ) ;
#8932=CARTESIAN_POINT ( 'NONE',  ( -3.232228556578340850, -13.29361487011126464, 2.695816835751057461 ) ) ;
#8934=CARTESIAN_POINT ( 'NONE',  ( -13.09560264576187905, 4.265433610975056133, 4.333333333333380999 ) ) ;
#8936=CARTESIAN_POINT ( 'NONE',  ( 6.434058582316796837, -23.73192549717337130, 5.303608408759367343 ) ) ;
#8937=CARTESIAN_POINT ( 'NONE',  ( -8.784691417683177406, -23.02099543870834353, 3.863526089495429972 ) ) ;
#8939=CARTESIAN_POINT ( 'NONE',  ( 13.37499999999998224, -20.25000000000006395, 4.416666666666681174 ) ) ;
#8942=VERTEX_POINT ( 'NONE', #612 ) ;
#8945=CARTESIAN_POINT ( 'NONE',  ( -13.86693669322925260, 4.592803008081209448, 5.801483467520450077 ) ) ;
#8951=CARTESIAN_POINT ( 'NONE',  ( 1.548630333695928396, -9.114917468222230923, 2.372643865078341019 ) ) ;
#8953=CARTESIAN_POINT ( 'NONE',  ( 13.88045627189955233, 4.525541730927888473, 6.662882075361062029 ) ) ;
#8956=CARTESIAN_POINT ( 'NONE',  ( 13.12529397354238192, 5.014845663890295846, 4.166666666666765551 ) ) ;
#8957=CARTESIAN_POINT ( 'NONE',  ( 12.25344141768317741, -21.94931252712233061, 2.499999999999999112 ) ) ;
#8959=CARTESIAN_POINT ( 'NONE',  ( -5.034691417683177406, -20.97900456129164581, 3.136473910504570917 ) ) ;
#8960=CARTESIAN_POINT ( 'NONE',  ( -11.22219141768317741, -19.52099543870834353, 4.586221378810406257 ) ) ;
#8963=CARTESIAN_POINT ( 'NONE',  ( 12.66835678905406049, -17.31048215276408797, 4.799178440007564994 ) ) ;
#8964=CARTESIAN_POINT ( 'NONE',  ( -13.09293046926041626, 3.380488697651010011, 5.994170676248444352 ) ) ;
#8970=CARTESIAN_POINT ( 'NONE',  ( 2.436080212393455735, -9.483920418190111334, 2.467411194204634839 ) ) ;
#8978=CARTESIAN_POINT ( 'NONE',  ( -2.050137595624097031, -10.15260257655714504, 1.696527147986202522 ) ) ;
#8985=CARTESIAN_POINT ( 'NONE',  ( 5.309058582316795949, -23.80360840875935935, 1.768074502826626260 ) ) ;
#8986=CARTESIAN_POINT ( 'NONE',  ( -12.62745083560477966, -20.12623280195927933, 5.001038150054709419 ) ) ;
#8987=CARTESIAN_POINT ( 'NONE',  ( -4.565941417683176518, -23.73192549717336064, 1.696391591240623331 ) ) ;
#8988=EDGE_LOOP ( 'NONE', ( #12112, #1921, #4176, #18056, #5320 ) ) ;
#8992=CARTESIAN_POINT ( 'NONE',  ( -13.50467269799730374, -14.45152875114793467, 6.346192769197517514 ) ) ;
#8994=CARTESIAN_POINT ( 'NONE',  ( 12.52780858231679595, -23.72900456129165647, 4.275561207030568411 ) ) ;
#8999=CARTESIAN_POINT ( 'NONE',  ( 13.56222317325195093, -11.54522975075300728, 6.408692769197242178 ) ) ;
#9005=CARTESIAN_POINT ( 'NONE',  ( -13.18405858231679417, -20.79840458871652942, 2.226721677130544030 ) ) ;
#9009=AXIS2_PLACEMENT_3D ( 'NONE', #20257, #5500, #2360 ) ;
#9010=CARTESIAN_POINT ( 'NONE',  ( 2.682825141213236009, -9.727160171598653093, 1.779880022082258373 ) ) ;
#9011=CIRCLE ( 'NONE', #4336, 0.3749999999999998890 ) ;
#9013=CARTESIAN_POINT ( 'NONE',  ( -13.09560264576187905, 4.265433610975056133, 3.666666666666500873 ) ) ;
#9014=CARTESIAN_POINT ( 'NONE',  ( 11.21530858231679417, -23.77099543870833998, 2.825813738724734847 ) ) ;
#9015=CARTESIAN_POINT ( 'NONE',  ( -13.50467269799730374, -14.45152875114793467, 6.346192769197517514 ) ) ;
#9018=CARTESIAN_POINT ( 'NONE',  ( 5.871558582316795949, -20.99999999999999645, 3.449312527122348371 ) ) ;
#9019=CARTESIAN_POINT ( 'NONE',  ( 10.28469141768317741, -23.02099543870834353, 3.863526089495429972 ) ) ;
#9020=CARTESIAN_POINT ( 'NONE',  ( -11.96530858231679595, -20.22900456129164937, 4.174186261275266929 ) ) ;
#9022=CARTESIAN_POINT ( 'NONE',  ( 13.37908441539295801, -19.29373702265862889, 4.740102594697787275 ) ) ;
#9032=CARTESIAN_POINT ( 'NONE',  ( -2.731427961995660958, -10.89409100229510052, 2.829571171190552015 ) ) ;
#9033=CARTESIAN_POINT ( 'NONE',  ( -13.87215786865436762, 4.856472367046606564, 5.506273593909547515 ) ) ;
#9035=FACE_OUTER_BOUND ( 'NONE', #3773, .T. ) ;
#9039=CARTESIAN_POINT ( 'NONE',  ( -11.68405858231679595, -20.26807450282662160, 1.696391591240633101 ) ) ;
#9040=CARTESIAN_POINT ( 'NONE',  ( -3.002445346198714837, -11.66215945560911749, 2.276826493710632171 ) ) ;
#9042=CARTESIAN_POINT ( 'NONE',  ( -13.37515323800563039, -20.24226148071262799, 4.627790572011877934 ) ) ;
#9047=CARTESIAN_POINT ( 'NONE',  ( 6.340308582316796837, -22.98484643305508612, 6.020995438708344416 ) ) ;
#9048=CARTESIAN_POINT ( 'NONE',  ( -7.847191417683175629, -21.53509896474923835, 2.520995438708346192 ) ) ;
#9050=CARTESIAN_POINT ( 'NONE',  ( 13.39170256340046095, -19.40652054827866380, 5.481861153867630065 ) ) ;
#9056=CARTESIAN_POINT ( 'NONE',  ( -13.85788212999909419, 4.135547564954428879, 5.982801014393342776 ) ) ;
#9065=CARTESIAN_POINT ( 'NONE',  ( 3.385922596301560894, -9.481287983549590237, 1.909350115156127403 ) ) ;
#9070=CARTESIAN_POINT ( 'NONE',  ( 10.84719141768317741, -21.53509896474923835, 2.520995438708346192 ) ) ;
#9071=CARTESIAN_POINT ( 'NONE',  ( -12.64131715375063258, -19.42598373559290792, 5.491151580003103660 ) ) ;
#9072=CARTESIAN_POINT ( 'NONE',  ( -12.99655858231679595, -22.05068747287764452, 2.499999999999999112 ) ) ;
#9074=CARTESIAN_POINT ( 'NONE',  ( -11.87844141768317741, -24.50000000000000000, 3.449312527122335048 ) ) ;
#9076=CARTESIAN_POINT ( 'NONE',  ( 12.62503976493681535, -19.49799187068907713, 4.533161381885315144 ) ) ;
#9077=CARTESIAN_POINT ( 'NONE',  ( -12.66369984131459070, -18.29565801360988075, 5.528024842915327142 ) ) ;
#9083=CARTESIAN_POINT ( 'NONE',  ( 1.957016269584227031, -9.152392576945766578, 2.382268221639079364 ) ) ;
#9087=CARTESIAN_POINT ( 'NONE',  ( -2.327620134574780231, -13.27885108724501251, 3.249410218619480872 ) ) ;
#9091=CARTESIAN_POINT ( 'NONE',  ( 5.027808582316795949, -24.47900456129166358, 4.586221378810390270 ) ) ;
#9092=CARTESIAN_POINT ( 'NONE',  ( -13.09532840572934376, 3.501584489333809724, 5.996774842915142401 ) ) ;
#9093=CARTESIAN_POINT ( 'NONE',  ( -12.44094141768317741, -20.72672167713052715, 2.298404588716546293 ) ) ;
#9095=CARTESIAN_POINT ( 'NONE',  ( 11.21530858231679417, -23.77099543870833998, 2.825813738724734847 ) ) ;
#9097=CARTESIAN_POINT ( 'NONE',  ( -13.77324158252158171, -0.8888000826463379189, 6.637859435864801760 ) ) ;
#9099=CARTESIAN_POINT ( 'NONE',  ( 11.87155858231679417, -20.24999999999999289, 3.449312527122348371 ) ) ;
#9103=CARTESIAN_POINT ( 'NONE',  ( 13.37499999999998224, -21.00000000000006395, 4.416666666666682062 ) ) ;
#9111=CARTESIAN_POINT ( 'NONE',  ( -10.27780858231679417, -20.27099543870833642, 2.724438792969431589 ) ) ;
#9112=CARTESIAN_POINT ( 'NONE',  ( 13.87470623115321899, 4.985164673244912414, 4.958488177337359026 ) ) ;
#9114=CARTESIAN_POINT ( 'NONE',  ( 2.195822829018478473, -9.226849102155203042, 1.651390144731336163 ) ) ;
#9116=CARTESIAN_POINT ( 'NONE',  ( -13.09560269887985307, 4.265436293439658577, 4.973800642626965640 ) ) ;
#9117=FACE_OUTER_BOUND ( 'NONE', #11323, .T. ) ;
#9118=CARTESIAN_POINT ( 'NONE',  ( -13.37607268932110038, -20.94582918928111681, 4.945564004704174010 ) ) ;
#9121=CARTESIAN_POINT ( 'NONE',  ( 9.715308582316794173, -23.77099543870833998, 2.825813738724734847 ) ) ;
#9123=CARTESIAN_POINT ( 'NONE',  ( 3.944195004867016241, -21.61378581760806838, 5.207602947182413899 ) ) ;
#9124=CARTESIAN_POINT ( 'NONE',  ( -10.65969141768317918, -22.67418626127524917, 1.729004561291651587 ) ) ;
#9126=CARTESIAN_POINT ( 'NONE',  ( 13.09560264576187905, 4.265433610975056133, 3.666666666666500873 ) ) ;
#9129=ORIENTED_EDGE ( 'NONE', *, *, #17929, .T. ) ;
#9132=CARTESIAN_POINT ( 'NONE',  ( -13.10372118337080849, 3.925419760224517329, 6.005889426248455010 ) ) ;
#9134=CARTESIAN_POINT ( 'NONE',  ( -13.39170256340046095, -19.40652054827866380, 5.481861153867630065 ) ) ;
#9141=CARTESIAN_POINT ( 'NONE',  ( -12.52780858231679773, -24.47900456129166358, 4.586221378810390270 ) ) ;
#9142=CARTESIAN_POINT ( 'NONE',  ( -0.5631383031621635116, -9.114917468222230923, 1.622643865078341463 ) ) ;
#9144=CARTESIAN_POINT ( 'NONE',  ( -13.84074239313819277, 4.019990853478630832, 5.241358430878110930 ) ) ;
#9147=CARTESIAN_POINT ( 'NONE',  ( 12.44094141768317741, -20.19639159124061933, 1.768074502826635586 ) ) ;
#9148=CARTESIAN_POINT ( 'NONE',  ( -5.128441417683177406, -20.99999999999999645, 3.550687472877664952 ) ) ;
#9151=CARTESIAN_POINT ( 'NONE',  ( 13.86470821076586368, 4.480264643675554659, 5.874551681240599343 ) ) ;
#9152=CARTESIAN_POINT ( 'NONE',  ( 12.62499999999998224, -20.24999999999998934, 4.166666666666636765 ) ) ;
#9157=CARTESIAN_POINT ( 'NONE',  ( -13.87406079471522347, 4.952570133121557028, 5.260711232101737522 ) ) ;
#9158=CARTESIAN_POINT ( 'NONE',  ( 0.000000000000000000, -9.114917468222230923, 2.372643865078340575 ) ) ;
#9163=CARTESIAN_POINT ( 'NONE',  ( 2.739050625766161762, -9.875938058683834342, 1.818089155622620412 ) ) ;
#9169=CARTESIAN_POINT ( 'NONE',  ( 13.09030858231679417, -21.63647391050454871, 2.479004561291657804 ) ) ;
#9170=CARTESIAN_POINT ( 'NONE',  ( -13.12119116326504908, 4.807653744879115010, 5.626470997801169105 ) ) ;
#9171=CARTESIAN_POINT ( 'NONE',  ( -11.30905858231679595, -22.74294823697954016, 2.828734674606448785 ) ) ;
#9172=CARTESIAN_POINT ( 'NONE',  ( -12.25344141768317741, -21.94931252712233061, 0.9999999999999978906 ) ) ;
#9174=CARTESIAN_POINT ( 'NONE',  ( 13.09560264576187905, 4.265433610975056133, 4.666666666666618113 ) ) ;
#9179=CARTESIAN_POINT ( 'NONE',  ( 1.619022621591186928, -9.864917468222230923, 2.372643865078341019 ) ) ;
#9184=CARTESIAN_POINT ( 'NONE',  ( -0.9854920305337622199, -9.864917468222230923, 1.622643865078341907 ) ) ;
#9188=CARTESIAN_POINT ( 'NONE',  ( 8.315941417683177406, -20.26807450282663225, 5.303608408759377113 ) ) ;
#9190=CARTESIAN_POINT ( 'NONE',  ( -10.94094141768317741, -20.72672167713052715, 2.298404588716546293 ) ) ;
#9192=CARTESIAN_POINT ( 'NONE',  ( 6.152808582316793284, -21.22443879296942626, 5.229004561291659137 ) ) ;
#9194=CARTESIAN_POINT ( 'NONE',  ( -13.85956729540471066, 3.470648417939721231, 6.731609435864099211 ) ) ;
#9196=CARTESIAN_POINT ( 'NONE',  ( 12.05905858231679417, -20.72672167713054137, 4.701595411283463477 ) ) ;
#9197=DIRECTION ( 'NONE',  ( 0.000000000000000000, 0.000000000000000000, 1.000000000000000000 ) ) ;
#9198=EDGE_LOOP ( 'NONE', ( #16935, #14004, #6688, #5641, #6486 ) ) ;
#9200=CARTESIAN_POINT ( 'NONE',  ( 13.67732412376249052, -5.732631749971324631, 6.533692769198849781 ) ) ;
#9204=SURFACE_SIDE_STYLE ('',( #3136 ) ) ;
#9211=CARTESIAN_POINT ( 'NONE',  ( 2.768424032093183662, -10.00067216410020166, 1.850123365707658785 ) ) ;
#9214=CARTESIAN_POINT ( 'NONE',  ( -13.09358652029869141, 4.163619275088517035, 5.207983256689002083 ) ) ;
#9215=CARTESIAN_POINT ( 'NONE',  ( 9.340308582316794173, -22.67418626127525982, 5.270995438708342640 ) ) ;
#9216=CARTESIAN_POINT ( 'NONE',  ( -13.71569110726703045, -3.795099083046435506, 6.575359435862661250 ) ) ;
#9218=CARTESIAN_POINT ( 'NONE',  ( 5.215308582316795949, -23.02099543870833998, 3.136473910504556262 ) ) ;
#9220=CARTESIAN_POINT ( 'NONE',  ( 11.22219141768317741, -21.02099543870834353, 3.964901035250761208 ) ) ;
#9221=CARTESIAN_POINT ( 'NONE',  ( -4.840308582316793284, -22.67418626127525982, 5.270995438708342640 ) ) ;
#9223=CARTESIAN_POINT ( 'NONE',  ( 13.37499999999998224, -19.49999999999998934, 4.166666666666637653 ) ) ;
#9229=CARTESIAN_POINT ( 'NONE',  ( -12.64751377014909828, -19.11305460747000495, 5.510446717915143289 ) ) ;
#9230=CARTESIAN_POINT ( 'NONE',  ( -2.534747216115884161, -9.671180236796224960, 2.515503256513427210 ) ) ;
#9231=CARTESIAN_POINT ( 'NONE',  ( -13.39902456816392906, -19.03675930772010361, 5.497554699623231400 ) ) ;
#9237=CARTESIAN_POINT ( 'NONE',  ( 4.647268150593999003, -21.47219718316376458, 5.373337411135923780 ) ) ;
#9238=CARTESIAN_POINT ( 'NONE',  ( -12.43405858231679595, -23.73192549717337130, 5.303608408759367343 ) ) ;
#9239=CARTESIAN_POINT ( 'NONE',  ( -0.2815691515810352374, -8.364917468222230923, 1.622643865078524428 ) ) ;
#9240=EDGE_CURVE ( 'NONE', #7887, #18614, #4970, .T. ) ;
#9243=CARTESIAN_POINT ( 'NONE',  ( -13.84476264919594612, 4.223013784394161974, 5.079233071712400793 ) ) ;
#9245=CARTESIAN_POINT ( 'NONE',  ( 10.00344141768317741, -22.05068747287766229, 6.000000000000001776 ) ) ;
#9246=CARTESIAN_POINT ( 'NONE',  ( -5.315941417683176518, -21.32873467460645145, 4.242948236979555254 ) ) ;
#9248=CARTESIAN_POINT ( 'NONE',  ( 13.87470602645761986, 4.985154336109792972, 4.333333333333382775 ) ) ;
#9254=CARTESIAN_POINT ( 'NONE',  ( -13.39722611581222189, -19.12758115148224647, 5.495601574623241170 ) ) ;
#9259=CARTESIAN_POINT ( 'NONE',  ( 2.594671182134835163, -9.923034775318452461, 2.580184533305832861 ) ) ;
#9262=CARTESIAN_POINT ( 'NONE',  ( 3.475298211275419380, -9.785109117490691233, 1.987377451789144933 ) ) ;
#9264=CARTESIAN_POINT ( 'NONE',  ( 13.12529397354238192, 5.014845663890295846, 4.791666666666685614 ) ) ;
#9268=CARTESIAN_POINT ( 'NONE',  ( 8.503441417683177406, -22.05068747287766229, 4.499999999999999112 ) ) ;
#9269=CARTESIAN_POINT ( 'NONE',  ( -13.12529418130016445, 5.014856155665242454, 4.958178834604180629 ) ) ;
#9270=CARTESIAN_POINT ( 'NONE',  ( -8.402808582316797725, -22.46490103525074034, 2.520995438708341307 ) ) ;
#9271=CARTESIAN_POINT ( 'NONE',  ( -6.065941417683177406, -23.73192549717336064, 1.696391591240623331 ) ) ;
#9273=CARTESIAN_POINT ( 'NONE',  ( 13.37680511754115287, -19.40884156416817774, 4.692171866446762429 ) ) ;
#9279=CARTESIAN_POINT ( 'NONE',  ( 1.743623630681728542, -9.116095536440919744, 2.372946416531167557 ) ) ;
#9285=CARTESIAN_POINT ( 'NONE',  ( -2.081625295426255295, -10.37614485793134556, 1.753937271548854815 ) ) ;
#9290=CARTESIAN_POINT ( 'NONE',  ( 3.974842109207560537, -21.73478823434188456, 6.006404853634143670 ) ) ;
#9293=CARTESIAN_POINT ( 'NONE',  ( -8.972191417683177406, -23.72900456129165292, 2.724438792969417822 ) ) ;
#9295=CARTESIAN_POINT ( 'NONE',  ( 13.27780858231679417, -19.52099543870833642, 2.413778621189609286 ) ) ;
#9297=CARTESIAN_POINT ( 'NONE',  ( -13.90434039801927568, 5.731690099970989216, 5.115558489342345361 ) ) ;
#9300=CARTESIAN_POINT ( 'NONE',  ( 6.902808582316793284, -22.77556120703056308, 1.770995438708339975 ) ) ;
#9303=CARTESIAN_POINT ( 'NONE',  ( 13.37923893525309715, -20.78593376972237650, 5.366589449429977954 ) ) ;
#9310=ORIENTED_EDGE ( 'NONE', *, *, #8649, .F. ) ;
#9311=CARTESIAN_POINT ( 'NONE',  ( -13.27780858231679595, -20.27099543870833642, 2.724438792969431589 ) ) ;
#9312=CARTESIAN_POINT ( 'NONE',  ( 12.62500000000001954, -20.25000000000274269, 4.083333333315724012 ) ) ;
#9313=CARTESIAN_POINT ( 'NONE',  ( 3.187906586576829682, -9.105473976199601083, 1.812833570429532859 ) ) ;
#9315=CARTESIAN_POINT ( 'NONE',  ( -13.37818000216760694, -19.33940989053615311, 4.728953261990445966 ) ) ;
#9317=CARTESIAN_POINT ( 'NONE',  ( 8.590308582316794173, -21.32581373872472597, 1.729004561291657582 ) ) ;
#9318=CARTESIAN_POINT ( 'NONE',  ( -13.87824226375436965, 4.413734319597230282, 6.694665752684481497 ) ) ;
#9321=CARTESIAN_POINT ( 'NONE',  ( 9.340308582316794173, -22.67418626127525982, 5.270995438708342640 ) ) ;
#9323=CARTESIAN_POINT ( 'NONE',  ( 12.99655858231679595, -22.05068747287764452, 2.499999999999999112 ) ) ;
#9325=CARTESIAN_POINT ( 'NONE',  ( 13.41806913471718588, -17.32500869677464550, 4.784333296715663764 ) ) ;
#9332=CARTESIAN_POINT ( 'NONE',  ( -12.65051119073526564, -18.96168486786632457, 5.513701926248478102 ) ) ;
#9334=CARTESIAN_POINT ( 'NONE',  ( -2.616191246582922680, -8.630616848980537270, 2.440880773935528048 ) ) ;
#9335=CARTESIAN_POINT ( 'NONE',  ( -13.39296152110871851, -19.34294318400601753, 5.489418334493660012 ) ) ;
#9338=CARTESIAN_POINT ( 'NONE',  ( 11.68405858231679417, -20.79840458871652942, 2.226721677130544030 ) ) ;
#9340=CARTESIAN_POINT ( 'NONE',  ( 13.12519991495504712, 4.260095705229160146, 6.739971950528219402 ) ) ;
#9341=CARTESIAN_POINT ( 'NONE',  ( -5.402808582316795949, -23.08622137881038938, 1.020995438708339309 ) ) ;
#9342=CARTESIAN_POINT ( 'NONE',  ( -1.872293763630120678, -10.04602735435188698, 2.419156501869924369 ) ) ;
#9344=CARTESIAN_POINT ( 'NONE',  ( -13.37499999999998224, -20.24999999999998934, 4.166666666666636765 ) ) ;
#9346=CARTESIAN_POINT ( 'NONE',  ( 10.19094141768317741, -23.80360840875937001, 5.231925497173365081 ) ) ;
#9347=CARTESIAN_POINT ( 'NONE',  ( -7.003441417683177406, -22.05068747287766229, 4.499999999999999112 ) ) ;
#9350=CARTESIAN_POINT ( 'NONE',  ( 13.41834698511420676, -18.81097725173551893, 6.252442769197418926 ) ) ;
#9357=CARTESIAN_POINT ( 'NONE',  ( -13.39662663169496781, -19.15785509940297615, 5.494950532956567102 ) ) ;
#9364=CARTESIAN_POINT ( 'NONE',  ( 2.534747216115884161, -9.671180236796224960, 2.515503256513427210 ) ) ;
#9366=CARTESIAN_POINT ( 'NONE',  ( 1.720709671993384093, -9.114925383610804843, 1.622645897908254753 ) ) ;
#9373=CARTESIAN_POINT ( 'NONE',  ( 6.440941417683175629, -21.25705176302044208, 2.828734674606458555 ) ) ;
#9374=CARTESIAN_POINT ( 'NONE',  ( -13.10252221513633941, 3.864871864382954048, 6.004587342915129966 ) ) ;
#9375=CARTESIAN_POINT ( 'NONE',  ( -9.902808582316795949, -22.46490103525074034, 2.520995438708341307 ) ) ;
#9376=CARTESIAN_POINT ( 'NONE',  ( -6.815941417683177406, -20.26807450282663225, 5.303608408759377113 ) ) ;
#9378=CARTESIAN_POINT ( 'NONE',  ( 13.09556065010287362, 4.263312830196960057, 5.034075356110313315 ) ) ;
#9385=CARTESIAN_POINT ( 'NONE',  ( 1.865667289525601680, -9.999006358835732300, 2.407080570882605297 ) ) ;
#9391=CARTESIAN_POINT ( 'NONE',  ( 8.034691417683175629, -20.22900456129164581, 2.825813738724748170 ) ) ;
#9393=CARTESIAN_POINT ( 'NONE',  ( -1.866357130655357688, -10.00562759449716133, 2.408781036472938730 ) ) ;
#9398=CARTESIAN_POINT ( 'NONE',  ( 12.34719141768317563, -21.22443879296941915, 1.770995438708345748 ) ) ;
#9400=CARTESIAN_POINT ( 'NONE',  ( -6.909691417683177406, -21.32581373872474373, 5.270995438708348857 ) ) ;
#9403=CARTESIAN_POINT ( 'NONE',  ( 6.434058582316794173, -23.20159541128345992, 4.773278322869455970 ) ) ;
#9405=CARTESIAN_POINT ( 'NONE',  ( -12.62527129584495000, -20.98629955982801576, 4.726243163759704657 ) ) ;
#9412=CARTESIAN_POINT ( 'NONE',  ( 13.87500000000000000, 5.000000000000049738, 4.000000000000001776 ) ) ;
#9417=CARTESIAN_POINT ( 'NONE',  ( -11.96530858231679595, -20.22900456129164937, 4.174186261275266929 ) ) ;
#9419=CARTESIAN_POINT ( 'NONE',  ( 12.64131715375063258, -19.42598373559290792, 5.491151580003103660 ) ) ;
#9422=CARTESIAN_POINT ( 'NONE',  ( 0.5631383031621635116, -9.864917468222230923, 1.622643865078341907 ) ) ;
#9425=CARTESIAN_POINT ( 'NONE',  ( -13.68663801924254741, -3.762280028282741551, 5.075999963380942503 ) ) ;
#9426=CARTESIAN_POINT ( 'NONE',  ( 4.934058582316793284, -23.20159541128345992, 4.773278322869455970 ) ) ;
#9427=CARTESIAN_POINT ( 'NONE',  ( -12.66024186180961308, -19.22028597861421417, 6.258173329156003106 ) ) ;
#9429=CARTESIAN_POINT ( 'NONE',  ( 8.121558582316792396, -23.74999999999999645, 3.550687472877651629 ) ) ;
#9430=CARTESIAN_POINT ( 'NONE',  ( 6.440941417683175629, -21.25705176302044208, 2.828734674606458555 ) ) ;
#9431=CARTESIAN_POINT ( 'NONE',  ( -6.715308582316794173, -23.77099543870833998, 2.825813738724734847 ) ) ;
#9433=CARTESIAN_POINT ( 'NONE',  ( 13.37499999998404299, -19.49999999996810729, 2.793053905886972998 ) ) ;
#9434=CARTESIAN_POINT ( 'NONE',  ( -2.506848361495492394, -9.459347215042898327, 1.711100304737409150 ) ) ;
#9440=CARTESIAN_POINT ( 'NONE',  ( -0.2815691515810352374, -8.364917468222230923, 2.372643865078523540 ) ) ;
#9446=CARTESIAN_POINT ( 'NONE',  ( 10.09030858231679417, -21.32581373872472952, 1.729004561291657138 ) ) ;
#9448=CARTESIAN_POINT ( 'NONE',  ( 12.62499979224180180, -20.25001049178813162, 4.458178821399696012 ) ) ;
#9449=CARTESIAN_POINT ( 'NONE',  ( -12.15969141768317918, -22.98484643305507191, 0.9790045612916508100 ) ) ;
#9450=CARTESIAN_POINT ( 'NONE',  ( -0.5631383031621635116, -9.864917468222230923, 1.622643865078341907 ) ) ;
#9452=CARTESIAN_POINT ( 'NONE',  ( -13.84501469867711698, 4.235742283194553259, 4.333333333333380999 ) ) ;
#9454=CARTESIAN_POINT ( 'NONE',  ( 12.62844141768317741, -20.24999999999999289, 3.550687472877664952 ) ) ;
#9455=CARTESIAN_POINT ( 'NONE',  ( -11.12155858231679595, -22.99999999999999645, 3.550687472877652073 ) ) ;
#9457=CARTESIAN_POINT ( 'NONE',  ( 13.40957725085194241, -19.25384883197511243, 6.242932005802575901 ) ) ;
#9458=CARTESIAN_POINT ( 'NONE',  ( 12.62499999999998224, -20.25000000000006395, 4.416666666666681174 ) ) ;
#9470=CARTESIAN_POINT ( 'NONE',  ( 3.059891148793807414, -12.07002330923453570, 2.381574079220715401 ) ) ;
#9477=CARTESIAN_POINT ( 'NONE',  ( -12.62499999999990052, -20.34958158682421114, 3.551156945994469627 ) ) ;
#9478=CARTESIAN_POINT ( 'NONE',  ( 4.190941417683176518, -22.74294823697955081, 4.171265325393542334 ) ) ;
#9479=CARTESIAN_POINT ( 'NONE',  ( -13.12424783836753228, 4.962015837561366993, 5.328858059679200565 ) ) ;
#9480=CARTESIAN_POINT ( 'NONE',  ( -6.715308582316796837, -23.02099543870833998, 3.136473910504556262 ) ) ;
#9481=CARTESIAN_POINT ( 'NONE',  ( -11.78469141768317563, -23.77099543870834353, 4.174186261275252718 ) ) ;
#9484=CARTESIAN_POINT ( 'NONE',  ( 13.09560264576187905, 4.265433610975056133, 2.999999999999999556 ) ) ;
#9492=CARTESIAN_POINT ( 'NONE',  ( 8.597191417683177406, -22.77556120703057729, 5.229004561291656472 ) ) ;
#9494=CARTESIAN_POINT ( 'NONE',  ( -1.717920576997000737, -9.114924032904250240, 2.372645551019823884 ) ) ;
#9499=CARTESIAN_POINT ( 'NONE',  ( 7.190941417683177406, -23.80360840875937001, 5.231925497173365081 ) ) ;
#9500=CARTESIAN_POINT ( 'NONE',  ( -8.597191417683177406, -22.77556120703057729, 5.229004561291655584 ) ) ;
#9502=CARTESIAN_POINT ( 'NONE',  ( 6.996558582316793284, -22.05068747287764452, 1.749999999999998446 ) ) ;
#9503=CARTESIAN_POINT ( 'NONE',  ( 12.62499999999998401, -20.24999999999998934, 2.439580858552613751 ) ) ;
#9504=CARTESIAN_POINT ( 'NONE',  ( -12.85087781109329974, -9.593170539812428288, 6.465204579154565145 ) ) ;
#9506=CARTESIAN_POINT ( 'NONE',  ( 6.152808582316793284, -21.22443879296942626, 5.229004561291659137 ) ) ;
#9513=CARTESIAN_POINT ( 'NONE',  ( -6.996558582316793284, -22.05068747287764452, 1.749999999999998446 ) ) ;
#9516=CARTESIAN_POINT ( 'NONE',  ( 2.557403344953185442, -14.91030650174552896, 3.668400560659690779 ) ) ;
#9520=CARTESIAN_POINT ( 'NONE',  ( -13.84402619238587206, 4.185822715484293077, 5.150938132831436533 ) ) ;
#9521=CARTESIAN_POINT ( 'NONE',  ( 6.715308582316794173, -23.77099543870833998, 2.825813738724734847 ) ) ;
#9522=CARTESIAN_POINT ( 'NONE',  ( -12.62608183053121458, -20.94536755816881168, 4.949360998036265613 ) ) ;
#9524=CARTESIAN_POINT ( 'NONE',  ( -5.871558582316795949, -19.49999999999998934, 3.449312527122348371 ) ) ;
#9527=CARTESIAN_POINT ( 'NONE',  ( 5.222191417683177406, -21.02099543870834353, 3.964901035250761208 ) ) ;
#9528=CARTESIAN_POINT ( 'NONE',  ( -11.22219141768317741, -20.27099543870833998, 4.275561207030583510 ) ) ;
#9530=CARTESIAN_POINT ( 'NONE',  ( 13.83051420738022763, 3.503467472703414742, 5.232249963382380464 ) ) ;
#9539=CARTESIAN_POINT ( 'NONE',  ( -3.549867680106858714, -10.29705900472337632, 2.118856410057032402 ) ) ;
#9544=CARTESIAN_POINT ( 'NONE',  ( -12.62562019941893432, -20.21867992933967173, 4.757612834768309540 ) ) ;
#9545=CARTESIAN_POINT ( 'NONE',  ( 10.55905858231679595, -20.72672167713054137, 4.701595411283463477 ) ) ;
#9547=CARTESIAN_POINT ( 'NONE',  ( 13.15469878640066526, 5.749788713235649773, 5.232478742873432509 ) ) ;
#9548=CARTESIAN_POINT ( 'NONE',  ( -2.050137595624097031, -10.15260257655714504, 1.696527147986202522 ) ) ;
#9550=CARTESIAN_POINT ( 'NONE',  ( -13.37499999999998401, -20.99999999999999645, 3.146526952850934755 ) ) ;
#9552=CARTESIAN_POINT ( 'NONE',  ( 6.909691417683176518, -21.01515356694492098, 6.020995438708349745 ) ) ;
#9553=CARTESIAN_POINT ( 'NONE',  ( -11.87155858231679595, -20.99999999999999645, 3.449312527122348371 ) ) ;
#9555=CARTESIAN_POINT ( 'NONE',  ( 13.37505392270939986, -20.99727690317663686, 4.612442573673130930 ) ) ;
#9564=CARTESIAN_POINT ( 'NONE',  ( 2.645259258103298983, -10.28229522185712241, 2.672449792925449596 ) ) ;
#9566=CARTESIAN_POINT ( 'NONE',  ( 1.797685059409938280, -9.880079706704160358, 1.626537830816663588 ) ) ;
#9572=CARTESIAN_POINT ( 'NONE',  ( -2.559937518207947793, -9.746075135043517079, 2.534737762559237773 ) ) ;
#9573=CARTESIAN_POINT ( 'NONE',  ( 12.34030858231679773, -22.36352608949544418, 4.520995438708343528 ) ) ;
#9574=CARTESIAN_POINT ( 'NONE',  ( -12.95145221759166354, -3.764163011652346569, 5.840524842913703552 ) ) ;
#9575=CARTESIAN_POINT ( 'NONE',  ( -11.02780858231679595, -23.72900456129165647, 4.275561207030568411 ) ) ;
#9576=CARTESIAN_POINT ( 'NONE',  ( -5.972191417683178294, -24.47900456129165292, 2.413778621189595963 ) ) ;
#9577=ORIENTED_EDGE ( 'NONE', *, *, #7561, .F. ) ;
#9578=CARTESIAN_POINT ( 'NONE',  ( 13.04243487821393721, 1.580461349787872782, 5.205428440007538349 ) ) ;
#9579=SURFACE_STYLE_FILL_AREA ( #17528 ) ;
#9587=CARTESIAN_POINT ( 'NONE',  ( 12.34719141768317741, -21.22443879296941915, 1.770995438708345748 ) ) ;
#9589=CARTESIAN_POINT ( 'NONE',  ( -3.277163086644854229, -14.76879761173520578, 3.824673233536266537 ) ) ;
#9591=CARTESIAN_POINT ( 'NONE',  ( -12.90280858231679595, -22.77556120703056308, 1.770995438708340197 ) ) ;
#9593=CARTESIAN_POINT ( 'NONE',  ( 7.940941417683175629, -20.19639159124061933, 1.768074502826635586 ) ) ;
#9594=DIRECTION ( 'NONE',  ( -0.000000000000000000, -0.000000000000000000, -1.000000000000000000 ) ) ;
#9595=CARTESIAN_POINT ( 'NONE',  ( -6.628441417683176518, -20.24999999999999289, 3.550687472877664952 ) ) ;
#9597=CARTESIAN_POINT ( 'NONE',  ( 8.027808582316792396, -23.72900456129165647, 4.275561207030568411 ) ) ;
#9599=CARTESIAN_POINT ( 'NONE',  ( -12.63806878948643231, -20.34002613093225520, 5.891296472647073124 ) ) ;
#9601=CARTESIAN_POINT ( 'NONE',  ( 5.871558582316794173, -20.24999999999999289, 3.449312527122348371 ) ) ;
#9609=CARTESIAN_POINT ( 'NONE',  ( -4.840308582316793284, -22.67418626127525982, 5.270995438708342640 ) ) ;
#9610=CARTESIAN_POINT ( 'NONE',  ( 12.64751377014909828, -19.11305460747000495, 5.510446717915143289 ) ) ;
#9613=CARTESIAN_POINT ( 'NONE',  ( 1.619022621591186928, -9.864917468222230923, 1.622643865078341907 ) ) ;
#9614=EDGE_CURVE ( 'NONE', #10698, #1939, #6330, .T. ) ;
#9617=CARTESIAN_POINT ( 'NONE',  ( -13.83973345681288158, 3.969039569021246550, 5.242263935944164288 ) ) ;
#9618=CARTESIAN_POINT ( 'NONE',  ( 8.027808582316792396, -23.72900456129165647, 4.275561207030568411 ) ) ;
#9619=CARTESIAN_POINT ( 'NONE',  ( -12.62500028073152869, -20.99998582305707728, 4.544498183892649479 ) ) ;
#9621=CARTESIAN_POINT ( 'NONE',  ( -7.934058582316796837, -23.73192549717337130, 5.303608408759367343 ) ) ;
#9622=CARTESIAN_POINT ( 'NONE',  ( 8.309058582316792396, -23.27327832286945153, 2.298404588716537411 ) ) ;
#9623=CARTESIAN_POINT ( 'NONE',  ( 6.534691417683177406, -20.97900456129164581, 3.136473910504570917 ) ) ;
#9624=CARTESIAN_POINT ( 'NONE',  ( -7.659691417683176518, -22.67418626127524917, 1.729004561291651587 ) ) ;
#9628=CARTESIAN_POINT ( 'NONE',  ( 13.37500000000002132, -20.24999999999450040, 3.833333333368183382 ) ) ;
#9637=CARTESIAN_POINT ( 'NONE',  ( -13.12529397354238192, 5.014845663890295846, 4.791666666666685614 ) ) ;
#9639=CARTESIAN_POINT ( 'NONE',  ( -0.5631383031621635116, -9.114917468222230923, 2.372643865078341019 ) ) ;
#9642=CARTESIAN_POINT ( 'NONE',  ( 2.693754455098655409, -10.04853567022903782, 2.237415670251142519 ) ) ;
#9643=CARTESIAN_POINT ( 'NONE',  ( -12.64511805349267526, -19.23403829861753422, 5.507852591554869726 ) ) ;
#9646=CARTESIAN_POINT ( 'NONE',  ( 13.15047398821051239, 5.536436404627260721, 5.896317606305554015 ) ) ;
#9649=CARTESIAN_POINT ( 'NONE',  ( -2.167793999318431197, -10.98794063836983703, 1.911058649813994315 ) ) ;
#9651=CARTESIAN_POINT ( 'NONE',  ( -13.87470602645761986, 4.985154336109792972, 4.166666666666765551 ) ) ;
#9653=CARTESIAN_POINT ( 'NONE',  ( 8.128441417683177406, -19.49999999999998934, 3.550687472877664952 ) ) ;
#9654=CARTESIAN_POINT ( 'NONE',  ( -8.777808582316797725, -21.02099543870833998, 3.035098964749253003 ) ) ;
#9657=CARTESIAN_POINT ( 'NONE',  ( 13.85716935893578317, 3.349552626256921517, 6.729005269197402939 ) ) ;
#9658=CARTESIAN_POINT ( 'NONE',  ( 12.69247507894198712, -16.84250851341299082, 5.559274842915185033 ) ) ;
#9670=CARTESIAN_POINT ( 'NONE',  ( 2.044552395631970665, -10.13052631352519306, 1.690857522621936226 ) ) ;
#9679=CARTESIAN_POINT ( 'NONE',  ( 8.965308582316795949, -20.97900456129165647, 3.863526089495444626 ) ) ;
#9680=CARTESIAN_POINT ( 'NONE',  ( -12.63298722613685676, -19.09664508008815531, 4.760766981674283471 ) ) ;
#9681=CARTESIAN_POINT ( 'NONE',  ( -11.40280858231679417, -22.77556120703056308, 1.770995438708339975 ) ) ;
#9683=CARTESIAN_POINT ( 'NONE',  ( -10.65969141768318096, -22.67418626127524917, 1.729004561291651809 ) ) ;
#9685=CARTESIAN_POINT ( 'NONE',  ( 13.84074239313819277, 4.019990853478630832, 5.241358430878110930 ) ) ;
#9695=CARTESIAN_POINT ( 'NONE',  ( 12.15969141768317563, -22.67418626127524917, 1.729004561291651587 ) ) ;
#9698=CARTESIAN_POINT ( 'NONE',  ( -0.9854920305337621089, -9.114917468222230923, 2.372643865078341019 ) ) ;
#9700=CARTESIAN_POINT ( 'NONE',  ( -10.37155858231679417, -20.24999999999999289, 3.449312527122348371 ) ) ;
#9703=CARTESIAN_POINT ( 'NONE',  ( 6.628441417683176518, -20.24999999999999289, 3.550687472877664952 ) ) ;
#9705=CARTESIAN_POINT ( 'NONE',  ( -6.065941417683177406, -23.20159541128344927, 2.226721677130534705 ) ) ;
#9707=CARTESIAN_POINT ( 'NONE',  ( 7.184058582316795949, -20.26807450282662160, 1.696391591240633101 ) ) ;
#9709=CARTESIAN_POINT ( 'NONE',  ( -12.64802275499843454, -19.83735087257960927, 6.157588447769994922 ) ) ;
#9716=ORIENTED_EDGE ( 'NONE', *, *, #1059, .F. ) ;
#9721=CARTESIAN_POINT ( 'NONE',  ( -11.87155858231679595, -19.49999999999998934, 3.449312527122348371 ) ) ;
#9722=CARTESIAN_POINT ( 'NONE',  ( 12.62745083560477966, -20.12623280195927933, 5.001038150054709419 ) ) ;
#9724=CARTESIAN_POINT ( 'NONE',  ( 1.897597015127918230, -9.924601616748528699, 1.637971946730535588 ) ) ;
#9726=CARTESIAN_POINT ( 'NONE',  ( 13.02818618459764188, 0.1109023222084986743, 5.923858176248589125 ) ) ;
#9729=CARTESIAN_POINT ( 'NONE',  ( -13.76337198624852398, 0.1127853055781036368, 5.159333296715827188 ) ) ;
#9730=CARTESIAN_POINT ( 'NONE',  ( 10.93405858231679595, -23.73192549717337130, 5.303608408759367343 ) ) ;
#9731=CARTESIAN_POINT ( 'NONE',  ( -13.08107971211413378, 2.032025461757085427, 6.715204579155630960 ) ) ;
#9734=CARTESIAN_POINT ( 'NONE',  ( 5.777808582316794173, -20.27099543870833642, 2.724438792969431589 ) ) ;
#9735=CARTESIAN_POINT ( 'NONE',  ( 8.690941417683177406, -22.74294823697955081, 4.171265325393542334 ) ) ;
#9736=CARTESIAN_POINT ( 'NONE',  ( -5.315941417683176518, -20.79840458871654363, 4.773278322869464851 ) ) ;
#9740=CARTESIAN_POINT ( 'NONE',  ( 13.84501469867711698, 4.235742283194553259, 4.916666666666649199 ) ) ;
#9750=CARTESIAN_POINT ( 'NONE',  ( -2.532303758294933704, -8.551221675625164664, 1.670490507339845054 ) ) ;
#9753=CARTESIAN_POINT ( 'NONE',  ( -12.62499979224180180, -20.25001049178813162, 4.458178821399696012 ) ) ;
#9754=CARTESIAN_POINT ( 'NONE',  ( 11.21530858231679417, -23.77099543870833998, 2.825813738724734847 ) ) ;
#9756=CARTESIAN_POINT ( 'NONE',  ( 13.15498530132288479, 5.764257716805535559, 4.583333333333295734 ) ) ;
#9759=CARTESIAN_POINT ( 'NONE',  ( -2.442511739767545098, -14.09457879449248807, 3.458905389639174821 ) ) ;
#9761=CARTESIAN_POINT ( 'NONE',  ( -13.37500000000002132, -20.99999999999450395, 3.833333333368183382 ) ) ;
#9763=CARTESIAN_POINT ( 'NONE',  ( 4.753441417683176518, -21.94931252712233061, 0.9999999999999978906 ) ) ;
#9764=CARTESIAN_POINT ( 'NONE',  ( -6.715308582316796837, -23.02099543870833998, 3.136473910504556262 ) ) ;
#9766=CARTESIAN_POINT ( 'NONE',  ( 13.67732412376249052, -5.732631749971324631, 6.533692769198849781 ) ) ;
#9767=CARTESIAN_POINT ( 'NONE',  ( 13.12529397354238192, 5.014845663890295846, 4.333333333333382775 ) ) ;
#9771=ORIENTED_EDGE ( 'NONE', *, *, #5397, .T. ) ;
#9777=CARTESIAN_POINT ( 'NONE',  ( 1.744064896197293324, -9.868721669903177229, 1.623620860066563365 ) ) ;
#9783=CARTESIAN_POINT ( 'NONE',  ( -11.02780858231679595, -23.72900456129165647, 4.275561207030568411 ) ) ;
#9784=EDGE_CURVE ( 'NONE', #12628, #4517, #18320, .T. ) ;
#9785=CARTESIAN_POINT ( 'NONE',  ( -2.436080212393455735, -9.483920418190111334, 2.467411194204634839 ) ) ;
#9787=CARTESIAN_POINT ( 'NONE',  ( -13.09543520949579865, 4.256978079540234106, 5.067654010725516578 ) ) ;
#9788=CARTESIAN_POINT ( 'NONE',  ( -11.12155858231679417, -23.74999999999999645, 3.550687472877651629 ) ) ;
#9790=CARTESIAN_POINT ( 'NONE',  ( -4.753441417683176518, -21.94931252712233061, 1.749999999999998446 ) ) ;
#9792=CARTESIAN_POINT ( 'NONE',  ( 13.41806913471718588, -17.32500869677464550, 4.784333296715663764 ) ) ;
#9794=EDGE_LOOP ( 'NONE', ( #19428, #1862, #12635, #9129, #6769 ) ) ;
#9795=DIRECTION ( 'NONE',  ( 0.000000000000000000, 0.000000000000000000, 1.000000000000000000 ) ) ;
#9799=B_SPLINE_CURVE_WITH_KNOTS ( 'NONE', 3,
 ( #15702, #1278, #4519, #4612, #17375, #13921, #12464, #4827, #7658, #10804, #9434, #11005, #1386, #20634, #20322, #17173, #15595, #6190, #2850, #3060, #15807, #10905, #14132, #12558, #20537, #1484, #5985, #14028, #18959, #19063 ),
 .UNSPECIFIED., .F., .F.,
 ( 4, 2, 2, 2, 2, 2, 2, 2, 2, 2, 2, 2, 2, 2, 4 ),
 ( 0.6080100341812841869, 0.6200887121040892236, 0.6309950902025724950, 0.6419014683010558775, 0.6637142244980225314, 0.7073397368919559502, 0.7509652492858893691, 0.7727780054828560230, 0.7836843835813394055, 0.7945907616798226769, 0.8074288390748337596, 0.8202669164698448423, 0.8459430712598670077, 0.8972953808399113385, 1.000000000000000000 ),
 .UNSPECIFIED. ) ;
#9801=CARTESIAN_POINT ( 'NONE',  ( 10.09719141768317563, -22.77556120703057729, 5.229004561291656472 ) ) ;
#9803=CARTESIAN_POINT ( 'NONE',  ( -1.337453470010121714, -9.864917468222230923, 2.372643865078341019 ) ) ;
#9805=CARTESIAN_POINT ( 'NONE',  ( -9.809058582316794173, -23.27327832286945153, 2.298404588716537411 ) ) ;
#9807=CARTESIAN_POINT ( 'NONE',  ( 8.315941417683177406, -20.79840458871654363, 4.773278322869464851 ) ) ;
#9809=CARTESIAN_POINT ( 'NONE',  ( -12.25344141768317741, -21.94931252712233061, 2.499999999999999112 ) ) ;
#9812=CARTESIAN_POINT ( 'NONE',  ( 10.93405858231679595, -23.73192549717337130, 5.303608408759367343 ) ) ;
#9813=CARTESIAN_POINT ( 'NONE',  ( 12.72125031657057015, -15.38935901321805133, 5.590524842915047365 ) ) ;
#9814=CARTESIAN_POINT ( 'NONE',  ( -13.11644927503132330, 3.818188389080370282, 6.753616037489316604 ) ) ;
#9822=CARTESIAN_POINT ( 'NONE',  ( 12.69874195915161330, -20.02071431810549740, 3.541097010573131421 ) ) ;
#9824=CARTESIAN_POINT ( 'NONE',  ( -4.934058582316793284, -23.20159541128345992, 4.773278322869455970 ) ) ;
#9825=CARTESIAN_POINT ( 'NONE',  ( 13.09532840572934376, 3.501584489333809724, 5.996774842915142401 ) ) ;
#9827=CARTESIAN_POINT ( 'NONE',  ( 12.62499999999998224, -20.24999999999998934, 4.166666666666636765 ) ) ;
#9830=CARTESIAN_POINT ( 'NONE',  ( -13.84439157666246878, 4.204274621457510186, 5.123803251657143676 ) ) ;
#9831=CARTESIAN_POINT ( 'NONE',  ( 8.215308582316795949, -24.52099543870834708, 2.515153566944913432 ) ) ;
#9832=CARTESIAN_POINT ( 'NONE',  ( -12.81251082758882376, -11.53070320674076576, 6.423537912489145185 ) ) ;
#9833=CARTESIAN_POINT ( 'NONE',  ( -11.03469141768317741, -19.47900456129164581, 2.515153566944927199 ) ) ;
#9836=CARTESIAN_POINT ( 'NONE',  ( 7.652808582316796837, -21.53509896474924901, 4.479004561291659137 ) ) ;
#9837=CARTESIAN_POINT ( 'NONE',  ( -5.034691417683179182, -20.22900456129164581, 2.825813738724748170 ) ) ;
#9840=CARTESIAN_POINT ( 'NONE',  ( 13.84501465882535598, 4.235740270674679842, 5.020612255068622076 ) ) ;
#9848=CARTESIAN_POINT ( 'NONE',  ( -13.12529397354238192, 5.014845663890295846, 4.166666666666749563 ) ) ;
#9852=CARTESIAN_POINT ( 'NONE',  ( -13.05696142222617695, 1.564051822406025583, 5.955108176248398166 ) ) ;
#9853=CARTESIAN_POINT ( 'NONE',  ( 4.687312169500630787, -21.51559725698340131, 5.182386163300424009 ) ) ;
#9855=CARTESIAN_POINT ( 'NONE',  ( 13.12270769621861355, 4.884238659038159902, 5.513847264053151065 ) ) ;
#9856=CARTESIAN_POINT ( 'NONE',  ( -1.407845757905374695, -9.114917468222230923, 2.372643865078341019 ) ) ;
#9858=CARTESIAN_POINT ( 'NONE',  ( -13.81626551376501588, 2.033908445126689557, 5.950679699622869911 ) ) ;
#9861=CARTESIAN_POINT ( 'NONE',  ( 4.284691417683177406, -24.52099543870834708, 4.484846433055073689 ) ) ;
#9862=CARTESIAN_POINT ( 'NONE',  ( -9.527808582316795949, -22.97900456129165647, 3.964901035250747885 ) ) ;
#9864=CARTESIAN_POINT ( 'NONE',  ( 12.62499999999998401, -20.99999999999999645, 3.146526952850934755 ) ) ;
#9865=CARTESIAN_POINT ( 'NONE',  ( 13.12463908936614132, 4.981774012991869505, 5.264611377988129171 ) ) ;
#9876=CARTESIAN_POINT ( 'NONE',  ( 1.882415164465650825, -10.11790622164856224, 2.437616430916333510 ) ) ;
#9883=CARTESIAN_POINT ( 'NONE',  ( -3.317048600639548095, -9.800042196285016161, 2.741212564741740465 ) ) ;
#9884=ORIENTED_EDGE ( 'NONE', *, *, #1439, .F. ) ;
#9886=CARTESIAN_POINT ( 'NONE',  ( -12.82182472306881671, -9.560351485048736109, 4.965845106672846399 ) ) ;
#9888=CARTESIAN_POINT ( 'NONE',  ( -4.687312169500634340, -21.70215802671379990, 4.455959925339818106 ) ) ;
#9889=CARTESIAN_POINT ( 'NONE',  ( -8.972191417683177406, -23.72900456129165292, 2.724438792969417822 ) ) ;
#9891=CARTESIAN_POINT ( 'NONE',  ( 13.84501469867711698, 4.235742283194553259, 4.833333333333343695 ) ) ;
#9892=( NAMED_UNIT ( * ) SI_UNIT ( $, .STERADIAN. ) SOLID_ANGLE_UNIT ( ) );
#9893=ORIENTED_EDGE ( 'NONE', *, *, #2951, .F. ) ;
#9902=CARTESIAN_POINT ( 'NONE',  ( -2.559937518207947793, -9.746075135043517079, 2.534737762559237773 ) ) ;
#9904=CARTESIAN_POINT ( 'NONE',  ( -9.059058582316794173, -20.72672167713054137, 4.701595411283463477 ) ) ;
#9906=CARTESIAN_POINT ( 'NONE',  ( 9.909691417683179182, -21.32581373872474373, 5.270995438708348857 ) ) ;
#9909=CARTESIAN_POINT ( 'NONE',  ( -4.378441417683176518, -23.74999999999999645, 3.449312527122335492 ) ) ;
#9910=VERTEX_POINT ( 'NONE', #6439 ) ;
#9911=CARTESIAN_POINT ( 'NONE',  ( 12.24655858231679595, -21.94931252712234127, 6.000000000000001776 ) ) ;
#9912=CARTESIAN_POINT ( 'NONE',  ( 13.02818618459764188, 0.1109023222084986743, 5.923858176248589125 ) ) ;
#9913=CARTESIAN_POINT ( 'NONE',  ( -12.63819864697926754, -19.58346832754827105, 5.450273968536036406 ) ) ;
#9920=ADVANCED_FACE ( 'NONE', ( #17205 ), #16961, .T. ) ;
#9928=CARTESIAN_POINT ( 'NONE',  ( 12.68288333306630378, -17.32689168014509207, 5.548858176248425700 ) ) ;
#9930=CARTESIAN_POINT ( 'NONE',  ( -13.37499999999998224, -20.24999999999998934, 4.166666666666636765 ) ) ;
#9932=CARTESIAN_POINT ( 'NONE',  ( 9.152808582316795949, -20.91377862118960351, 5.979004561291660913 ) ) ;
#9933=CARTESIAN_POINT ( 'NONE',  ( -13.15498530132288479, 5.764257716805535559, 4.791666666666684726 ) ) ;
#9935=CARTESIAN_POINT ( 'NONE',  ( -5.496558582316795949, -22.05068747287764452, 0.9999999999999978906 ) ) ;
#9938=CARTESIAN_POINT ( 'NONE',  ( 11.59030858231679595, -21.63647391050454871, 2.479004561291657804 ) ) ;
#9939=CARTESIAN_POINT ( 'NONE',  ( -6.440941417683176518, -20.72672167713052715, 2.298404588716546293 ) ) ;
#9942=CARTESIAN_POINT ( 'NONE',  ( 13.84501469867711698, 4.235742283194553259, 3.666666666666500873 ) ) ;
#9948=CARTESIAN_POINT ( 'NONE',  ( 13.37500000000002132, -20.25000000000274269, 4.083333333315724012 ) ) ;
#9950=CARTESIAN_POINT ( 'NONE',  ( 3.211992482548209349, -9.366834950279640637, 2.629956289783360823 ) ) ;
#9951=CARTESIAN_POINT ( 'NONE',  ( 1.513434189748285696, -9.114917468222230923, 1.622643865078341463 ) ) ;
#9952=CARTESIAN_POINT ( 'NONE',  ( -13.08573665985359824, 3.017201322601628100, 5.986358176248492313 ) ) ;
#9953=CARTESIAN_POINT ( 'NONE',  ( 5.027808582316793284, -23.72900456129165292, 4.275561207030568411 ) ) ;
#9955=CARTESIAN_POINT ( 'NONE',  ( 13.12529380813666435, 5.014837310896125722, 5.033295791462342628 ) ) ;
#9958=CARTESIAN_POINT ( 'NONE',  ( -1.337453470010121714, -9.114917468222230923, 2.372643865078341019 ) ) ;
#9959=CARTESIAN_POINT ( 'NONE',  ( -13.87470602645761986, 4.985154336109792972, 4.916666666666650087 ) ) ;
#9961=CARTESIAN_POINT ( 'NONE',  ( 9.065941417683177406, -23.20159541128344927, 2.226721677130534705 ) ) ;
#9962=CARTESIAN_POINT ( 'NONE',  ( -6.059058582316795949, -21.25705176302045274, 4.171265325393551215 ) ) ;
#9964=CARTESIAN_POINT ( 'NONE',  ( 13.90434039801927568, 5.731690099970989216, 5.115558489342345361 ) ) ;
#9965=CARTESIAN_POINT ( 'NONE',  ( 13.12529397353891270, 5.014845663890295846, 3.333333333333220239 ) ) ;
#9973=AXIS2_PLACEMENT_3D ( 'NONE', #3422, #14501, #4781 ) ;
#9976=CARTESIAN_POINT ( 'NONE',  ( 1.709849555000590104, -9.864920124259167977, 1.622644547201689713 ) ) ;
#9979=CARTESIAN_POINT ( 'NONE',  ( 13.12211305460728106, -20.60792114491041005, 3.483674240224274410 ) ) ;
#9981=CARTESIAN_POINT ( 'NONE',  ( -9.340308582316794173, -22.67418626127525982, 5.270995438708342640 ) ) ;
#9983=CARTESIAN_POINT ( 'NONE',  ( -1.728780693989796724, -8.364929292255887106, 2.372646901726390478 ) ) ;
#9986=CARTESIAN_POINT ( 'NONE',  ( -12.64917329730235096, -18.27924848622803466, 4.778345106674467324 ) ) ;
#9987=CARTESIAN_POINT ( 'NONE',  ( -8.777808582316792396, -20.27099543870833642, 2.724438792969431589 ) ) ;
#9989=CARTESIAN_POINT ( 'NONE',  ( -5.315941417683176518, -20.79840458871654363, 4.773278322869464851 ) ) ;
#9992=CARTESIAN_POINT ( 'NONE',  ( 13.38090111944825367, -19.20199346786276351, 4.743968713382380464 ) ) ;
#10003=CARTESIAN_POINT ( 'NONE',  ( 7.284691417683176518, -23.77099543870834353, 4.174186261275251830 ) ) ;
#10006=CARTESIAN_POINT ( 'NONE',  ( -13.87490072368896676, 4.990068513505961256, 3.999999999999998224 ) ) ;
#10008=CARTESIAN_POINT ( 'NONE',  ( -4.746558582316793284, -21.94931252712234482, 5.250000000000000888 ) ) ;
#10010=CARTESIAN_POINT ( 'NONE',  ( 9.440941417683177406, -20.72672167713052715, 2.298404588716546293 ) ) ;
#10012=CARTESIAN_POINT ( 'NONE',  ( -10.00344141768317741, -22.05068747287766229, 4.499999999999999112 ) ) ;
#10014=CARTESIAN_POINT ( 'NONE',  ( -10.84030858231679595, -22.98484643305508612, 6.020995438708344416 ) ) ;
#10016=CARTESIAN_POINT ( 'NONE',  ( 12.62499999999998224, -20.24999999999991829, 4.333333333333343695 ) ) ;
#10017=CARTESIAN_POINT ( 'NONE',  ( -12.62745083560477966, -20.12623280195927933, 5.001038150054709419 ) ) ;
#10022=MECHANICAL_DESIGN_GEOMETRIC_PRESENTATION_REPRESENTATION('',(#10367),#3042);
#10027=CARTESIAN_POINT ( 'NONE',  ( 13.37327929115833669, -20.24999999707183207, 3.449077790995325632 ) ) ;
#10031=CARTESIAN_POINT ( 'NONE',  ( 13.11514659413808737, 4.502403003978772134, 5.887634658581065494 ) ) ;
#10034=CARTESIAN_POINT ( 'NONE',  ( 12.62503117662529739, -20.24842558042254836, 4.565011198945062354 ) ) ;
#10037=CARTESIAN_POINT ( 'NONE',  ( 12.90280858231679595, -23.08622137881038938, 1.020995438708339309 ) ) ;
#10038=CARTESIAN_POINT ( 'NONE',  ( -13.10745701327265778, 3.364079170269163921, 6.743850412489304169 ) ) ;
#10040=CARTESIAN_POINT ( 'NONE',  ( -10.94094141768317741, -20.19639159124061933, 1.768074502826635586 ) ) ;
#10046=CARTESIAN_POINT ( 'NONE',  ( 11.77780858231679595, -21.02099543870833998, 3.035098964749253003 ) ) ;
#10047=CARTESIAN_POINT ( 'NONE',  ( -4.284691417683176518, -23.77099543870834353, 4.174186261275251830 ) ) ;
#10051=CARTESIAN_POINT ( 'NONE',  ( 13.87215786865436762, 4.856472367046606564, 5.506273593909547515 ) ) ;
#10061=CARTESIAN_POINT ( 'NONE',  ( 13.54769662923970763, -11.52882022337116119, 5.659013032956382361 ) ) ;
#10064=CARTESIAN_POINT ( 'NONE',  ( 3.173374397671306912, -9.279487642487616483, 2.607523756204581211 ) ) ;
#10065=CARTESIAN_POINT ( 'NONE',  ( 0.2815691515810352930, -9.114917468222230923, 1.622643865078524206 ) ) ;
#10066=CARTESIAN_POINT ( 'NONE',  ( -12.62525331949183105, -19.48720736566255951, 4.581880915780448760 ) ) ;
#10067=CARTESIAN_POINT ( 'NONE',  ( 8.777808582316792396, -20.27099543870833642, 2.724438792969431589 ) ) ;
#10069=CARTESIAN_POINT ( 'NONE',  ( 13.10192273101908000, 3.834597916462216816, 6.003936301248457674 ) ) ;
#10070=CARTESIAN_POINT ( 'NONE',  ( -2.702705060698113115, -10.69015907548275379, 2.777197378435510622 ) ) ;
#10071=CARTESIAN_POINT ( 'NONE',  ( 7.184058582316795949, -21.32873467460644079, 2.757051763020455404 ) ) ;
#10073=CARTESIAN_POINT ( 'NONE',  ( 11.40969141768318096, -21.32581373872474373, 5.270995438708348857 ) ) ;
#10074=CARTESIAN_POINT ( 'NONE',  ( -10.27780858231679595, -21.02099543870833998, 3.035098964749253003 ) ) ;
#10076=CARTESIAN_POINT ( 'NONE',  ( 12.62500000000002132, -21.00000000000274269, 4.083333333315724012 ) ) ;
#10077=CARTESIAN_POINT ( 'NONE',  ( 12.62499999999998401, -19.49999999999998934, 2.439580858552613751 ) ) ;
#10078=CARTESIAN_POINT ( 'NONE',  ( -13.09878990694840795, -19.87505979123735500, 3.486523226841349743 ) ) ;
#10079=ORIENTED_EDGE ( 'NONE', *, *, #8544, .T. ) ;
#10083=CARTESIAN_POINT ( 'NONE',  ( 2.693754455098655409, -9.955255285363838524, 2.600628789231445470 ) ) ;
#10087=CARTESIAN_POINT ( 'NONE',  ( 1.126276606324276619, -9.114917468222230923, 2.372643865078341019 ) ) ;
#10091=CARTESIAN_POINT ( 'NONE',  ( -1.957016269584227031, -9.152392576945766578, 2.382268221639079364 ) ) ;
#10092=CARTESIAN_POINT ( 'NONE',  ( -7.746558582316794173, -21.94931252712234482, 5.250000000000000888 ) ) ;
#10093=CARTESIAN_POINT ( 'NONE',  ( -3.767139617958116471, -12.99583330722436791, 3.561955564372631500 ) ) ;
#10095=CARTESIAN_POINT ( 'NONE',  ( -13.37499999999998224, -19.49999999999991473, 4.333333333333343695 ) ) ;
#10096=CARTESIAN_POINT ( 'NONE',  ( -5.965308582316793284, -20.22900456129164937, 4.174186261275266929 ) ) ;
#10097=CARTESIAN_POINT ( 'NONE',  ( -6.440941417683176518, -20.72672167713052715, 2.298404588716546293 ) ) ;
#10099=CARTESIAN_POINT ( 'NONE',  ( 13.84501469867711698, 4.235742283194553259, 3.666666666666500873 ) ) ;
#10106=B_SPLINE_CURVE_WITH_KNOTS ( 'NONE', 3,
 ( #19929, #13527, #11756, #11957, #19615, #18147, #18248, #2039, #8521, #473, #13216, #16773, #3711, #10091, #16466, #19830, #3911, #10291, #16661, #4121, #18556, #13733, #1093, #5797, #2542, #6000, #12168, #8930, #5693, #20237 ),
 .UNSPECIFIED., .F., .F.,
 ( 4, 2, 2, 2, 2, 2, 2, 2, 2, 2, 2, 2, 2, 2, 4 ),
 ( 0.6078525888943429045, 0.6200887121040892236, 0.6309950902025724950, 0.6419014683010558775, 0.6637142244980225314, 0.7073397368919559502, 0.7509652492858893691, 0.7727780054828560230, 0.7836843835813394055, 0.7945907616798226769, 0.8074288390748337596, 0.8202669164698448423, 0.8459430712598670077, 0.8972953808399113385, 1.000000000000000000 ),
 .UNSPECIFIED. ) ;
#10108=CARTESIAN_POINT ( 'NONE',  ( 4.284691417683176518, -23.77099543870834353, 4.174186261275251830 ) ) ;
#10112=CARTESIAN_POINT ( 'NONE',  ( 3.162271481458107658, -13.95306990448253437, 3.615178062515473911 ) ) ;
#10115=CARTESIAN_POINT ( 'NONE',  ( 13.90439735423812273, 5.734566389025032684, 4.833333333333343695 ) ) ;
#10119=CARTESIAN_POINT ( 'NONE',  ( 10.84719141768317563, -21.22443879296941915, 1.770995438708345748 ) ) ;
#10121=CARTESIAN_POINT ( 'NONE',  ( -6.628441417683177406, -20.99999999999999645, 3.550687472877664952 ) ) ;
#10122=CARTESIAN_POINT ( 'NONE',  ( -9.246558582316795949, -21.94931252712234127, 6.000000000000001776 ) ) ;
#10123=ORIENTED_EDGE ( 'NONE', *, *, #20656, .T. ) ;
#10124=CARTESIAN_POINT ( 'NONE',  ( 12.62499999999998224, -20.25000000000006395, 4.416666666666681174 ) ) ;
#10125=CARTESIAN_POINT ( 'NONE',  ( -13.15452713448031297, 5.741120291255121799, 5.290164123766007087 ) ) ;
#10135=CARTESIAN_POINT ( 'NONE',  ( 13.10012427866737639, 3.743776072700027324, 6.001983176248468332 ) ) ;
#10137=CARTESIAN_POINT ( 'NONE',  ( -1.798207051321043304, -8.367281747657623114, 1.623251059268568053 ) ) ;
#10140=CARTESIAN_POINT ( 'NONE',  ( 12.63819864697926754, -19.58346832754827105, 5.450273968536036406 ) ) ;
#10144=CARTESIAN_POINT ( 'NONE',  ( 12.80905858231679417, -23.80360840875935935, 1.768074502826626260 ) ) ;
#10145=CARTESIAN_POINT ( 'NONE',  ( -12.62524871736568954, -20.23743977303344010, 4.661898514667671023 ) ) ;
#10146=CARTESIAN_POINT ( 'NONE',  ( -9.253441417683177406, -21.94931252712233061, 0.9999999999999978906 ) ) ;
#10149=CARTESIAN_POINT ( 'NONE',  ( 9.809058582316795949, -22.74294823697954016, 2.828734674606448785 ) ) ;
#10150=CARTESIAN_POINT ( 'NONE',  ( -13.87500000000000000, 5.000000000000049738, 4.000000000000000888 ) ) ;
#10153=CARTESIAN_POINT ( 'NONE',  ( 13.85223456079946303, 3.850345320370711644, 5.989742199623227847 ) ) ;
#10160=CARTESIAN_POINT ( 'NONE',  ( 13.85723511636018301, 4.102873376188801657, 5.986996695041598926 ) ) ;
#10164=CARTESIAN_POINT ( 'NONE',  ( 3.292205091070697698, -9.639507599131205140, 2.699984073191874057 ) ) ;
#10166=CARTESIAN_POINT ( 'NONE',  ( -13.05202662408965075, 2.064844516520778939, 5.215845106673912213 ) ) ;
#10169=CARTESIAN_POINT ( 'NONE',  ( 12.72125031657057015, -15.38935901321805133, 5.590524842915047365 ) ) ;
#10171=CARTESIAN_POINT ( 'NONE',  ( 9.621558582316795949, -22.99999999999999645, 3.550687472877652073 ) ) ;
#10172=CARTESIAN_POINT ( 'NONE',  ( 7.284691417683176518, -23.77099543870834353, 4.174186261275252718 ) ) ;
#10173=CARTESIAN_POINT ( 'NONE',  ( -8.215308582316792396, -23.77099543870833998, 2.825813738724734847 ) ) ;
#10175=CARTESIAN_POINT ( 'NONE',  ( 13.12035191997235906, 4.015271958632619764, 6.757839745787993735 ) ) ;
#10176=CARTESIAN_POINT ( 'NONE',  ( 13.04243487821393721, 1.580461349787872782, 5.205428440007538349 ) ) ;
#10186=CARTESIAN_POINT ( 'NONE',  ( 3.047379876266447685, -13.13734219723468755, 3.405682891496055742 ) ) ;
#10189=CARTESIAN_POINT ( 'NONE',  ( 13.37327929115833669, -20.24999999707183207, 3.449077790995325632 ) ) ;
#10191=CARTESIAN_POINT ( 'NONE',  ( -7.465308582316795061, -20.22900456129164937, 4.174186261275266929 ) ) ;
#10192=CARTESIAN_POINT ( 'NONE',  ( -3.528325504133930313, -10.14411005961392398, 2.079576065490765124 ) ) ;
#10194=CARTESIAN_POINT ( 'NONE',  ( -13.37514942709654164, -19.49245393162283690, 4.562067678168288509 ) ) ;
#10195=CARTESIAN_POINT ( 'NONE',  ( -6.340308582316793284, -22.67418626127525982, 5.270995438708342640 ) ) ;
#10197=CARTESIAN_POINT ( 'NONE',  ( -4.847191417683178294, -21.22443879296941915, 1.770995438708345748 ) ) ;
#10199=CARTESIAN_POINT ( 'NONE',  ( 13.37524505148396514, -20.23762490005974968, 4.659512268729234741 ) ) ;
#10209=CARTESIAN_POINT ( 'NONE',  ( 6.815941417683176518, -20.79840458871654363, 4.773278322869464851 ) ) ;
#10212=CARTESIAN_POINT ( 'NONE',  ( 3.564229130755586006, -10.39902496812945465, 2.145043306434553987 ) ) ;
#10213=CARTESIAN_POINT ( 'NONE',  ( -6.996558582316793284, -22.05068747287764452, 1.749999999999998446 ) ) ;
#10214=CARTESIAN_POINT ( 'NONE',  ( 12.62499999999998224, -20.99999999999998934, 4.291666666666699825 ) ) ;
#10216=CARTESIAN_POINT ( 'NONE',  ( 10.28469141768317741, -23.02099543870834353, 3.863526089495429972 ) ) ;
#10217=CARTESIAN_POINT ( 'NONE',  ( -12.62500000000001954, -20.24999999999450040, 3.833333333368183382 ) ) ;
#10218=CARTESIAN_POINT ( 'NONE',  ( -6.347191417683176518, -21.53509896474923835, 2.520995438708346192 ) ) ;
#10219=CARTESIAN_POINT ( 'NONE',  ( -10.18405858231679595, -20.26807450282662160, 1.696391591240633101 ) ) ;
#10221=CARTESIAN_POINT ( 'NONE',  ( 12.62746768552656285, -19.37538188090202596, 4.723115281690125400 ) ) ;
#10222=CARTESIAN_POINT ( 'NONE',  ( -13.12175473207386922, 4.086113969730903683, 6.756475741440692850 ) ) ;
#10230=CARTESIAN_POINT ( 'NONE',  ( 12.93505857549037863, -19.87496680839758056, 3.508858656608841997 ) ) ;
#10233=CARTESIAN_POINT ( 'NONE',  ( 13.12529397354238192, 5.014845663890295846, 4.916666666666650087 ) ) ;
#10234=CARTESIAN_POINT ( 'NONE',  ( -2.887553741010006281, -10.84643174835951207, 2.067331322690557638 ) ) ;
#10239=CARTESIAN_POINT ( 'NONE',  ( 6.246558582316795949, -21.94931252712234127, 6.000000000000001776 ) ) ;
#10240=CARTESIAN_POINT ( 'NONE',  ( -13.02818618459764188, 0.1109023222084986743, 5.923858176248589125 ) ) ;
#10241=CARTESIAN_POINT ( 'NONE',  ( -7.753441417683177406, -21.94931252712233061, 0.9999999999999978906 ) ) ;
#10246=CARTESIAN_POINT ( 'NONE',  ( 11.49655858231679595, -22.05068747287764452, 2.499999999999999112 ) ) ;
#10250=CARTESIAN_POINT ( 'NONE',  ( 13.85723511636018301, 4.102873376188801657, 5.986996695041598926 ) ) ;
#10260=CARTESIAN_POINT ( 'NONE',  ( 13.37499999999998224, -20.24999999999998934, 4.291666666666698937 ) ) ;
#10262=CARTESIAN_POINT ( 'NONE',  ( 3.779650890485476200, -11.92851441922421607, 2.537846752097290715 ) ) ;
#10263=CARTESIAN_POINT ( 'NONE',  ( 1.754777266914451461, -9.116337928146160507, 1.623008667563337726 ) ) ;
#10264=CARTESIAN_POINT ( 'NONE',  ( -13.12529397354238192, 5.014845663890295846, 4.916666666666650087 ) ) ;
#10265=CARTESIAN_POINT ( 'NONE',  ( 6.996558582316793284, -22.05068747287764452, 1.749999999999998446 ) ) ;
#10267=CARTESIAN_POINT ( 'NONE',  ( 12.83635126708105823, -9.576761012430582198, 5.715524842913705328 ) ) ;
#10269=CARTESIAN_POINT ( 'NONE',  ( 8.402808582316797725, -22.46490103525074034, 2.520995438708341307 ) ) ;
#10271=CARTESIAN_POINT ( 'NONE',  ( 6.722191417683177406, -20.27099543870833998, 4.275561207030583510 ) ) ;
#10272=CARTESIAN_POINT ( 'NONE',  ( -10.37155858231679417, -20.24999999999999289, 3.449312527122348371 ) ) ;
#10274=CARTESIAN_POINT ( 'NONE',  ( 13.15452713448031297, 5.741120291255121799, 5.290164123766007087 ) ) ;
#10275=CARTESIAN_POINT ( 'NONE',  ( 12.62500004114794372, -19.49999792202770621, 4.520295319612473328 ) ) ;
#10278=EDGE_LOOP ( 'NONE', ( #17143, #17633, #20298, #19321, #18937 ) ) ;
#10286=CARTESIAN_POINT ( 'NONE',  ( 2.875042468481914248, -11.91375063635796039, 3.091440134965714126 ) ) ;
#10290=CARTESIAN_POINT ( 'NONE',  ( 13.30134771663319704, -20.47916202560290699, 3.458891087130237185 ) ) ;
#10291=CARTESIAN_POINT ( 'NONE',  ( -1.743623630681728542, -9.116095536440919744, 2.372946416531167557 ) ) ;
#10292=CARTESIAN_POINT ( 'NONE',  ( -6.996558582316793284, -22.05068747287764452, 1.749999999999998446 ) ) ;
#10293=CARTESIAN_POINT ( 'NONE',  ( -3.422464802389687311, -10.54865018547243061, 2.933470051312085936 ) ) ;
#10295=CARTESIAN_POINT ( 'NONE',  ( -13.09560264576187905, 4.265433610975056133, 4.583333333333295734 ) ) ;
#10296=CARTESIAN_POINT ( 'NONE',  ( -8.965308582316794173, -20.22900456129164937, 4.174186261275266929 ) ) ;
#10298=CARTESIAN_POINT ( 'NONE',  ( 8.121558582316795949, -24.50000000000000000, 3.550687472877651629 ) ) ;
#10299=CARTESIAN_POINT ( 'NONE',  ( -4.097191417683176518, -22.77556120703057729, 5.229004561291655584 ) ) ;
#10302=CARTESIAN_POINT ( 'NONE',  ( 13.37499979530394967, -20.25001033714808329, 4.458488164327452097 ) ) ;
#10303=DIRECTION ( 'NONE',  ( 0.000000000000000000, 0.2487476929738665354, 0.9685683172808094987 ) ) ;
#10310=CARTESIAN_POINT ( 'NONE',  ( -13.39359219590679295, -19.31109410670777038, 5.491647114909025795 ) ) ;
#10312=CARTESIAN_POINT ( 'NONE',  ( 5.315941417683176518, -20.79840458871654363, 4.773278322869464851 ) ) ;
#10317=CARTESIAN_POINT ( 'NONE',  ( 2.910499702382182807, -8.879427762644468203, 2.504780387061739333 ) ) ;
#10318=CARTESIAN_POINT ( 'NONE',  ( -7.090308582316795061, -21.32581373872472952, 1.729004561291657138 ) ) ;
#10320=CARTESIAN_POINT ( 'NONE',  ( 13.90439735423812273, 5.734566389025032684, 4.333333333333380999 ) ) ;
#10324=CARTESIAN_POINT ( 'NONE',  ( 4.847191417683178294, -21.22443879296941915, 1.770995438708345748 ) ) ;
#10325=CARTESIAN_POINT ( 'NONE',  ( -12.64691428603184242, -19.14332855539073464, 5.509795676248469221 ) ) ;
#10326=CARTESIAN_POINT ( 'NONE',  ( -5.784691417683178294, -23.02099543870834353, 3.863526089495429972 ) ) ;
#10327=CARTESIAN_POINT ( 'NONE',  ( -10.65969141768317741, -22.98484643305507191, 0.9790045612916508100 ) ) ;
#10329=CARTESIAN_POINT ( 'NONE',  ( 12.62958809053144549, -19.26830142816300295, 4.757073430686623361 ) ) ;
#10330=CARTESIAN_POINT ( 'NONE',  ( -13.10192273101908000, 3.834597916462216816, 6.003936301248457674 ) ) ;
#10342=CARTESIAN_POINT ( 'NONE',  ( -3.462011766956747394, -14.92507028461178287, 3.114807177791267812 ) ) ;
#10347=CARTESIAN_POINT ( 'NONE',  ( 9.534691417683177406, -19.47900456129164581, 2.515153566944927199 ) ) ;
#10348=CARTESIAN_POINT ( 'NONE',  ( -13.10012427866737639, 3.743776072700027324, 6.001983176248468332 ) ) ;
#10349=CARTESIAN_POINT ( 'NONE',  ( -7.097191417683176518, -23.08622137881040359, 5.979004561291654696 ) ) ;
#10352=CARTESIAN_POINT ( 'NONE',  ( 12.43405858231679417, -23.20159541128345992, 4.773278322869455970 ) ) ;
#10354=CARTESIAN_POINT ( 'NONE',  ( -13.86796007304617717, 3.894483688830428836, 6.740724019197413597 ) ) ;
#10356=CARTESIAN_POINT ( 'NONE',  ( 4.746558582316795061, -21.94931252712234127, 4.499999999999999112 ) ) ;
#10360=CARTESIAN_POINT ( 'NONE',  ( 13.87470602645761986, 4.985154336109792972, 4.666666666666619889 ) ) ;
#10366=CARTESIAN_POINT ( 'NONE',  ( 13.37499999999998224, -20.24999999999998934, 4.166666666666636765 ) ) ;
#10367=STYLED_ITEM ( 'NONE', ( #299 ), #4794 ) ;
#10369=CARTESIAN_POINT ( 'NONE',  ( 3.321934647848983957, -9.834888441627915867, 2.750161776669472591 ) ) ;
#10373=CARTESIAN_POINT ( 'NONE',  ( -12.62499999999998224, -19.49999999999998934, 4.291666666666699825 ) ) ;
#10375=CARTESIAN_POINT ( 'NONE',  ( 12.52780858231679595, -23.72900456129165647, 4.275561207030568411 ) ) ;
#10376=CARTESIAN_POINT ( 'NONE',  ( -13.41834698511420676, -18.81097725173551893, 6.252442769197418926 ) ) ;
#10379=CARTESIAN_POINT ( 'NONE',  ( 6.527808582316795949, -22.97900456129165647, 3.964901035250747885 ) ) ;
#10381=CARTESIAN_POINT ( 'NONE',  ( 4.284691417683176518, -23.77099543870834353, 4.174186261275252718 ) ) ;
#10382=CARTESIAN_POINT ( 'NONE',  ( -11.87155858231679417, -20.24999999999999289, 3.449312527122348371 ) ) ;
#10385=CARTESIAN_POINT ( 'NONE',  ( 12.66024186180961308, -19.22028597861421417, 6.258173329156003106 ) ) ;
#10386=CARTESIAN_POINT ( 'NONE',  ( 13.07121011584135672, 3.033610849983475521, 5.236678440007632496 ) ) ;
#10398=CARTESIAN_POINT ( 'NONE',  ( 1.407845757905374695, -9.864917468222230923, 2.372643865078341019 ) ) ;
#10403=CARTESIAN_POINT ( 'NONE',  ( -8.402808582316794173, -22.77556120703056308, 1.770995438708339975 ) ) ;
#10404=CARTESIAN_POINT ( 'NONE',  ( -2.887553741010006281, -10.84643174835951207, 2.067331322690557638 ) ) ;
#10406=CARTESIAN_POINT ( 'NONE',  ( -13.37500003877585186, -19.49999804181952712, 4.520055687292853008 ) ) ;
#10407=CARTESIAN_POINT ( 'NONE',  ( -4.717959273841178636, -21.72818306014730183, 5.243595146365860771 ) ) ;
#10408=CARTESIAN_POINT ( 'NONE',  ( 9.434058582316795949, -23.73192549717337130, 5.303608408759367343 ) ) ;
#10409=CARTESIAN_POINT ( 'NONE',  ( -11.59719141768317741, -22.46490103525075810, 4.479004561291653808 ) ) ;
#10411=CARTESIAN_POINT ( 'NONE',  ( 13.85593616229004610, 4.037276195647738319, 5.992122970672676630 ) ) ;
#10412=CARTESIAN_POINT ( 'NONE',  ( 13.50000000000000178, 5.000000000000047962, 4.000000000000000000 ) ) ;
#10417=AXIS2_PLACEMENT_3D ( 'NONE', #10762, #20189, #6056 ) ;
#10419=CARTESIAN_POINT ( 'NONE',  ( -13.39107665282975645, -19.43812903209671461, 5.476542851584349947 ) ) ;
#10420=VECTOR ( 'NONE', #18616, 1000.000000000000000 ) ;
#10428=CARTESIAN_POINT ( 'NONE',  ( 1.337453470010121714, -8.364917468222230923, 2.372643865078341019 ) ) ;
#10429=CARTESIAN_POINT ( 'NONE',  ( -8.309058582316792396, -23.27327832286945153, 2.298404588716537411 ) ) ;
#10430=CARTESIAN_POINT ( 'NONE',  ( 13.87005939078915873, 4.000499234880882327, 6.742989431566016378 ) ) ;
#10432=CARTESIAN_POINT ( 'NONE',  ( 5.222191417683178294, -20.27099543870833998, 4.275561207030583510 ) ) ;
#10433=CARTESIAN_POINT ( 'NONE',  ( -12.62499979224180180, -20.25001049178813162, 4.458178821399696012 ) ) ;
#10434=CARTESIAN_POINT ( 'NONE',  ( -8.409691417683177406, -21.63647391050456648, 4.520995438708348857 ) ) ;
#10436=CARTESIAN_POINT ( 'NONE',  ( -9.534691417683177406, -19.47900456129164581, 2.515153566944927199 ) ) ;
#10438=CARTESIAN_POINT ( 'NONE',  ( 12.62599452815238443, -19.44977632830967806, 4.656396506304353977 ) ) ;
#10439=CARTESIAN_POINT ( 'NONE',  ( -13.12529397354238192, 5.014845663890295846, 4.166666666666765551 ) ) ;
#10444=( BOUNDED_CURVE ( )  B_SPLINE_CURVE ( 3, ( #5025, #17790, #5226, #426 ),
 .UNSPECIFIED., .F., .T. ) 
 B_SPLINE_CURVE_WITH_KNOTS ( ( 4, 4 ),
 ( 0.2500000000000000000, 0.5000000000000000000 ),
 .UNSPECIFIED. ) 
 CURVE ( )  GEOMETRIC_REPRESENTATION_ITEM ( )  RATIONAL_B_SPLINE_CURVE ( ( 0.4833790284681487304, 0.4833790284681486193, 0.6445053712908659360, 0.9667580569362994591 ) ) 
 REPRESENTATION_ITEM ( '' )  );
#10453=CARTESIAN_POINT ( 'NONE',  ( -2.768424032093183662, -10.00067216410020166, 1.850123365707658785 ) ) ;
#10457=CARTESIAN_POINT ( 'NONE',  ( 11.03469141768317741, -19.47900456129164581, 2.515153566944927199 ) ) ;
#10458=CARTESIAN_POINT ( 'NONE',  ( -12.91308523408712183, -5.701695678577235249, 5.798858176249892082 ) ) ;
#10459=CARTESIAN_POINT ( 'NONE',  ( -9.159691417683175629, -22.98484643305507191, 0.9790045612916508100 ) ) ;
#10463=CARTESIAN_POINT ( 'NONE',  ( -13.87486364728600208, 4.243114187942282456, 6.725269602253773016 ) ) ;
#10466=CARTESIAN_POINT ( 'NONE',  ( 12.15280858231679595, -21.22443879296942626, 5.229004561291659137 ) ) ;
#10470=CARTESIAN_POINT ( 'NONE',  ( 13.85593616229004610, 4.037276195647738319, 5.992122970672676630 ) ) ;
#10478=CARTESIAN_POINT ( 'NONE',  ( 1.731569788986178304, -8.364930642962441709, 1.622647248614820015 ) ) ;
#10480=CARTESIAN_POINT ( 'NONE',  ( -13.12529397354238192, 5.014845663890295846, 4.791666666666685614 ) ) ;
#10482=CARTESIAN_POINT ( 'NONE',  ( -13.38795836133016870, -20.34560275282643005, 5.879540349057044146 ) ) ;
#10484=CARTESIAN_POINT ( 'NONE',  ( 11.40280858231679417, -22.77556120703056308, 1.770995438708339975 ) ) ;
#10485=CARTESIAN_POINT ( 'NONE',  ( 5.972191417683179182, -23.72900456129165292, 2.724438792969417822 ) ) ;
#10486=CARTESIAN_POINT ( 'NONE',  ( -12.24655858231679240, -21.94931252712234482, 5.250000000000000888 ) ) ;
#10488=CARTESIAN_POINT ( 'NONE',  ( 13.02352923685845631, -0.8742735386340954040, 6.652704579156702991 ) ) ;
#10489=CARTESIAN_POINT ( 'NONE',  ( 13.08080186171710224, 3.517994016715657146, 5.247095106674282583 ) ) ;
#10491=ORIENTED_EDGE ( 'NONE', *, *, #9784, .F. ) ;
#10496=CARTESIAN_POINT ( 'NONE',  ( -12.64511805349267526, -19.23403829861753422, 5.507852591554869726 ) ) ;
#10499=CARTESIAN_POINT ( 'NONE',  ( 0.9854920305337622199, -9.864917468222230923, 2.372643865078341019 ) ) ;
#10503=CARTESIAN_POINT ( 'NONE',  ( -11.21530858231679595, -24.52099543870834708, 2.515153566944913432 ) ) ;
#10504=CARTESIAN_POINT ( 'NONE',  ( -2.742252025265078608, -15.06657917462210605, 2.958534504914692942 ) ) ;
#10506=CARTESIAN_POINT ( 'NONE',  ( -13.45643611822145225, -15.38747602984844853, 4.825999963382285429 ) ) ;
#10508=CARTESIAN_POINT ( 'NONE',  ( 9.722191417683177406, -19.52099543870834353, 4.586221378810406257 ) ) ;
#10509=CARTESIAN_POINT ( 'NONE',  ( -10.65969141768317741, -22.36352608949543352, 2.479004561291652031 ) ) ;
#10511=CARTESIAN_POINT ( 'NONE',  ( 13.39902456816392906, -19.03675930772010361, 5.497554699623231400 ) ) ;
#10518=CARTESIAN_POINT ( 'NONE',  ( -13.85163507668220539, 3.820071372449974412, 5.989091157956555556 ) ) ;
#10526=CARTESIAN_POINT ( 'NONE',  ( 1.548630333695928618, -8.364917468222230923, 2.372643865078341019 ) ) ;
#10528=CARTESIAN_POINT ( 'NONE',  ( 12.62500000000002132, -21.00000000000274269, 4.083333333315724012 ) ) ;
#10532=CARTESIAN_POINT ( 'NONE',  ( 10.09719141768317741, -22.46490103525075810, 4.479004561291653808 ) ) ;
#10533=CARTESIAN_POINT ( 'NONE',  ( -12.63249216759192350, -19.87164553660301536, 5.297612231341934041 ) ) ;
#10534=CARTESIAN_POINT ( 'NONE',  ( -7.003441417683177406, -22.05068747287766229, 4.499999999999999112 ) ) ;
#10535=CARTESIAN_POINT ( 'NONE',  ( -10.75344141768317741, -21.94931252712233061, 0.9999999999999978906 ) ) ;
#10537=CARTESIAN_POINT ( 'NONE',  ( 13.12503131243110843, 5.001581277770153378, 5.166347330538456184 ) ) ;
#10538=CARTESIAN_POINT ( 'NONE',  ( -13.12529380813666435, 5.014837310896125722, 5.033295791462342628 ) ) ;
#10549=CARTESIAN_POINT ( 'NONE',  ( -2.044552395631970665, -10.13052631352519306, 1.690857522621936226 ) ) ;
#10554=CARTESIAN_POINT ( 'NONE',  ( 6.809058582316796837, -23.80360840875935935, 1.768074502826626260 ) ) ;
#10555=CARTESIAN_POINT ( 'NONE',  ( -12.66369984131459070, -18.29565801360988075, 5.528024842915327142 ) ) ;
#10556=CARTESIAN_POINT ( 'NONE',  ( -7.190941417683177406, -23.80360840875937001, 5.231925497173365081 ) ) ;
#10557=( BOUNDED_CURVE ( )  B_SPLINE_CURVE ( 2, ( #3171, #19184, #6417, #6201, #8090, #15916, #4733, #11319, #14455, #12883, #6301, #19286, #17703, #11121, #3375, #18969, #19076, #4838, #9338, #7876, #4530, #4625, #11018, #9754, #10914, #15714, #17491, #14235, #16139, #1397, #9545, #1593, #3070, #12570, #17388, #9446, #7973, #15817, #14346, #30, #3683, #18011, #8401, #11732, #6726, #14768, #1904, #13193, #17810, #10067, #16440, #14867, #445, #7033, #2012, #14661, #8191, #19691, #16632, #542, #16537, #3476, #17907, #5245, #6824, #5354, #19591, #14557, #10265, #11526, #8287, #19806, #2212, #16238, #18124, #11622, #2115, #8594, #11833, #3885, #6617, #5148, #6921, #14964, #8497, #13290, #342, #3574, #3790, #9953, #13093, #645, #16338, #19496, #9853 ),
 .UNSPECIFIED., .F., .F. ) 
 B_SPLINE_CURVE_WITH_KNOTS ( ( 3, 2, 2, 2, 2, 2, 2, 2, 2, 2, 2, 2, 2, 2, 2, 2, 2, 2, 2, 2, 2, 2, 2, 2, 2, 2, 2, 2, 2, 2, 2, 2, 2, 2, 2, 2, 2, 2, 2, 2, 2, 2, 2, 2, 2, 2, 2, 3 ),
 ( 0.000000000000000000, 0.02083333333333333218, 0.04166666666666666435, 0.06250000000000000000, 0.08333333333333332871, 0.1041666666666666713, 0.1250000000000000000, 0.1458333333333333426, 0.1666666666666666574, 0.1875000000000000000, 0.2083333333333333426, 0.2291666666666666574, 0.2500000000000000000, 0.2708333333333333148, 0.2916666666666666852, 0.3124999999999999445, 0.3333333333333333148, 0.3541666666666666852, 0.3750000000000000000, 0.3958333333333333148, 0.4166666666666666852, 0.4375000000000000555, 0.4583333333333333148, 0.4791666666666666852, 0.5000000000000000000, 0.5208333333333333703, 0.5416666666666666297, 0.5625000000000000000, 0.5833333333333333703, 0.6041666666666666297, 0.6249999999999998890, 0.6458333333333333703, 0.6666666666666666297, 0.6875000000000000000, 0.7083333333333333703, 0.7291666666666666297, 0.7500000000000000000, 0.7708333333333333703, 0.7916666666666666297, 0.8125000000000000000, 0.8333333333333333703, 0.8541666666666666297, 0.8750000000000001110, 0.8958333333333333703, 0.9166666666666666297, 0.9375000000000000000, 0.9583333333333333703, 0.9650437087885355147 ),
 .UNSPECIFIED. ) 
 CURVE ( )  GEOMETRIC_REPRESENTATION_ITEM ( )  RATIONAL_B_SPLINE_CURVE ( ( 1.000000000000000000, 0.9238795325112867385, 1.000000000000000000, 0.9238795325112867385, 1.000000000000000000, 0.9238795325112867385, 1.000000000000000000, 0.9238795325112867385, 1.000000000000000000, 0.9238795325112867385, 1.000000000000000000, 0.9238795325112867385, 1.000000000000000000, 0.9238795325112867385, 1.000000000000000000, 0.9238795325112867385, 1.000000000000000000, 0.9238795325112867385, 1.000000000000000000, 0.9238795325112867385, 1.000000000000000000, 0.9238795325112867385, 1.000000000000000000, 0.9238795325112867385, 1.000000000000000000, 0.9238795325112867385, 1.000000000000000000, 0.9238795325112867385, 1.000000000000000000, 0.9238795325112867385, 1.000000000000000000, 0.9238795325112867385, 1.000000000000000000, 0.9238795325112867385, 1.000000000000000000, 0.9238795325112867385, 1.000000000000000000, 0.9238795325112867385, 1.000000000000000000, 0.9238795325112867385, 1.000000000000000000, 0.9238795325112867385, 1.000000000000000000, 0.9238795325112867385, 1.000000000000000000, 0.9238795325112867385, 1.000000000000000000, 0.9238795325112867385, 1.000000000000000000, 0.9238795325112867385, 1.000000000000000000, 0.9238795325112867385, 1.000000000000000000, 0.9238795325112867385, 1.000000000000000000, 0.9238795325112867385, 1.000000000000000000, 0.9238795325112867385, 1.000000000000000000, 0.9238795325112867385, 1.000000000000000000, 0.9238795325112867385, 1.000000000000000000, 0.9238795325112867385, 1.000000000000000000, 0.9238795325112867385, 1.000000000000000000, 0.9238795325112867385, 1.000000000000000000, 0.9238795325112867385, 1.000000000000000000, 0.9238795325112867385, 1.000000000000000000, 0.9238795325112867385, 1.000000000000000000, 0.9238795325112867385, 1.000000000000000000, 0.9238795325112867385, 1.000000000000000000, 0.9238795325112867385, 1.000000000000000000, 0.9238795325112867385, 1.000000000000000000, 0.9238795325112867385, 1.000000000000000000, 0.9238795325112867385, 1.000000000000000000, 0.9238795325112867385, 1.000000000000000000, 0.9238795325112867385, 1.000000000000000000, 0.9238795325112867385, 1.000000000000000000, 0.9754817479996107377, 0.9667580569362973497 ) ) 
 REPRESENTATION_ITEM ( '' )  );
#10561=CARTESIAN_POINT ( 'NONE',  ( -13.37500027835944039, -20.99998594284889464, 4.544258551573043370 ) ) ;
#10563=CARTESIAN_POINT ( 'NONE',  ( 10.09030858231679595, -21.32581373872472597, 1.729004561291657582 ) ) ;
#10569=CARTESIAN_POINT ( 'NONE',  ( 13.42074492158312715, -18.68988146005270679, 6.255046935864005064 ) ) ;
#10574=FACE_OUTER_BOUND ( 'NONE', #11960, .T. ) ;
#10577=CARTESIAN_POINT ( 'NONE',  ( 2.808565762442263303, -10.28561894962424716, 1.923303392614186924 ) ) ;
#10579=CARTESIAN_POINT ( 'NONE',  ( 2.786182376113650605, -10.12667130264514626, 1.882483419865550900 ) ) ;
#10580=CARTESIAN_POINT ( 'NONE',  ( -13.09560264576187905, 4.265433610975056133, 4.791666666666684726 ) ) ;
#10582=CARTESIAN_POINT ( 'NONE',  ( -13.40322194933353828, -19.57479155865495457, 6.214283636730510096 ) ) ;
#10584=CARTESIAN_POINT ( 'NONE',  ( 12.52780858231679595, -23.72900456129165647, 4.275561207030568411 ) ) ;
#10585=CARTESIAN_POINT ( 'NONE',  ( 6.065941417683177406, -23.20159541128344927, 2.226721677130534705 ) ) ;
#10586=CARTESIAN_POINT ( 'NONE',  ( -10.18405858231679417, -20.79840458871652942, 2.226721677130544030 ) ) ;
#10588=CARTESIAN_POINT ( 'NONE',  ( 12.67794853492974561, -16.82609898603114118, 4.809595106674325216 ) ) ;
#10593=CARTESIAN_POINT ( 'NONE',  ( -13.05696142222617695, 1.564051822406025583, 5.955108176248398166 ) ) ;
#10594=CARTESIAN_POINT ( 'NONE',  ( -2.645259258103298983, -10.28229522185712241, 2.672449792925449596 ) ) ;
#10595=CARTESIAN_POINT ( 'NONE',  ( -13.80667376788930056, 1.549525278393783179, 5.940263032956496048 ) ) ;
#10601=CARTESIAN_POINT ( 'NONE',  ( -9.152808582316795949, -20.91377862118960351, 5.979004561291660913 ) ) ;
#10602=CARTESIAN_POINT ( 'NONE',  ( -1.798207051321043304, -8.367281747657623114, 1.623251059268568053 ) ) ;
#10605=CARTESIAN_POINT ( 'NONE',  ( -13.84501469867711698, 4.235742283194553259, 4.916666666666649199 ) ) ;
#10607=CARTESIAN_POINT ( 'NONE',  ( 9.909691417683175629, -21.01515356694492098, 6.020995438708349745 ) ) ;
#10608=CARTESIAN_POINT ( 'NONE',  ( -8.034691417683175629, -20.97900456129164581, 3.136473910504570917 ) ) ;
#10610=ADVANCED_FACE ( 'NONE', ( #19233 ), #18194, .T. ) ;
#10611=CARTESIAN_POINT ( 'NONE',  ( 13.80667376788930056, 1.549525278393783179, 5.940263032956496048 ) ) ;
#10614=VERTEX_POINT ( 'NONE', #18455 ) ;
#10617=CARTESIAN_POINT ( 'NONE',  ( -13.87470602645761986, 4.985154336109792972, 4.791666666666685614 ) ) ;
#10624=CARTESIAN_POINT ( 'NONE',  ( 3.302240162463773832, -9.695145533921818881, 2.714273006325518711 ) ) ;
#10630=CARTESIAN_POINT ( 'NONE',  ( 4.378441417683176518, -23.74999999999999645, 3.449312527122335492 ) ) ;
#10631=CARTESIAN_POINT ( 'NONE',  ( -12.62515553039088090, -20.24214571525854467, 4.629702272822510345 ) ) ;
#10632=CARTESIAN_POINT ( 'NONE',  ( -9.152808582316795949, -21.53509896474924901, 4.479004561291659137 ) ) ;
#10633=CARTESIAN_POINT ( 'NONE',  ( -8.222191417683175629, -19.52099543870834353, 4.586221378810406257 ) ) ;
#10637=CARTESIAN_POINT ( 'NONE',  ( 13.12512971825177033, 5.006550771716304915, 5.133277049491872468 ) ) ;
#10638=CARTESIAN_POINT ( 'NONE',  ( -13.12463908936614132, 4.981774012991869505, 5.264611377988129171 ) ) ;
#10645=CARTESIAN_POINT ( 'NONE',  ( 1.710927537542899612, -9.866086492083725901, 2.372944093759576933 ) ) ;
#10651=CARTESIAN_POINT ( 'NONE',  ( -0.9854920305337621089, -9.114917468222230923, 1.622643865078341463 ) ) ;
#10657=CARTESIAN_POINT ( 'NONE',  ( 4.746558582316795061, -21.94931252712234127, 6.000000000000001776 ) ) ;
#10658=CARTESIAN_POINT ( 'NONE',  ( -13.10756170493883310, 4.119366099410778581, 6.001761809183453700 ) ) ;
#10659=CARTESIAN_POINT ( 'NONE',  ( -12.53469141768317741, -20.22900456129164581, 2.825813738724747726 ) ) ;
#10661=CARTESIAN_POINT ( 'NONE',  ( 12.24655858231679240, -21.94931252712234482, 5.250000000000000888 ) ) ;
#10663=CARTESIAN_POINT ( 'NONE',  ( -13.71569110726703045, -3.795099083046435506, 6.575359435862661250 ) ) ;
#10666=CARTESIAN_POINT ( 'NONE',  ( 9.996558582316794173, -22.05068747287764452, 1.749999999999998446 ) ) ;
#10671=CARTESIAN_POINT ( 'NONE',  ( 13.79242507427300879, 0.07996625081441015304, 6.658692769197546824 ) ) ;
#10677=CARTESIAN_POINT ( 'NONE',  ( -8.965308582316794173, -20.22900456129164937, 4.174186261275266929 ) ) ;
#10681=CARTESIAN_POINT ( 'NONE',  ( 3.462011766956747394, -14.92507028461178287, 3.114807177791267812 ) ) ;
#10686=CARTESIAN_POINT ( 'NONE',  ( -13.37523871602689596, -19.48794484064217514, 4.577160611493482634 ) ) ;
#10687=CARTESIAN_POINT ( 'NONE',  ( 12.90280858231679773, -22.77556120703056308, 1.770995438708339975 ) ) ;
#10688=CARTESIAN_POINT ( 'NONE',  ( -13.87470602645415063, 4.985154336109792972, 3.333333333332063830 ) ) ;
#10691=CARTESIAN_POINT ( 'NONE',  ( 9.902808582316794173, -22.77556120703056308, 1.770995438708339975 ) ) ;
#10692=CARTESIAN_POINT ( 'NONE',  ( 12.62844141768317741, -20.99999999999999645, 3.550687472877664952 ) ) ;
#10693=CARTESIAN_POINT ( 'NONE',  ( -5.402808582316794173, -22.77556120703056308, 1.770995438708339975 ) ) ;
#10695=CARTESIAN_POINT ( 'NONE',  ( 13.09560264575884503, 4.265433610975056133, 3.333333333333364568 ) ) ;
#10698=VERTEX_POINT ( 'NONE', #1189 ) ;
#10703=CARTESIAN_POINT ( 'NONE',  ( -12.62524871736568954, -20.23743977303344010, 4.661898514667671023 ) ) ;
#10704=CARTESIAN_POINT ( 'NONE',  ( -2.436080212393455735, -9.483920418190111334, 2.467411194204634839 ) ) ;
#10705=CARTESIAN_POINT ( 'NONE',  ( -13.49014615398506045, -14.43511922376608680, 5.596513032956658584 ) ) ;
#10711=CARTESIAN_POINT ( 'NONE',  ( -4.687312169500632564, -21.51559725698341197, 5.182386163300427562 ) ) ;
#10712=CARTESIAN_POINT ( 'NONE',  ( -1.652577328807104839, -9.114908150887895744, 1.622641472200749835 ) ) ;
#10714=CARTESIAN_POINT ( 'NONE',  ( -13.38800411018677572, -19.59329243556743805, 5.436267741224407146 ) ) ;
#10715=MECHANICAL_DESIGN_GEOMETRIC_PRESENTATION_REPRESENTATION('',(#1680),#2036);
#10718=CARTESIAN_POINT ( 'NONE',  ( 10.84719141768317741, -20.91377862118959285, 1.020995438708345082 ) ) ;
#10719=CARTESIAN_POINT ( 'NONE',  ( -9.347191417683177406, -21.53509896474923835, 2.520995438708346192 ) ) ;
#10721=CARTESIAN_POINT ( 'NONE',  ( 13.42793873098995938, -18.32659408500397191, 6.262859435864284841 ) ) ;
#10722=CARTESIAN_POINT ( 'NONE',  ( 12.62499999999998579, -20.24999999999999289, 3.146526952850934755 ) ) ;
#10728=CARTESIAN_POINT ( 'NONE',  ( -13.84264281492353987, 3.365962153638767607, 5.979325532956542233 ) ) ;
#10729=CARTESIAN_POINT ( 'NONE',  ( 1.655860418491166941, -9.114909740826840689, 2.372641880528837621 ) ) ;
#10737=CARTESIAN_POINT ( 'NONE',  ( 0.9854920305337622199, -8.364917468222230923, 1.622643865078341907 ) ) ;
#10739=CARTESIAN_POINT ( 'NONE',  ( 13.10756170493883310, 4.119366099410778581, 6.001761809183453700 ) ) ;
#10743=CARTESIAN_POINT ( 'NONE',  ( 5.315941417683176518, -21.32873467460645145, 4.242948236979555254 ) ) ;
#10744=CARTESIAN_POINT ( 'NONE',  ( -12.65410809543883985, -18.78004118034163739, 5.517608176248461227 ) ) ;
#10745=CARTESIAN_POINT ( 'NONE',  ( -12.05905858231679595, -21.25705176302045274, 4.171265325393551215 ) ) ;
#10746=CARTESIAN_POINT ( 'NONE',  ( -10.28469141768317741, -24.52099543870834708, 4.484846433055073689 ) ) ;
#10748=CARTESIAN_POINT ( 'NONE',  ( 13.05202662408965075, 2.064844516520778939, 5.215845106673912213 ) ) ;
#10754=CARTESIAN_POINT ( 'NONE',  ( 1.939860967060266672, -10.52577007527361808, 2.542364016426418516 ) ) ;
#10760=CARTESIAN_POINT ( 'NONE',  ( -2.155282726790247239, -12.05525952636828357, 2.935167462089139256 ) ) ;
#10762=CARTESIAN_POINT ( 'NONE',  ( 2.693754455098655409, -10.04853567022903782, 2.237415670251142519 ) ) ;
#10767=CARTESIAN_POINT ( 'NONE',  ( 8.034691417683175629, -19.47900456129164581, 2.515153566944927199 ) ) ;
#10768=CARTESIAN_POINT ( 'NONE',  ( -13.12529397354238192, 5.014845663890295846, 3.000000000000000000 ) ) ;
#10769=CARTESIAN_POINT ( 'NONE',  ( -7.378441417683176518, -23.74999999999999645, 3.449312527122335492 ) ) ;
#10771=CARTESIAN_POINT ( 'NONE',  ( 6.809058582316794173, -23.27327832286945153, 2.298404588716537411 ) ) ;
#10773=CARTESIAN_POINT ( 'NONE',  ( -13.42793873098995938, -18.32659408500397191, 6.262859435864284841 ) ) ;
#10776=CARTESIAN_POINT ( 'NONE',  ( 10.37155858231679417, -20.24999999999999289, 3.449312527122348371 ) ) ;
#10780=CARTESIAN_POINT ( 'NONE',  ( 13.45671396861735403, -16.87344458480707843, 6.294109435864141844 ) ) ;
#10785=DIRECTION ( 'NONE',  ( -0.9908228861781570584, 0.1309180808328758994, -0.03362237850931586169 ) ) ;
#10787=CARTESIAN_POINT ( 'NONE',  ( -11.12155858231679417, -23.74999999999999645, 3.550687472877651629 ) ) ;
#10788=CARTESIAN_POINT ( 'NONE',  ( 13.87470586348985258, 4.985146106231644225, 5.033049509202228933 ) ) ;
#10791=CARTESIAN_POINT ( 'NONE',  ( 1.754777266914451461, -9.116337928146160507, 1.623008667563337726 ) ) ;
#10794=CARTESIAN_POINT ( 'NONE',  ( -13.37680511754115287, -19.40884156416817774, 4.692171866446762429 ) ) ;
#10796=CARTESIAN_POINT ( 'NONE',  ( -13.60059015675642513, -9.607697083824668027, 6.450359435862663027 ) ) ;
#10799=CARTESIAN_POINT ( 'NONE',  ( 5.590308582316795949, -21.63647391050454871, 2.479004561291657804 ) ) ;
#10800=CARTESIAN_POINT ( 'NONE',  ( 10.00344141768317741, -22.05068747287766229, 4.499999999999999112 ) ) ;
#10801=CARTESIAN_POINT ( 'NONE',  ( -10.56594141768317741, -23.20159541128344927, 2.226721677130534705 ) ) ;
#10803=CARTESIAN_POINT ( 'NONE',  ( 13.37503747255156306, -19.49810763614315690, 4.531249681074674740 ) ) ;
#10804=CARTESIAN_POINT ( 'NONE',  ( -2.589709240944451096, -9.559844081062008669, 1.736909907557668165 ) ) ;
#10806=ADVANCED_FACE ( 'NONE', ( #9035 ), #6274, .T. ) ;
#10811=CARTESIAN_POINT ( 'NONE',  ( -12.64323021897839006, -19.32937394158751943, 5.504219675487169283 ) ) ;
#10812=CARTESIAN_POINT ( 'NONE',  ( -1.824488249492779879, -9.124319963227819130, 2.375058613629473570 ) ) ;
#10813=CARTESIAN_POINT ( 'NONE',  ( -13.87470602645761986, 4.985154336109792972, 4.583333333333296622 ) ) ;
#10815=CARTESIAN_POINT ( 'NONE',  ( -12.62499999999998224, -20.24999999999998934, 4.291666666666698937 ) ) ;
#10820=CARTESIAN_POINT ( 'NONE',  ( -7.746558582316795949, -21.94931252712234127, 6.000000000000001776 ) ) ;
#10821=CARTESIAN_POINT ( 'NONE',  ( -2.226467333542268445, -8.440126719678968215, 1.641959103308203716 ) ) ;
#10824=CARTESIAN_POINT ( 'NONE',  ( -13.37499999998404121, -20.24999999996810729, 2.793053905886972998 ) ) ;
#10826=CARTESIAN_POINT ( 'NONE',  ( 10.37844141768317741, -24.50000000000000000, 3.449312527122335048 ) ) ;
#10827=CARTESIAN_POINT ( 'NONE',  ( -5.784691417683178294, -23.02099543870834353, 3.863526089495429972 ) ) ;
#10829=CARTESIAN_POINT ( 'NONE',  ( 13.37923893525309715, -20.78593376972237650, 5.366589449429977954 ) ) ;
#10837=CARTESIAN_POINT ( 'NONE',  ( -13.85403523778986390, 3.941279508358651817, 5.991705257707216958 ) ) ;
#10839=CARTESIAN_POINT ( 'NONE',  ( 1.337453470010121714, -9.114917468222230923, 2.372643865078341019 ) ) ;
#10844=CARTESIAN_POINT ( 'NONE',  ( 2.801385037117921861, -10.23463596792102415, 1.910209944425432349 ) ) ;
#10846=CARTESIAN_POINT ( 'NONE',  ( 13.12119116326504908, 4.807653744879115010, 5.626470997801169105 ) ) ;
#10851=CARTESIAN_POINT ( 'NONE',  ( 4.378441417683176518, -22.99999999999999645, 3.449312527122335048 ) ) ;
#10852=CARTESIAN_POINT ( 'NONE',  ( -13.00900269284621302, -0.8578640112522492034, 5.903024842915844062 ) ) ;
#10853=CARTESIAN_POINT ( 'NONE',  ( -8.496558582316795949, -22.05068747287764452, 2.499999999999999112 ) ) ;
#10854=CARTESIAN_POINT ( 'NONE',  ( -4.003441417683175629, -22.05068747287766229, 6.000000000000001776 ) ) ;
#10856=CARTESIAN_POINT ( 'NONE',  ( 13.37499999999998401, -19.49999999999998934, 3.666666666666654084 ) ) ;
#10860=EDGE_LOOP ( 'NONE', ( #9310, #20349, #4312, #7918, #3313 ) ) ;
#10861=CARTESIAN_POINT ( 'NONE',  ( 1.982945319006538032, -10.83166796549307520, 2.620924705558935308 ) ) ;
#10866=CARTESIAN_POINT ( 'NONE',  ( -1.337453470010121714, -9.114917468222230923, 1.622643865078341463 ) ) ;
#10870=CARTESIAN_POINT ( 'NONE',  ( 7.284691417683176518, -24.52099543870834708, 4.484846433055073689 ) ) ;
#10872=CARTESIAN_POINT ( 'NONE',  ( -11.12844141768317741, -20.24999999999999289, 3.550687472877664952 ) ) ;
#10875=CARTESIAN_POINT ( 'NONE',  ( 8.777808582316792396, -20.27099543870833642, 2.724438792969431589 ) ) ;
#10877=CARTESIAN_POINT ( 'NONE',  ( -12.62499999998404299, -20.99999999996810729, 2.793053905886972998 ) ) ;
#10879=CARTESIAN_POINT ( 'NONE',  ( 8.871558582316794173, -20.24999999999999289, 3.449312527122348371 ) ) ;
#10882=CARTESIAN_POINT ( 'NONE',  ( 13.86316420010827777, 3.652292105464413297, 6.735515685864076119 ) ) ;
#10888=CARTESIAN_POINT ( 'NONE',  ( -10.65280858231679240, -21.22443879296942626, 5.229004561291659137 ) ) ;
#10891=CARTESIAN_POINT ( 'NONE',  ( 1.619022621591186928, -8.364917468222230923, 1.622643865078341907 ) ) ;
#10893=CARTESIAN_POINT ( 'NONE',  ( -13.37847682517167947, -19.32442032882675775, 4.733786629989340078 ) ) ;
#10894=CARTESIAN_POINT ( 'NONE',  ( 8.684058582316794173, -20.79840458871652942, 2.226721677130544030 ) ) ;
#10895=CARTESIAN_POINT ( 'NONE',  ( -13.89730118381875279, 5.376209782841177898, 6.083536567043803522 ) ) ;
#10896=EDGE_CURVE ( 'NONE', #17122, #15169, #15543, .T. ) ;
#10898=CARTESIAN_POINT ( 'NONE',  ( 5.684058582316794173, -20.79840458871652942, 2.226721677130544030 ) ) ;
#10899=CARTESIAN_POINT ( 'NONE',  ( 8.128441417683177406, -20.99999999999999645, 3.550687472877664952 ) ) ;
#10900=CARTESIAN_POINT ( 'NONE',  ( -11.87844141768317563, -23.74999999999999645, 3.449312527122335492 ) ) ;
#10903=CARTESIAN_POINT ( 'NONE',  ( 13.09560264576187905, 4.265433610975056133, 4.666666666666618113 ) ) ;
#10905=CARTESIAN_POINT ( 'NONE',  ( -1.548630333695928396, -9.114917468222230923, 1.622643865078341463 ) ) ;
#10909=CARTESIAN_POINT ( 'NONE',  ( -12.62745083560477966, -20.12623280195927933, 5.001038150054709419 ) ) ;
#10910=CARTESIAN_POINT ( 'NONE',  ( -1.407845757905374695, -9.114917468222230923, 2.372643865078341019 ) ) ;
#10911=CARTESIAN_POINT ( 'NONE',  ( -13.87470602645761986, 4.985154336109792972, 4.333333333333382775 ) ) ;
#10914=CARTESIAN_POINT ( 'NONE',  ( 11.12155858231679417, -23.74999999999999645, 3.550687472877651629 ) ) ;
#10916=CARTESIAN_POINT ( 'NONE',  ( 12.62499999999998401, -20.24999999999998934, 2.439580858552613751 ) ) ;
#10918=CARTESIAN_POINT ( 'NONE',  ( -13.27780858231679417, -19.52099543870833642, 2.413778621189609286 ) ) ;
#10919=CARTESIAN_POINT ( 'NONE',  ( -1.896776615114361908, -10.21987218505477024, 2.463803327293850209 ) ) ;
#10921=CARTESIAN_POINT ( 'NONE',  ( -13.84501469867711698, 4.235742283194553259, 4.791666666666684726 ) ) ;
#10923=CARTESIAN_POINT ( 'NONE',  ( 10.65969141768317741, -22.98484643305507191, 0.9790045612916508100 ) ) ;
#10924=CARTESIAN_POINT ( 'NONE',  ( -4.847191417683177406, -21.53509896474923835, 2.520995438708346192 ) ) ;
#10926=CARTESIAN_POINT ( 'NONE',  ( 13.37499999999998224, -21.00000000000006395, 4.416666666666682062 ) ) ;
#10927=CARTESIAN_POINT ( 'NONE',  ( 12.62524871736568954, -20.23743977303344010, 4.661898514667671023 ) ) ;
#10932=CARTESIAN_POINT ( 'NONE',  ( -13.85980676119184629, 4.232741440188380722, 5.965367510457697975 ) ) ;
#10933=CARTESIAN_POINT ( 'NONE',  ( 2.367358971471363649, -9.400572650371021410, 2.446005822389718087 ) ) ;
#10936=CARTESIAN_POINT ( 'NONE',  ( 3.162271481458107658, -13.95306990448253437, 3.615178062515473911 ) ) ;
#10938=CARTESIAN_POINT ( 'NONE',  ( 1.906542528716098417, -8.376716462152538512, 1.625674082428238298 ) ) ;
#10940=CARTESIAN_POINT ( 'NONE',  ( 13.12270769621861355, 4.884238659038159902, 5.513847264053151065 ) ) ;
#10946=CARTESIAN_POINT ( 'NONE',  ( 7.003441417683177406, -22.05068747287766229, 4.499999999999999112 ) ) ;
#10947=CARTESIAN_POINT ( 'NONE',  ( -13.06655316810189227, 2.048434989138931961, 5.965524842914772030 ) ) ;
#10948=CARTESIAN_POINT ( 'NONE',  ( -7.934058582316796837, -22.67126532539354855, 4.242948236979545484 ) ) ;
#10949=CARTESIAN_POINT ( 'NONE',  ( -4.097191417683177406, -23.08622137881040359, 5.979004561291654696 ) ) ;
#10952=CARTESIAN_POINT ( 'NONE',  ( 12.93692567357942202, -3.747753484270499591, 5.090845106672844622 ) ) ;
#10957=CARTESIAN_POINT ( 'NONE',  ( 0.2815691515810352374, -9.864917468222230923, 2.372643865078523540 ) ) ;
#10961=CARTESIAN_POINT ( 'NONE',  ( 8.222191417683175629, -20.27099543870833998, 4.275561207030583510 ) ) ;
#10963=CARTESIAN_POINT ( 'NONE',  ( -1.925499516411631973, -10.42380411186744382, 2.516177120048874283 ) ) ;
#10968=CARTESIAN_POINT ( 'NONE',  ( 12.44094141768317741, -20.72672167713052715, 2.298404588716546293 ) ) ;
#10971=CARTESIAN_POINT ( 'NONE',  ( -11.03469141768318273, -20.22900456129164581, 2.825813738724747726 ) ) ;
#10973=CARTESIAN_POINT ( 'NONE',  ( 6.059058582316793284, -20.72672167713054137, 4.701595411283463477 ) ) ;
#10975=CARTESIAN_POINT ( 'NONE',  ( -13.02352923685845631, -0.8742735386340954040, 6.652704579156702991 ) ) ;
#10977=CARTESIAN_POINT ( 'NONE',  ( 8.777808582316792396, -20.27099543870833642, 2.724438792969431589 ) ) ;
#10987=CARTESIAN_POINT ( 'NONE',  ( -11.77780858231679417, -20.27099543870833642, 2.724438792969431589 ) ) ;
#10988=CARTESIAN_POINT ( 'NONE',  ( 12.62503117662529739, -20.24842558042254836, 4.565011198945062354 ) ) ;
#10990=CARTESIAN_POINT ( 'NONE',  ( 2.031432063436913182, -10.08997855658269671, 1.680444048616273722 ) ) ;
#10993=CARTESIAN_POINT ( 'NONE',  ( -13.07121011584135672, 3.033610849983475521, 5.236678440007632496 ) ) ;
#10995=CARTESIAN_POINT ( 'NONE',  ( 6.246558582316794173, -21.94931252712234482, 5.250000000000000888 ) ) ;
#10996=CARTESIAN_POINT ( 'NONE',  ( -12.64802275499843454, -19.83735087257960927, 6.157588447769994922 ) ) ;
#10999=CARTESIAN_POINT ( 'NONE',  ( 7.090308582316794173, -21.32581373872472597, 1.729004561291657582 ) ) ;
#11001=CARTESIAN_POINT ( 'NONE',  ( 5.690941417683177406, -22.74294823697955081, 4.171265325393542334 ) ) ;
#11002=CARTESIAN_POINT ( 'NONE',  ( -5.965308582316793284, -20.22900456129164937, 4.174186261275266929 ) ) ;
#11004=CARTESIAN_POINT ( 'NONE',  ( 13.37500003877585186, -19.49999804181952712, 4.520055687292853008 ) ) ;
#11005=CARTESIAN_POINT ( 'NONE',  ( -2.309828811027716977, -9.292785183284841821, 1.668323847571005603 ) ) ;
#11014=CARTESIAN_POINT ( 'NONE',  ( -1.932703420524435112, -8.381852853175612239, 2.376993210252662969 ) ) ;
#11016=CARTESIAN_POINT ( 'NONE',  ( 2.739050625766161762, -9.875938058683834342, 1.818089155622620412 ) ) ;
#11018=CARTESIAN_POINT ( 'NONE',  ( 11.30905858231679417, -23.27327832286945153, 2.298404588716537411 ) ) ;
#11021=CARTESIAN_POINT ( 'NONE',  ( 13.14782865898149034, 5.402847278557675104, 6.092770214907355708 ) ) ;
#11022=CARTESIAN_POINT ( 'NONE',  ( -6.715308582316796837, -24.52099543870834708, 2.515153566944913432 ) ) ;
#11023=CARTESIAN_POINT ( 'NONE',  ( -2.196516900615978152, -11.19187256518208784, 1.963432442569047698 ) ) ;
#11026=CARTESIAN_POINT ( 'NONE',  ( -13.39482594849551944, -19.24878960097397140, 5.493002502378098839 ) ) ;
#11028=CARTESIAN_POINT ( 'NONE',  ( 6.065941417683177406, -23.73192549717336064, 1.696391591240623331 ) ) ;
#11029=CARTESIAN_POINT ( 'NONE',  ( -13.27780858231679417, -21.02099543870833998, 3.035098964749253003 ) ) ;
#11031=CARTESIAN_POINT ( 'NONE',  ( 13.37543017851028893, -20.97827598523083026, 4.780017688621249761 ) ) ;
#11045=CARTESIAN_POINT ( 'NONE',  ( 3.506783328160878010, -9.991161114504492957, 2.040295720924476530 ) ) ;
#11050=CARTESIAN_POINT ( 'NONE',  ( -13.18405858231679417, -20.79840458871652942, 2.226721677130544030 ) ) ;
#11051=CARTESIAN_POINT ( 'NONE',  ( -1.904508877737772998, -9.138371295333994837, 2.378667276417936627 ) ) ;
#11052=CARTESIAN_POINT ( 'NONE',  ( 12.80905858231679417, -22.74294823697954016, 2.828734674606448785 ) ) ;
#11053=CARTESIAN_POINT ( 'NONE',  ( -13.11514659413808737, 4.502403003978772134, 5.887634658581065494 ) ) ;
#11054=CARTESIAN_POINT ( 'NONE',  ( -11.21530858231679595, -23.02099543870833998, 3.136473910504556262 ) ) ;
#11055=CARTESIAN_POINT ( 'NONE',  ( -10.84719141768317563, -21.22443879296941915, 1.770995438708345748 ) ) ;
#11057=CARTESIAN_POINT ( 'NONE',  ( 13.09560264576187905, 4.265433610975056133, 4.916666666666649199 ) ) ;
#11070=CARTESIAN_POINT ( 'NONE',  ( 9.347191417683177406, -21.22443879296941915, 1.770995438708345748 ) ) ;
#11072=CARTESIAN_POINT ( 'NONE',  ( -1.743623630681728542, -9.116095536440919744, 2.372946416531167557 ) ) ;
#11074=CARTESIAN_POINT ( 'NONE',  ( -10.93405858231679417, -23.20159541128345992, 4.773278322869455970 ) ) ;
#11075=CARTESIAN_POINT ( 'NONE',  ( 12.25344141768317741, -21.94931252712233061, 1.749999999999998446 ) ) ;
#11077=CARTESIAN_POINT ( 'NONE',  ( -10.56594141768317741, -23.20159541128344927, 2.226721677130534705 ) ) ;
#11079=CARTESIAN_POINT ( 'NONE',  ( 5.590308582316794173, -21.32581373872472597, 1.729004561291657582 ) ) ;
#11080=FACE_OUTER_BOUND ( 'NONE', #10860, .T. ) ;
#11081=CARTESIAN_POINT ( 'NONE',  ( -12.67103257592000176, -18.67535491604046172, 6.269892079155907183 ) ) ;
#11083=CARTESIAN_POINT ( 'NONE',  ( 8.215308582316792396, -23.77099543870833998, 2.825813738724734847 ) ) ;
#11087=FILL_AREA_STYLE ('',( #7538 ) ) ;
#11093=CARTESIAN_POINT ( 'NONE',  ( -8.121558582316792396, -23.74999999999999645, 3.550687472877651629 ) ) ;
#11095=CARTESIAN_POINT ( 'NONE',  ( 12.62499999999998224, -20.24999999999998934, 4.291666666666698937 ) ) ;
#11097=CARTESIAN_POINT ( 'NONE',  ( 1.665360951492234287, -9.864914341757378580, 1.622643062139706993 ) ) ;
#11099=CARTESIAN_POINT ( 'NONE',  ( -13.84501465882535598, 4.235740270674679842, 5.020612255068622076 ) ) ;
#11100=CARTESIAN_POINT ( 'NONE',  ( 13.18405858231679595, -20.26807450282662160, 1.696391591240633101 ) ) ;
#11101=CARTESIAN_POINT ( 'NONE',  ( -12.66383876651304874, -19.03864229108970463, 6.262079579155994224 ) ) ;
#11106=CARTESIAN_POINT ( 'NONE',  ( 8.315941417683177406, -21.32873467460645145, 4.242948236979555254 ) ) ;
#11107=CARTESIAN_POINT ( 'NONE',  ( -5.121558582316794173, -23.74999999999999645, 3.550687472877651629 ) ) ;
#11109=CARTESIAN_POINT ( 'NONE',  ( 13.83710853266996388, 3.836480899831821834, 5.239411421715695738 ) ) ;
#11116=CARTESIAN_POINT ( 'NONE',  ( -3.564229130755586006, -10.39902496812945465, 2.145043306434553987 ) ) ;
#11120=CARTESIAN_POINT ( 'NONE',  ( -13.00900269284621302, -0.8578640112522492034, 5.903024842915844062 ) ) ;
#11121=CARTESIAN_POINT ( 'NONE',  ( 12.15280858231679595, -21.22443879296942626, 5.229004561291660025 ) ) ;
#11123=CARTESIAN_POINT ( 'NONE',  ( 13.15384296923648400, 5.706569946443514674, 5.461568745250741763 ) ) ;
#11124=CARTESIAN_POINT ( 'NONE',  ( 0.000000000000000000, -9.864917468222230923, 1.622643865078341241 ) ) ;
#11126=CARTESIAN_POINT ( 'NONE',  ( -13.87470602645761986, 4.985154336109792972, 3.666666666666500873 ) ) ;
#11129=CARTESIAN_POINT ( 'NONE',  ( 12.15969141768317741, -22.67418626127524917, 1.729004561291651809 ) ) ;
#11130=CARTESIAN_POINT ( 'NONE',  ( -3.944195004867014909, -21.80034658733847053, 4.481176709221804444 ) ) ;
#11132=CARTESIAN_POINT ( 'NONE',  ( 13.87470602645761986, 4.985154336109792972, 4.166666666666765551 ) ) ;
#11133=CARTESIAN_POINT ( 'NONE',  ( 12.62500000000001954, -20.24999999999450040, 3.833333333368183382 ) ) ;
#11141=CARTESIAN_POINT ( 'NONE',  ( -13.12500000000000000, 5.004982103124741677, 3.999999999999983569 ) ) ;
#11144=CARTESIAN_POINT ( 'NONE',  ( 2.747777887823422471, -9.906471667804277459, 1.825930796414880763 ) ) ;
#11149=CARTESIAN_POINT ( 'NONE',  ( -12.62155858231679417, -23.74999999999999645, 3.550687472877651629 ) ) ;
#11150=CARTESIAN_POINT ( 'NONE',  ( -2.109407804498405703, -9.207748739546751438, 2.396484790045401603 ) ) ;
#11151=CARTESIAN_POINT ( 'NONE',  ( 7.940941417683175629, -21.25705176302044208, 2.828734674606458555 ) ) ;
#11152=CARTESIAN_POINT ( 'NONE',  ( -13.12529380813666435, 5.014837310896125722, 5.033295791462342628 ) ) ;
#11153=CARTESIAN_POINT ( 'NONE',  ( -7.277808582316795061, -21.02099543870833998, 3.035098964749253003 ) ) ;
#11155=CARTESIAN_POINT ( 'NONE',  ( -10.94094141768317741, -20.72672167713052715, 2.298404588716546293 ) ) ;
#11157=CARTESIAN_POINT ( 'NONE',  ( 13.37499999999998401, -19.49999999999998934, 3.146526952850934755 ) ) ;
#11158=FILL_AREA_STYLE_COLOUR ( '', #8027 ) ;
#11169=CARTESIAN_POINT ( 'NONE',  ( -1.772926875221950249, -9.883376166076789815, 2.377384427436886494 ) ) ;
#11171=CARTESIAN_POINT ( 'NONE',  ( -11.12155858231679417, -23.74999999999999645, 3.550687472877651629 ) ) ;
#11172=CARTESIAN_POINT ( 'NONE',  ( 5.878441417683177406, -24.50000000000000000, 3.449312527122335048 ) ) ;
#11173=CARTESIAN_POINT ( 'NONE',  ( -12.62844141768317741, -20.99999999999999645, 3.550687472877664952 ) ) ;
#11176=CARTESIAN_POINT ( 'NONE',  ( 7.465308582316795061, -20.22900456129164937, 4.174186261275266929 ) ) ;
#11178=CARTESIAN_POINT ( 'NONE',  ( -12.68302225826488616, -18.06987595762608478, 6.282912912489355683 ) ) ;
#11180=CARTESIAN_POINT ( 'NONE',  ( 6.527808582316794173, -23.72900456129165647, 4.275561207030568411 ) ) ;
#11189=CARTESIAN_POINT ( 'NONE',  ( -6.152808582316793284, -21.22443879296942626, 5.229004561291659137 ) ) ;
#11190=CARTESIAN_POINT ( 'NONE',  ( 12.64571531779736979, -19.20387645123237164, 5.508493592915143289 ) ) ;
#11192=CARTESIAN_POINT ( 'NONE',  ( 2.041623931606483033, -10.12028065167953272, 1.688226231982305370 ) ) ;
#11194=CARTESIAN_POINT ( 'NONE',  ( -13.84476264919594612, 4.223013784394161974, 5.079233071712400793 ) ) ;
#11195=CARTESIAN_POINT ( 'NONE',  ( 5.871558582316794173, -20.24999999999999289, 3.449312527122348371 ) ) ;
#11196=CARTESIAN_POINT ( 'NONE',  ( -13.90258797164900884, 5.643192568275169130, 5.568788873356017355 ) ) ;
#11200=CARTESIAN_POINT ( 'NONE',  ( -5.684058582316795949, -20.26807450282662160, 1.696391591240633101 ) ) ;
#11201=CARTESIAN_POINT ( 'NONE',  ( 8.871558582316794173, -20.24999999999999289, 3.449312527122348371 ) ) ;
#11204=CARTESIAN_POINT ( 'NONE',  ( 13.37155858231679595, -20.99999999999999645, 3.449312527122348371 ) ) ;
#11205=CARTESIAN_POINT ( 'NONE',  ( -9.722191417683177406, -20.27099543870833998, 4.275561207030583510 ) ) ;
#11207=CARTESIAN_POINT ( 'NONE',  ( 13.84495141469777479, 4.232546442235974204, 5.040078719623224401 ) ) ;
#11215=CARTESIAN_POINT ( 'NONE',  ( -1.548630333695928618, -8.364917468222230923, 2.372643865078341019 ) ) ;
#11218=CARTESIAN_POINT ( 'NONE',  ( -13.11145189917479392, 4.315820908324673688, 5.961432613039677086 ) ) ;
#11221=CARTESIAN_POINT ( 'NONE',  ( 13.12405442816082868, 4.202248622120948518, 6.747400073346936367 ) ) ;
#11222=CARTESIAN_POINT ( 'NONE',  ( -1.853238653218509890, -9.965882697426144077, 2.398573752920997837 ) ) ;
#11224=CARTESIAN_POINT ( 'NONE',  ( -13.87367531042247748, 4.933103176334663331, 5.324010972534209074 ) ) ;
#11226=CARTESIAN_POINT ( 'NONE',  ( 5.409691417683178294, -21.01515356694492098, 6.020995438708349745 ) ) ;
#11227=CARTESIAN_POINT ( 'NONE',  ( -6.815941417683177406, -21.32873467460645145, 4.242948236979555254 ) ) ;
#11229=CARTESIAN_POINT ( 'NONE',  ( 12.62505438222622622, -20.99725369757571869, 4.613400783263607252 ) ) ;
#11230=CARTESIAN_POINT ( 'NONE',  ( 12.62499999999998401, -19.49999999999998934, 3.666666666666654084 ) ) ;
#11232=ORIENTED_EDGE ( 'NONE', *, *, #17929, .F. ) ;
#11239=CARTESIAN_POINT ( 'NONE',  ( 1.407845757905374695, -9.114917468222230923, 1.622643865078341463 ) ) ;
#11244=CARTESIAN_POINT ( 'NONE',  ( -12.15280858231679595, -21.22443879296942626, 5.229004561291659137 ) ) ;
#11245=FACE_OUTER_BOUND ( 'NONE', #10278, .T. ) ;
#11246=CARTESIAN_POINT ( 'NONE',  ( 9.715308582316795949, -23.02099543870833998, 3.136473910504556262 ) ) ;
#11247=CARTESIAN_POINT ( 'NONE',  ( -12.62503976493681535, -19.49799187068907713, 4.533161381885315144 ) ) ;
#11248=CARTESIAN_POINT ( 'NONE',  ( -13.18405858231679417, -20.79840458871652942, 2.226721677130544030 ) ) ;
#11249=CARTESIAN_POINT ( 'NONE',  ( -11.31594141768317741, -20.79840458871654363, 4.773278322869464851 ) ) ;
#11251=CARTESIAN_POINT ( 'NONE',  ( 13.37908441539295801, -19.29373702265862889, 4.740102594697787275 ) ) ;
#11259=CARTESIAN_POINT ( 'NONE',  ( 10.65969141768317918, -22.67418626127524917, 1.729004561291651587 ) ) ;
#11262=CARTESIAN_POINT ( 'NONE',  ( -2.623717082130370137, -10.12934627674766830, 2.633169448359191644 ) ) ;
#11264=CARTESIAN_POINT ( 'NONE',  ( -13.37327929115833491, -20.24999999560066399, 3.449077790995343840 ) ) ;
#11265=ADVANCED_FACE ( 'NONE', ( #16694 ), #12561, .T. ) ;
#11266=EDGE_CURVE ( 'NONE', #4517, #11657, #15237, .T. ) ;
#11267=CARTESIAN_POINT ( 'NONE',  ( 12.15969141768317741, -22.67418626127524917, 1.729004561291651809 ) ) ;
#11269=CARTESIAN_POINT ( 'NONE',  ( -4.565941417683176518, -23.20159541128344927, 2.226721677130534705 ) ) ;
#11271=CARTESIAN_POINT ( 'NONE',  ( 12.05905858231679595, -20.19639159124062999, 5.231925497173373074 ) ) ;
#11273=CARTESIAN_POINT ( 'NONE',  ( -12.62499999999998401, -20.99999999999998934, 2.439580858552613751 ) ) ;
#11276=CARTESIAN_POINT ( 'NONE',  ( 5.215308582316793284, -23.77099543870833998, 2.825813738724734847 ) ) ;
#11284=CARTESIAN_POINT ( 'NONE',  ( -5.496558582316794173, -22.05068747287764452, 1.749999999999998446 ) ) ;
#11288=CARTESIAN_POINT ( 'NONE',  ( 1.776440835594205847, -9.874406767442327038, 1.625080906685880233 ) ) ;
#11289=CARTESIAN_POINT ( 'NONE',  ( 12.79798428357658047, -11.51429367935891790, 5.673858176248284479 ) ) ;
#11291=CARTESIAN_POINT ( 'NONE',  ( -13.83710853266996388, 3.836480899831821834, 5.239411421715695738 ) ) ;
#11292=CARTESIAN_POINT ( 'NONE',  ( 7.559058582316794173, -20.72672167713054137, 4.701595411283463477 ) ) ;
#11293=CARTESIAN_POINT ( 'NONE',  ( -13.90439735423812273, 5.734566389025032684, 4.833333333333343695 ) ) ;
#11295=CARTESIAN_POINT ( 'NONE',  ( -8.777808582316797725, -19.52099543870833642, 2.413778621189609286 ) ) ;
#11296=CARTESIAN_POINT ( 'NONE',  ( 6.340308582316793284, -22.67418626127525982, 5.270995438708342640 ) ) ;
#11298=CARTESIAN_POINT ( 'NONE',  ( 8.878441417683177406, -22.99999999999999645, 3.449312527122335048 ) ) ;
#11299=CARTESIAN_POINT ( 'NONE',  ( -8.503441417683177406, -22.05068747287765873, 5.250000000000000888 ) ) ;
#11303=CARTESIAN_POINT ( 'NONE',  ( 13.37499999999998224, -20.24999999999998934, 4.291666666666698937 ) ) ;
#11314=CARTESIAN_POINT ( 'NONE',  ( -1.619022621591186928, -8.364917468222230923, 2.372643865078341019 ) ) ;
#11315=CARTESIAN_POINT ( 'NONE',  ( 1.655860418491166941, -9.114909740826840689, 2.372641880528837621 ) ) ;
#11318=CARTESIAN_POINT ( 'NONE',  ( -12.74043380832193684, -14.42059267975384529, 5.611358176248560703 ) ) ;
#11319=CARTESIAN_POINT ( 'NONE',  ( 12.71530858231679417, -23.77099543870833998, 2.825813738724734847 ) ) ;
#11321=CARTESIAN_POINT ( 'NONE',  ( 12.62499999999998224, -20.24999999999998934, 4.166666666666636765 ) ) ;
#11322=CARTESIAN_POINT ( 'NONE',  ( -1.337453470010121714, -9.864917468222230923, 1.622643865078341907 ) ) ;
#11323=EDGE_LOOP ( 'NONE', ( #9893, #15110, #15951, #3491, #6070 ) ) ;
#11324=CARTESIAN_POINT ( 'NONE',  ( -13.87470602645761986, 4.985154336109792972, 4.583333333333296622 ) ) ;
#11326=CARTESIAN_POINT ( 'NONE',  ( 7.097191417683176518, -23.08622137881040359, 5.979004561291654696 ) ) ;
#11327=CARTESIAN_POINT ( 'NONE',  ( -10.37155858231679595, -20.99999999999999645, 3.449312527122348371 ) ) ;
#11329=CARTESIAN_POINT ( 'NONE',  ( 13.86796007304617717, 3.894483688830428836, 6.740724019197413597 ) ) ;
#11330=CARTESIAN_POINT ( 'NONE',  ( 13.12529397354238192, 5.014845663890295846, 4.916666666666650087 ) ) ;
#11331=CIRCLE ( 'NONE', #1644, 0.3749999999999997224 ) ;
#11341=CARTESIAN_POINT ( 'NONE',  ( 1.865667289525601680, -9.999006358835732300, 2.407080570882605297 ) ) ;
#11345=CARTESIAN_POINT ( 'NONE',  ( 13.12529397354238192, 5.014845663890297622, 3.999999999999981792 ) ) ;
#11348=CARTESIAN_POINT ( 'NONE',  ( -3.277163086644854229, -14.76879761173520578, 3.824673233536266537 ) ) ;
#11350=CARTESIAN_POINT ( 'NONE',  ( -12.62515856830665584, -19.49199230051052822, 4.565864671500353467 ) ) ;
#11351=CARTESIAN_POINT ( 'NONE',  ( -5.684058582316795949, -21.32873467460644079, 2.757051763020455404 ) ) ;
#11354=CARTESIAN_POINT ( 'NONE',  ( -7.753441417683176518, -21.94931252712233061, 1.749999999999998446 ) ) ;
#11356=CARTESIAN_POINT ( 'NONE',  ( 13.82811627091129836, 3.382371681020614584, 5.229645796715683304 ) ) ;
#11365=CARTESIAN_POINT ( 'NONE',  ( 11.31594141768317741, -20.79840458871654363, 4.773278322869464851 ) ) ;
#11368=CARTESIAN_POINT ( 'NONE',  ( -1.732184490400474175, -9.869581059509965115, 2.373841568485653308 ) ) ;
#11369=CARTESIAN_POINT ( 'NONE',  ( 2.367358971471363649, -9.400572650371021410, 2.446005822389718087 ) ) ;
#11372=CARTESIAN_POINT ( 'NONE',  ( 9.628441417683177406, -20.24999999999999289, 3.550687472877664952 ) ) ;
#11374=CARTESIAN_POINT ( 'NONE',  ( -4.940941417683177406, -20.72672167713052715, 2.298404588716546293 ) ) ;
#11376=CARTESIAN_POINT ( 'NONE',  ( 9.059058582316795949, -20.19639159124062999, 5.231925497173373074 ) ) ;
#11377=CARTESIAN_POINT ( 'NONE',  ( 13.11145189917479392, 4.315820908324673688, 5.961432613039677086 ) ) ;
#11378=CARTESIAN_POINT ( 'NONE',  ( -13.12860732321105139, 4.432169822159808703, 6.709107302035562270 ) ) ;
#11390=CARTESIAN_POINT ( 'NONE',  ( 13.37499999932878048, -20.20702557250647047, 3.448843586020831964 ) ) ;
#11393=CARTESIAN_POINT ( 'NONE',  ( -13.18405858231679595, -20.26807450282662160, 1.696391591240633101 ) ) ;
#11397=CARTESIAN_POINT ( 'NONE',  ( 12.64691428603184242, -19.14332855539073464, 5.509795676248469221 ) ) ;
#11399=CARTESIAN_POINT ( 'NONE',  ( -13.84501469867711698, 4.235742283194553259, 4.333333333333380999 ) ) ;
#11400=CARTESIAN_POINT ( 'NONE',  ( 12.15280858231679950, -20.91377862118960351, 5.979004561291660913 ) ) ;
#11401=CARTESIAN_POINT ( 'NONE',  ( -12.73577686058281344, -15.40576854059989920, 6.340204579155907183 ) ) ;
#11402=CARTESIAN_POINT ( 'NONE',  ( -11.97219141768317918, -24.47900456129165292, 2.413778621189595963 ) ) ;
#11406=CARTESIAN_POINT ( 'NONE',  ( 8.871558582316795949, -20.99999999999999645, 3.449312527122348371 ) ) ;
#11407=CARTESIAN_POINT ( 'NONE',  ( -7.003441417683177406, -22.05068747287765873, 5.250000000000000888 ) ) ;
#11410=CARTESIAN_POINT ( 'NONE',  ( 13.76337198624852398, 0.1127853055781036368, 5.159333296715827188 ) ) ;
#11416=CARTESIAN_POINT ( 'NONE',  ( -3.944195004867014909, -21.61378581760806128, 5.207602947182413011 ) ) ;
#11420=CARTESIAN_POINT ( 'NONE',  ( -13.12526104302547836, 5.013182672784613381, 5.066812735559260261 ) ) ;
#11422=CARTESIAN_POINT ( 'NONE',  ( -3.521144778809589315, -10.09312707791070096, 2.066482617302010105 ) ) ;
#11424=CARTESIAN_POINT ( 'NONE',  ( -13.10252221513633941, 3.864871864382954048, 6.004587342915129966 ) ) ;
#11427=CARTESIAN_POINT ( 'NONE',  ( 13.02818618459764188, 0.1109023222084986743, 5.923858176248589125 ) ) ;
#11431=CARTESIAN_POINT ( 'NONE',  ( -13.54769662923970763, -11.52882022337116119, 5.659013032956382361 ) ) ;
#11434=CARTESIAN_POINT ( 'NONE',  ( 8.503441417683177406, -22.05068747287766229, 6.000000000000001776 ) ) ;
#11435=CARTESIAN_POINT ( 'NONE',  ( -6.902808582316795949, -22.46490103525074034, 2.520995438708341307 ) ) ;
#11437=CARTESIAN_POINT ( 'NONE',  ( 13.84997554952896515, 2.986265251207539606, 6.721192769197450012 ) ) ;
#11438=CARTESIAN_POINT ( 'NONE',  ( 13.12270769621861355, 4.884238659038159902, 5.513847264053151065 ) ) ;
#11448=CARTESIAN_POINT ( 'NONE',  ( 13.87500000000000000, 5.000000000000049738, 4.000000000000001776 ) ) ;
#11449=CARTESIAN_POINT ( 'NONE',  ( 1.866357130655357688, -10.00562759449716133, 2.408781036472938730 ) ) ;
#11455=CARTESIAN_POINT ( 'NONE',  ( -1.619022621591187150, -9.114917468222230923, 2.372643865078341019 ) ) ;
#11457=CARTESIAN_POINT ( 'NONE',  ( -13.09106898171683930, 4.036483576700608644, 5.256123545019964816 ) ) ;
#11458=CARTESIAN_POINT ( 'NONE',  ( -5.590308582316795949, -21.63647391050454871, 2.479004561291657804 ) ) ;
#11461=CARTESIAN_POINT ( 'NONE',  ( -9.628441417683177406, -20.24999999999999289, 3.550687472877664952 ) ) ;
#11464=CARTESIAN_POINT ( 'NONE',  ( 13.84501469867711698, 4.235742283194553259, 4.916666666666649199 ) ) ;
#11472=MANIFOLD_SOLID_BREP ( 'Mirror1', #14638 ) ;
#11474=CARTESIAN_POINT ( 'NONE',  ( 4.003441417683176518, -22.05068747287765873, 5.250000000000000888 ) ) ;
#11477=CARTESIAN_POINT ( 'NONE',  ( -0.2815691515810352374, -9.864917468222230923, 2.372643865078523540 ) ) ;
#11478=CARTESIAN_POINT ( 'NONE',  ( 1.957016269584227031, -9.152392576945766578, 2.382268221639079364 ) ) ;
#11479=CARTESIAN_POINT ( 'NONE',  ( -9.246558582316794173, -21.94931252712234482, 5.250000000000000888 ) ) ;
#11481=CARTESIAN_POINT ( 'NONE',  ( 10.00344141768317563, -22.05068747287765873, 5.250000000000000888 ) ) ;
#11483=CARTESIAN_POINT ( 'NONE',  ( -5.128441417683177406, -20.24999999999999289, 3.550687472877664952 ) ) ;
#11486=CARTESIAN_POINT ( 'NONE',  ( 10.65280858231679595, -20.91377862118960351, 5.979004561291660913 ) ) ;
#11487=CARTESIAN_POINT ( 'NONE',  ( 12.62515553039088090, -20.24214571525854467, 4.629702272822510345 ) ) ;
#11488=CARTESIAN_POINT ( 'NONE',  ( -13.11704875914858270, 3.848462337001107070, 6.754267079155989784 ) ) ;
#11497=CARTESIAN_POINT ( 'NONE',  ( -13.37155858231679595, -19.49999999999998934, 3.449312527122348371 ) ) ;
#11499=CARTESIAN_POINT ( 'NONE',  ( 13.12529397354238192, 5.014845663890295846, 4.333333333333374782 ) ) ;
#11502=CARTESIAN_POINT ( 'NONE',  ( 13.00900269284621302, -0.8578640112522492034, 5.903024842915844062 ) ) ;
#11504=CARTESIAN_POINT ( 'NONE',  ( -13.82811627091129836, 3.382371681020614584, 5.229645796715683304 ) ) ;
#11505=CARTESIAN_POINT ( 'NONE',  ( 13.09030858231679417, -21.01515356694490322, 0.9790045612916562501 ) ) ;
#11506=CARTESIAN_POINT ( 'NONE',  ( -13.11345185444515415, 3.666818649476655700, 6.750360829155977349 ) ) ;
#11507=CARTESIAN_POINT ( 'NONE',  ( -6.621558582316796837, -24.50000000000000000, 3.550687472877651629 ) ) ;
#11510=CARTESIAN_POINT ( 'NONE',  ( 10.74655858231679595, -21.94931252712234127, 4.499999999999999112 ) ) ;
#11511=CARTESIAN_POINT ( 'NONE',  ( -5.690941417683176518, -23.27327832286946219, 4.701595411283453707 ) ) ;
#11514=CARTESIAN_POINT ( 'NONE',  ( 13.84501474873290938, 4.235744811019327649, 4.974109985360144037 ) ) ;
#11519=CARTESIAN_POINT ( 'NONE',  ( 13.39170256340046095, -19.40652054827866380, 5.481861153867630065 ) ) ;
#11523=CARTESIAN_POINT ( 'NONE',  ( 0.000000000000000000, -9.114917468222230923, 1.622643865078341019 ) ) ;
#11525=CARTESIAN_POINT ( 'NONE',  ( -12.66369984131459070, -18.29565801360988075, 5.528024842915327142 ) ) ;
#11526=CARTESIAN_POINT ( 'NONE',  ( 6.902808582316795061, -22.77556120703056308, 1.770995438708340197 ) ) ;
#11528=CARTESIAN_POINT ( 'NONE',  ( 13.06655316810189227, 2.048434989138931961, 5.965524842914772030 ) ) ;
#11529=CARTESIAN_POINT ( 'NONE',  ( -1.337453470010121714, -9.864917468222230923, 2.372643865078341019 ) ) ;
#11532=CARTESIAN_POINT ( 'NONE',  ( -13.87454419214980739, 4.976981703567351367, 5.131312659523921127 ) ) ;
#11534=CARTESIAN_POINT ( 'NONE',  ( 10.84719141768317563, -21.22443879296941915, 1.770995438708345748 ) ) ;
#11535=CARTESIAN_POINT ( 'NONE',  ( -7.184058582316795949, -21.32873467460644079, 2.757051763020455404 ) ) ;
#11536=VERTEX_POINT ( 'NONE', #16272 ) ;
#11537=CARTESIAN_POINT ( 'NONE',  ( 12.62500000000002132, -20.99999999999450395, 3.833333333368183382 ) ) ;
#11538=CARTESIAN_POINT ( 'NONE',  ( 12.64571531779736979, -19.20387645123237164, 5.508493592915143289 ) ) ;
#11548=CARTESIAN_POINT ( 'NONE',  ( 2.049450250860079592, -10.15122911285664564, 1.696174415070213382 ) ) ;
#11551=CARTESIAN_POINT ( 'NONE',  ( 12.62672070884157804, -20.24999999999983658, 3.550922209436377042 ) ) ;
#11553=CARTESIAN_POINT ( 'NONE',  ( -9.902808582316794173, -22.77556120703056308, 1.770995438708339975 ) ) ;
#11554=CARTESIAN_POINT ( 'NONE',  ( -3.270401025279431995, -9.547343748290430199, 2.676314555138040063 ) ) ;
#11556=CARTESIAN_POINT ( 'NONE',  ( -12.62525331949183105, -19.48720736566255951, 4.581880915780448760 ) ) ;
#11557=CARTESIAN_POINT ( 'NONE',  ( -5.496558582316795949, -22.05068747287764452, 2.499999999999999112 ) ) ;
#11558=CARTESIAN_POINT ( 'NONE',  ( -10.19094141768317563, -23.27327832286946219, 4.701595411283453707 ) ) ;
#11560=CARTESIAN_POINT ( 'NONE',  ( 13.74418849449709512, -0.8559810278826442964, 5.138499963383082125 ) ) ;
#11573=CARTESIAN_POINT ( 'NONE',  ( -13.87500000000000000, 4.995017896875348917, 3.999999999999998224 ) ) ;
#11575=CARTESIAN_POINT ( 'NONE',  ( -8.027808582316792396, -23.72900456129165292, 4.275561207030568411 ) ) ;
#11578=CARTESIAN_POINT ( 'NONE',  ( 10.19094141768317563, -23.27327832286946219, 4.701595411283453707 ) ) ;
#11580=CARTESIAN_POINT ( 'NONE',  ( -4.097191417683176518, -22.77556120703057729, 5.229004561291655584 ) ) ;
#11582=CARTESIAN_POINT ( 'NONE',  ( 10.84030858231679595, -22.98484643305508612, 6.020995438708344416 ) ) ;
#11583=CARTESIAN_POINT ( 'NONE',  ( 13.10252221513633941, 3.864871864382954048, 6.004587342915129966 ) ) ;
#11584=CARTESIAN_POINT ( 'NONE',  ( -13.12035191997235906, 4.015271958632619764, 6.757839745787993735 ) ) ;
#11588=CARTESIAN_POINT ( 'NONE',  ( 13.12499999999999645, 5.000000000000047073, 3.999999999999996447 ) ) ;
#11597=CARTESIAN_POINT ( 'NONE',  ( 12.62562019941893432, -20.21867992933967173, 4.757612834768309540 ) ) ;
#11599=CIRCLE ( 'NONE', #6966, 0.3750000000000003331 ) ;
#11600=CARTESIAN_POINT ( 'NONE',  ( 7.934058582316796837, -23.73192549717337130, 5.303608408759367343 ) ) ;
#11601=CARTESIAN_POINT ( 'NONE',  ( -13.11862022235054503, 3.927821228673052723, 6.755987001683414483 ) ) ;
#11602=CARTESIAN_POINT ( 'NONE',  ( -11.31594141768317741, -20.26807450282663225, 5.303608408759377113 ) ) ;
#11606=CARTESIAN_POINT ( 'NONE',  ( 9.996558582316795949, -22.05068747287764452, 2.499999999999999112 ) ) ;
#11607=CARTESIAN_POINT ( 'NONE',  ( -4.472191417683177406, -23.72900456129164937, 2.724438792969417378 ) ) ;
#11610=CARTESIAN_POINT ( 'NONE',  ( 13.39722611581222189, -19.12758115148224647, 5.495601574623241170 ) ) ;
#11617=CARTESIAN_POINT ( 'NONE',  ( 13.44218742460511073, -16.85703505742523234, 5.544429699623282914 ) ) ;
#11619=CARTESIAN_POINT ( 'NONE',  ( 0.2815691515810352930, -9.114917468222230923, 2.372643865078523984 ) ) ;
#11621=CARTESIAN_POINT ( 'NONE',  ( -13.12529397354238192, 5.014845663890295846, 3.666666666666500873 ) ) ;
#11622=CARTESIAN_POINT ( 'NONE',  ( 6.340308582316794173, -22.67418626127525982, 5.270995438708342640 ) ) ;
#11624=CARTESIAN_POINT ( 'NONE',  ( 12.64323021897839006, -19.32937394158751943, 5.504219675487169283 ) ) ;
#11626=CARTESIAN_POINT ( 'NONE',  ( -1.619022621591187150, -9.114917468222230923, 2.372643865078341019 ) ) ;
#11627=CARTESIAN_POINT ( 'NONE',  ( 7.840308582316795949, -22.36352608949544418, 4.520995438708343528 ) ) ;
#11628=CARTESIAN_POINT ( 'NONE',  ( 9.534691417683177406, -20.22900456129164581, 2.825813738724747726 ) ) ;
#11629=CARTESIAN_POINT ( 'NONE',  ( -8.309058582316795949, -22.74294823697954016, 2.828734674606448785 ) ) ;
#11631=CARTESIAN_POINT ( 'NONE',  ( 13.87005939078915873, 4.000499234880882327, 6.742989431566016378 ) ) ;
#11632=CARTESIAN_POINT ( 'NONE',  ( 13.09532840572934376, 3.501584489333809724, 5.996774842915142401 ) ) ;
#11645=CARTESIAN_POINT ( 'NONE',  ( 2.567175533087980188, -9.771398394011347577, 2.541241281345096859 ) ) ;
#11650=CARTESIAN_POINT ( 'NONE',  ( -10.18405858231679417, -20.79840458871652942, 2.226721677130544030 ) ) ;
#11651=CARTESIAN_POINT ( 'NONE',  ( -3.321934647848983957, -9.834888441627915867, 2.750161776669472591 ) ) ;
#11653=CARTESIAN_POINT ( 'NONE',  ( -13.05202662408965075, 2.064844516520778939, 5.215845106673912213 ) ) ;
#11654=CARTESIAN_POINT ( 'NONE',  ( -8.684058582316794173, -20.79840458871652942, 2.226721677130544030 ) ) ;
#11655=CARTESIAN_POINT ( 'NONE',  ( -9.347191417683177406, -21.22443879296941915, 1.770995438708345748 ) ) ;
#11657=VERTEX_POINT ( 'NONE', #7381 ) ;
#11658=CARTESIAN_POINT ( 'NONE',  ( 13.76337198624852398, 0.1127853055781036368, 5.159333296715827188 ) ) ;
#11661=CARTESIAN_POINT ( 'NONE',  ( -13.50000000000000178, 5.000000000000047962, 2.000000000000000000 ) ) ;
#11666=CARTESIAN_POINT ( 'NONE',  ( 5.222191417683177406, -20.27099543870833998, 4.275561207030583510 ) ) ;
#11671=CARTESIAN_POINT ( 'NONE',  ( -8.215308582316792396, -23.77099543870833998, 2.825813738724734847 ) ) ;
#11674=CARTESIAN_POINT ( 'NONE',  ( 8.409691417683177406, -21.32581373872474373, 5.270995438708348857 ) ) ;
#11676=CARTESIAN_POINT ( 'NONE',  ( -5.409691417683178294, -21.63647391050456648, 4.520995438708348857 ) ) ;
#11677=CARTESIAN_POINT ( 'NONE',  ( -7.840308582316795949, -22.98484643305508612, 6.020995438708344416 ) ) ;
#11679=CARTESIAN_POINT ( 'NONE',  ( 12.65410809543883985, -18.78004118034163739, 5.517608176248461227 ) ) ;
#11680=CARTESIAN_POINT ( 'NONE',  ( -13.10985494974158705, 3.485174961951963191, 6.746454579156001330 ) ) ;
#11689=VERTEX_POINT ( 'NONE', #15112 ) ;
#11691=CARTESIAN_POINT ( 'NONE',  ( 13.27375163337954156, -19.99368846338235883, 3.462660621537502870 ) ) ;
#11694=CARTESIAN_POINT ( 'NONE',  ( 13.12529418130016445, 5.014856155665242454, 4.958178834604180629 ) ) ;
#11699=CARTESIAN_POINT ( 'NONE',  ( 12.62499979224180180, -20.25001049178813162, 4.458178821399696012 ) ) ;
#11702=CARTESIAN_POINT ( 'NONE',  ( 10.27780858231679595, -19.52099543870833642, 2.413778621189609286 ) ) ;
#11703=CARTESIAN_POINT ( 'NONE',  ( -13.14782865898149034, 5.402847278557675104, 6.092770214907355708 ) ) ;
#11705=CARTESIAN_POINT ( 'NONE',  ( -6.340308582316796837, -22.98484643305508612, 6.020995438708344416 ) ) ;
#11709=CARTESIAN_POINT ( 'NONE',  ( 9.902808582316795949, -22.46490103525074034, 2.520995438708341307 ) ) ;
#11715=CARTESIAN_POINT ( 'NONE',  ( 13.44218742460511073, -16.85703505742523234, 5.544429699623282914 ) ) ;
#11724=CARTESIAN_POINT ( 'NONE',  ( 13.85528666703740619, 4.004476685417483139, 5.993048563355776182 ) ) ;
#11728=CARTESIAN_POINT ( 'NONE',  ( 1.619022621591186928, -8.364917468222230923, 2.372643865078341019 ) ) ;
#11731=CARTESIAN_POINT ( 'NONE',  ( -12.63598464672302590, -18.94527534048458151, 4.764022190007618285 ) ) ;
#11732=CARTESIAN_POINT ( 'NONE',  ( 9.340308582316794173, -22.67418626127525982, 5.270995438708342640 ) ) ;
#11734=CARTESIAN_POINT ( 'NONE',  ( 12.65410809543883985, -18.78004118034163739, 5.517608176248461227 ) ) ;
#11735=CARTESIAN_POINT ( 'NONE',  ( -2.583953725994688533, -9.847075946378776479, 2.560676788604062004 ) ) ;
#11736=CARTESIAN_POINT ( 'NONE',  ( 10.93405858231679595, -22.67126532539354855, 4.242948236979545484 ) ) ;
#11738=CARTESIAN_POINT ( 'NONE',  ( 8.503441417683177406, -22.05068747287765873, 5.250000000000000888 ) ) ;
#11739=CARTESIAN_POINT ( 'NONE',  ( -5.121558582316795061, -22.99999999999999645, 3.550687472877652073 ) ) ;
#11741=CARTESIAN_POINT ( 'NONE',  ( 13.12519991495504712, 4.260095705229160146, 6.739971950528219402 ) ) ;
#11742=CARTESIAN_POINT ( 'NONE',  ( 13.09358652029869141, 4.163619275088517035, 5.207983256689002083 ) ) ;
#11743=CARTESIAN_POINT ( 'NONE',  ( -12.62672070884157804, -20.24999999999991473, 3.550922209436377042 ) ) ;
#11751=CARTESIAN_POINT ( 'NONE',  ( 2.702705060698113115, -10.69015907548275379, 2.777197378435510622 ) ) ;
#11752=CARTESIAN_POINT ( 'NONE',  ( 13.12500000000000178, 5.000000000000047962, 4.000000000000000000 ) ) ;
#11755=CARTESIAN_POINT ( 'NONE',  ( 13.23120918948287361, -20.54541409651599082, 3.468569357888747540 ) ) ;
#11756=CARTESIAN_POINT ( 'NONE',  ( -2.592143777221601386, -9.905122062175031772, 2.575584190728205325 ) ) ;
#11757=CARTESIAN_POINT ( 'NONE',  ( -5.121558582316794173, -23.74999999999999645, 3.550687472877651629 ) ) ;
#11758=CARTESIAN_POINT ( 'NONE',  ( -1.407845757905374695, -8.364917468222230923, 2.372643865078341019 ) ) ;
#11760=CARTESIAN_POINT ( 'NONE',  ( -13.09560264576187905, 4.265433610975056133, 3.666666666666500873 ) ) ;
#11761=CARTESIAN_POINT ( 'NONE',  ( -6.715308582316794173, -23.77099543870833998, 2.825813738724734847 ) ) ;
#11762=CARTESIAN_POINT ( 'NONE',  ( -5.878441417683177406, -23.74999999999999645, 3.449312527122335492 ) ) ;
#11764=CARTESIAN_POINT ( 'NONE',  ( 13.37499999999998579, -20.24999999999999289, 3.146526952850934755 ) ) ;
#11776=CARTESIAN_POINT ( 'NONE',  ( 0.2815691515810352930, -9.114917468222230923, 2.372643865078523984 ) ) ;
#11777=CARTESIAN_POINT ( 'NONE',  ( -7.934058582316792396, -23.20159541128345992, 4.773278322869455970 ) ) ;
#11780=CARTESIAN_POINT ( 'NONE',  ( 13.87144757537903494, 4.070602556641903291, 6.741633940066556363 ) ) ;
#11782=CARTESIAN_POINT ( 'NONE',  ( 10.19094141768317741, -22.74294823697955081, 4.171265325393542334 ) ) ;
#11783=CARTESIAN_POINT ( 'NONE',  ( -12.64195242771744709, -19.39390240027112000, 5.496549442168085164 ) ) ;
#11784=CARTESIAN_POINT ( 'NONE',  ( -7.472191417683177406, -22.97900456129165292, 3.035098964749240125 ) ) ;
#11785=CARTESIAN_POINT ( 'NONE',  ( -6.246558582316795949, -21.94931252712234127, 6.000000000000001776 ) ) ;
#11788=CARTESIAN_POINT ( 'NONE',  ( 13.10557919622060652, 4.019249409169220577, 6.007898877577752650 ) ) ;
#11789=CARTESIAN_POINT ( 'NONE',  ( -13.09546733092777160, 2.758600211853326822, 6.730829579156167419 ) ) ;
#11791=ADVANCED_FACE ( 'NONE', ( #2246 ), #2662, .T. ) ;
#11797=CARTESIAN_POINT ( 'NONE',  ( 13.29909190252318041, -20.02341932109202105, 3.459266583615586033 ) ) ;
#11799=DIRECTION ( 'NONE',  ( -0.1351665943404306014, -0.9596796555888912339, 0.2464649070825229438 ) ) ;
#11800=CARTESIAN_POINT ( 'NONE',  ( 12.69247507894198712, -16.84250851341299082, 5.559274842915185033 ) ) ;
#11801=CARTESIAN_POINT ( 'NONE',  ( -3.342893013439646843, -9.383962644129466568, 1.884355023724047173 ) ) ;
#11806=CARTESIAN_POINT ( 'NONE',  ( 13.12529397354238192, 5.014845663890295846, 4.666666666666619889 ) ) ;
#11807=CARTESIAN_POINT ( 'NONE',  ( 4.413027396565882832, -21.64511906963072363, 4.828480566969830079 ) ) ;
#11808=CARTESIAN_POINT ( 'NONE',  ( 10.09030858231679595, -21.01515356694490322, 0.9790045612916562501 ) ) ;
#11809=CARTESIAN_POINT ( 'NONE',  ( -13.15498530132288479, 5.764257716805535559, 2.999999999999999556 ) ) ;
#11810=CARTESIAN_POINT ( 'NONE',  ( -4.190941417683176518, -23.80360840875937001, 5.231925497173365081 ) ) ;
#11813=CARTESIAN_POINT ( 'NONE',  ( 9.715308582316795949, -23.02099543870833998, 3.136473910504556262 ) ) ;
#11817=CARTESIAN_POINT ( 'NONE',  ( 13.39482594849551944, -19.24878960097397140, 5.493002502378098839 ) ) ;
#11822=EDGE_CURVE ( 'NONE', #11689, #14392, #19741, .T. ) ;
#11826=CARTESIAN_POINT ( 'NONE',  ( 13.39359219590679295, -19.31109410670777038, 5.491647114909025795 ) ) ;
#11828=CARTESIAN_POINT ( 'NONE',  ( 1.932703420524435112, -8.381852853175612239, 2.376993210252662969 ) ) ;
#11831=CARTESIAN_POINT ( 'NONE',  ( 0.9854920305337621089, -9.114917468222230923, 1.622643865078341463 ) ) ;
#11832=CARTESIAN_POINT ( 'NONE',  ( -12.63238774201960268, -19.12691902800888499, 4.760115940007608515 ) ) ;
#11833=CARTESIAN_POINT ( 'NONE',  ( 6.059058582316793284, -20.72672167713054137, 4.701595411283463477 ) ) ;
#11835=CARTESIAN_POINT ( 'NONE',  ( 12.62888984277510218, -20.05356293986039873, 5.111704976569332537 ) ) ;
#11836=CARTESIAN_POINT ( 'NONE',  ( -2.567175533087980188, -9.771398394011347577, 2.541241281345096859 ) ) ;
#11837=CARTESIAN_POINT ( 'NONE',  ( 7.934058582316796837, -22.67126532539354855, 4.242948236979545484 ) ) ;
#11838=CARTESIAN_POINT ( 'NONE',  ( 7.847191417683176518, -21.22443879296941915, 1.770995438708345748 ) ) ;
#11839=CARTESIAN_POINT ( 'NONE',  ( -8.121558582316792396, -23.74999999999999645, 3.550687472877651629 ) ) ;
#11841=CARTESIAN_POINT ( 'NONE',  ( 13.15047398821051239, 5.536436404627260721, 5.896317606305554015 ) ) ;
#11842=CARTESIAN_POINT ( 'NONE',  ( 12.63958155142659834, -18.76363165295958524, 4.767928440007602298 ) ) ;
#11851=CARTESIAN_POINT ( 'NONE',  ( -3.944195004867014909, -21.61378581760806128, 5.207602947182413011 ) ) ;
#11852=CARTESIAN_POINT ( 'NONE',  ( 1.797604806073912709, -9.120796646272857799, 2.374153755450133740 ) ) ;
#11857=CARTESIAN_POINT ( 'NONE',  ( -7.559058582316794173, -20.72672167713054137, 4.701595411283463477 ) ) ;
#11858=CARTESIAN_POINT ( 'NONE',  ( -3.292205091070697698, -9.639507599131205140, 2.699984073191874057 ) ) ;
#11860=CARTESIAN_POINT ( 'NONE',  ( -13.37505992445764136, -19.49697381488866554, 4.539006848837218833 ) ) ;
#11861=CARTESIAN_POINT ( 'NONE',  ( -8.590308582316794173, -21.32581373872472597, 1.729004561291657582 ) ) ;
#11862=CARTESIAN_POINT ( 'NONE',  ( -3.944195004867016241, -21.61378581760806838, 5.207602947182413899 ) ) ;
#11864=CARTESIAN_POINT ( 'NONE',  ( 13.84983662433050178, 3.729249528687784920, 5.987138032956566214 ) ) ;
#11875=CARTESIAN_POINT ( 'NONE',  ( 5.972191417683177406, -23.72900456129164937, 2.724438792969417378 ) ) ;
#11878=CARTESIAN_POINT ( 'NONE',  ( 0.000000000000000000, -9.114917468222230923, 2.372643865078340575 ) ) ;
#11880=CARTESIAN_POINT ( 'NONE',  ( 12.62499999999998224, -20.99999999999998934, 4.166666666666637653 ) ) ;
#11882=CARTESIAN_POINT ( 'NONE',  ( 12.44094141768317741, -21.25705176302044208, 2.828734674606458555 ) ) ;
#11883=CARTESIAN_POINT ( 'NONE',  ( -12.63943061533661982, -19.52125392549825733, 5.470334935344855154 ) ) ;
#11884=CARTESIAN_POINT ( 'NONE',  ( -4.284691417683177406, -23.02099543870834353, 3.863526089495429972 ) ) ;
#11885=CARTESIAN_POINT ( 'NONE',  ( -7.378441417683177406, -24.50000000000000000, 3.449312527122335048 ) ) ;
#11887=CARTESIAN_POINT ( 'NONE',  ( 13.12529397354238192, 5.014845663890295846, 3.000000000000000000 ) ) ;
#11888=CARTESIAN_POINT ( 'NONE',  ( -13.10252221513633941, 3.864871864382954048, 6.004587342915129966 ) ) ;
#11898=CARTESIAN_POINT ( 'NONE',  ( 13.10557919622060652, 4.019249409169220577, 6.007898877577752650 ) ) ;
#11900=CARTESIAN_POINT ( 'NONE',  ( -2.844469389063872811, -10.54053385813977606, 1.988770633557972012 ) ) ;
#11906=CARTESIAN_POINT ( 'NONE',  ( 9.628441417683177406, -19.49999999999998934, 3.550687472877664952 ) ) ;
#11907=CARTESIAN_POINT ( 'NONE',  ( -12.64195242771744709, -19.39390240027112000, 5.496549442168085164 ) ) ;
#11908=CARTESIAN_POINT ( 'NONE',  ( -8.409691417683177406, -21.01515356694492098, 6.020995438708349745 ) ) ;
#11912=CARTESIAN_POINT ( 'NONE',  ( -13.86833701876684088, 3.913519447696059750, 6.741146579470268740 ) ) ;
#11913=CARTESIAN_POINT ( 'NONE',  ( 6.621558582316796837, -22.99999999999999645, 3.550687472877652073 ) ) ;
#11917=CARTESIAN_POINT ( 'NONE',  ( 13.87406079471522347, 4.952570133121557028, 5.260711232101737522 ) ) ;
#11926=CARTESIAN_POINT ( 'NONE',  ( 13.40022353639839103, -18.97621141187856608, 5.498856782956575984 ) ) ;
#11928=CARTESIAN_POINT ( 'NONE',  ( 1.619022621591187150, -9.114917468222230923, 2.372643865078341019 ) ) ;
#11930=CARTESIAN_POINT ( 'NONE',  ( -12.62868952012632207, -19.31367923361656480, 4.748088538831167327 ) ) ;
#11931=LINE ( 'NONE', #18325, #19334 ) ;
#11932=CARTESIAN_POINT ( 'NONE',  ( 11.68405858231679417, -20.79840458871652942, 2.226721677130544030 ) ) ;
#11933=CARTESIAN_POINT ( 'NONE',  ( -13.84517967659089521, 2.744073667841084418, 6.715984435864265301 ) ) ;
#11936=CARTESIAN_POINT ( 'NONE',  ( 8.590308582316797725, -21.63647391050454871, 2.479004561291657804 ) ) ;
#11937=CARTESIAN_POINT ( 'NONE',  ( 8.034691417683175629, -20.22900456129164581, 2.825813738724747726 ) ) ;
#11938=CARTESIAN_POINT ( 'NONE',  ( -12.71530858231679240, -23.77099543870833998, 2.825813738724734847 ) ) ;
#11940=CARTESIAN_POINT ( 'NONE',  ( 13.15316049959406364, 5.672105229501871904, 5.573635960501007958 ) ) ;
#11941=CARTESIAN_POINT ( 'NONE',  ( 13.06641424290328501, 2.791419266617020334, 5.231470106674447784 ) ) ;
#11952=CARTESIAN_POINT ( 'NONE',  ( 2.513306525444908512, -9.622685169956881168, 2.503048754562789746 ) ) ;
#11957=CARTESIAN_POINT ( 'NONE',  ( -2.583953725994688533, -9.847075946378776479, 2.560676788604062004 ) ) ;
#11958=CARTESIAN_POINT ( 'NONE',  ( -4.840308582316793284, -22.67418626127525982, 5.270995438708342640 ) ) ;
#11959=CARTESIAN_POINT ( 'NONE',  ( -3.564229130755586006, -10.39902496812945465, 2.145043306434553987 ) ) ;
#11960=EDGE_LOOP ( 'NONE', ( #7612, #20201, #2128, #16616, #4876 ) ) ;
#11961=CARTESIAN_POINT ( 'NONE',  ( -13.38007464613909470, -19.24373036997283037, 4.743072998953621777 ) ) ;
#11962=CARTESIAN_POINT ( 'NONE',  ( -7.465308582316795061, -20.22900456129164937, 4.174186261275266929 ) ) ;
#11963=CARTESIAN_POINT ( 'NONE',  ( 12.62155858231679417, -24.50000000000000000, 3.550687472877651629 ) ) ;
#11964=CARTESIAN_POINT ( 'NONE',  ( -11.97219141768317918, -22.97900456129165292, 3.035098964749240125 ) ) ;
#11966=CARTESIAN_POINT ( 'NONE',  ( 13.85403523778986390, 3.941279508358651817, 5.991705257707216958 ) ) ;
#11973=ADVANCED_FACE ( 'NONE', ( #4339 ), #8425, .F. ) ;
#11974=CARTESIAN_POINT ( 'NONE',  ( -13.37741471237955260, -20.12805702483293757, 4.993653275319895890 ) ) ;
#11980=CARTESIAN_POINT ( 'NONE',  ( 3.422464802389687311, -10.54865018547243061, 2.933470051312085936 ) ) ;
#11981=CARTESIAN_POINT ( 'NONE',  ( -4.840308582316793284, -22.67418626127525982, 5.270995438708342640 ) ) ;
#11984=CARTESIAN_POINT ( 'NONE',  ( 12.63178515739782348, -20.65734955141111584, 5.567013446834313761 ) ) ;
#11988=CARTESIAN_POINT ( 'NONE',  ( 5.972191417683179182, -23.72900456129165292, 2.724438792969417822 ) ) ;
#11990=CARTESIAN_POINT ( 'NONE',  ( -8.222191417683175629, -21.02099543870834353, 3.964901035250761208 ) ) ;
#11991=CARTESIAN_POINT ( 'NONE',  ( -11.78469141768317741, -24.52099543870834708, 4.484846433055073689 ) ) ;
#11993=CARTESIAN_POINT ( 'NONE',  ( 13.12529418130016445, 5.014856155665242454, 4.958178834604180629 ) ) ;
#11994=CARTESIAN_POINT ( 'NONE',  ( -12.91308523408712183, -5.701695678577235249, 5.798858176249892082 ) ) ;
#12007=CARTESIAN_POINT ( 'NONE',  ( -3.436477319925839602, -9.631595465688135960, 1.947952079262935676 ) ) ;
#12011=CARTESIAN_POINT ( 'NONE',  ( 6.527808582316795949, -24.47900456129166358, 4.586221378810390270 ) ) ;
#12012=CARTESIAN_POINT ( 'NONE',  ( -13.12529397354238192, 5.014845663890295846, 4.791666666666685614 ) ) ;
#12013=CARTESIAN_POINT ( 'NONE',  ( -8.503441417683177406, -22.05068747287766229, 6.000000000000001776 ) ) ;
#12014=CIRCLE ( 'NONE', #13035, 0.3749999999999997224 ) ;
#12018=CARTESIAN_POINT ( 'NONE',  ( -13.67732412376249052, -5.732631749971324631, 6.533692769198849781 ) ) ;
#12020=CARTESIAN_POINT ( 'NONE',  ( 11.49655858231679417, -22.05068747287764452, 1.749999999999998446 ) ) ;
#12024=CARTESIAN_POINT ( 'NONE',  ( 13.87470602645761986, 4.985154336109792972, 4.166666666666765551 ) ) ;
#12033=( GEOMETRIC_REPRESENTATION_CONTEXT ( 3 ) GLOBAL_UNCERTAINTY_ASSIGNED_CONTEXT ( ( #20539 ) ) GLOBAL_UNIT_ASSIGNED_CONTEXT ( ( #17046, #20716, #12747 ) ) REPRESENTATION_CONTEXT ( 'NONE', 'WORKASPACE' ) );
#12035=CARTESIAN_POINT ( 'NONE',  ( 1.337453470010121714, -9.114917468222230923, 2.372643865078341019 ) ) ;
#12036=AXIS2_PLACEMENT_3D ( 'NONE', #4965, #14376, #8313 ) ;
#12038=CARTESIAN_POINT ( 'NONE',  ( -13.12529397354238192, 5.014845663890295846, 4.833333333333344584 ) ) ;
#12041=CARTESIAN_POINT ( 'NONE',  ( -13.40653076352726103, -19.40769644187082932, 6.236886054669082746 ) ) ;
#12044=CARTESIAN_POINT ( 'NONE',  ( 10.93405858231679417, -23.20159541128345992, 4.773278322869455970 ) ) ;
#12045=CARTESIAN_POINT ( 'NONE',  ( 12.44094141768317741, -21.25705176302044208, 2.828734674606458555 ) ) ;
#12046=CARTESIAN_POINT ( 'NONE',  ( -11.21530858231679417, -23.77099543870833998, 2.825813738724734847 ) ) ;
#12048=CARTESIAN_POINT ( 'NONE',  ( 12.64802275499843454, -19.83735087257960927, 6.157588447769994922 ) ) ;
#12050=CARTESIAN_POINT ( 'NONE',  ( 12.63238774201960268, -19.12691902800888499, 4.760115940007608515 ) ) ;
#12060=CARTESIAN_POINT ( 'NONE',  ( -12.62515553039088090, -20.24214571525854467, 4.629702272822510345 ) ) ;
#12063=CARTESIAN_POINT ( 'NONE',  ( 0.5631383031621635116, -9.864917468222230923, 2.372643865078341019 ) ) ;
#12069=CARTESIAN_POINT ( 'NONE',  ( -9.902808582316795949, -23.08622137881038938, 1.020995438708339309 ) ) ;
#12070=CARTESIAN_POINT ( 'NONE',  ( -2.787023586469211001, -10.13267000451481614, 1.884023048047904103 ) ) ;
#12072=CARTESIAN_POINT ( 'NONE',  ( -13.76337198624852398, 0.1127853055781036368, 5.159333296715827188 ) ) ;
#12073=CARTESIAN_POINT ( 'NONE',  ( -7.090308582316794173, -21.32581373872472597, 1.729004561291657582 ) ) ;
#12074=CARTESIAN_POINT ( 'NONE',  ( 11.97219141768317918, -24.47900456129165292, 2.413778621189595963 ) ) ;
#12075=CARTESIAN_POINT ( 'NONE',  ( -10.84719141768317741, -21.53509896474923835, 2.520995438708346192 ) ) ;
#12077=CARTESIAN_POINT ( 'NONE',  ( 13.81626551376501588, 2.033908445126689557, 5.950679699622869911 ) ) ;
#12079=ORIENTED_EDGE ( 'NONE', *, *, #10896, .T. ) ;
#12083=CARTESIAN_POINT ( 'NONE',  ( -13.83065313257865370, 2.760483195222930952, 5.966304699623404595 ) ) ;
#12090=CARTESIAN_POINT ( 'NONE',  ( 3.292205091070697698, -9.639507599131205140, 2.699984073191874057 ) ) ;
#12093=CARTESIAN_POINT ( 'NONE',  ( 13.90258797164900884, 5.643192568275169130, 5.568788873356017355 ) ) ;
#12098=CARTESIAN_POINT ( 'NONE',  ( 9.909691417683175629, -21.63647391050456648, 4.520995438708348857 ) ) ;
#12100=CARTESIAN_POINT ( 'NONE',  ( -3.944195004867014909, -21.80034658733847053, 4.481176709221804444 ) ) ;
#12102=CARTESIAN_POINT ( 'NONE',  ( -11.59719141768317741, -23.08622137881040359, 5.979004561291654696 ) ) ;
#12104=CARTESIAN_POINT ( 'NONE',  ( 12.72590726430969532, -14.40418315237199742, 4.861678440007700885 ) ) ;
#12105=CARTESIAN_POINT ( 'NONE',  ( -12.64691428603184242, -19.14332855539073464, 5.509795676248469221 ) ) ;
#12112=ORIENTED_EDGE ( 'NONE', *, *, #19216, .F. ) ;
#12116=CARTESIAN_POINT ( 'NONE',  ( -2.012076196476103362, -9.160103213191565175, 1.634248467062433541 ) ) ;
#12120=CARTESIAN_POINT ( 'NONE',  ( 9.722191417683177406, -19.52099543870834353, 4.586221378810406257 ) ) ;
#12121=CARTESIAN_POINT ( 'NONE',  ( -13.10192273101908000, 3.834597916462216816, 6.003936301248457674 ) ) ;
#12122=CARTESIAN_POINT ( 'NONE',  ( -6.253441417683175629, -21.94931252712233061, 0.9999999999999978906 ) ) ;
#12124=CARTESIAN_POINT ( 'NONE',  ( 13.18405858231679417, -20.79840458871652942, 2.226721677130544030 ) ) ;
#12126=CARTESIAN_POINT ( 'NONE',  ( -13.86676110481170632, 3.833935792988865110, 6.739421935864088553 ) ) ;
#12128=CARTESIAN_POINT ( 'NONE',  ( 10.18405858231679417, -20.79840458871652942, 2.226721677130544030 ) ) ;
#12129=CARTESIAN_POINT ( 'NONE',  ( -3.944195004867014909, -21.61378581760806128, 5.207602947182413011 ) ) ;
#12132=CARTESIAN_POINT ( 'NONE',  ( 13.38795836133016870, -20.34560275282643005, 5.879540349057044146 ) ) ;
#12138=CARTESIAN_POINT ( 'NONE',  ( -9.621558582316794173, -23.74999999999999645, 3.550687472877651629 ) ) ;
#12142=CARTESIAN_POINT ( 'NONE',  ( 2.801385037117921861, -10.23463596792102415, 1.910209944425432349 ) ) ;
#12144=CARTESIAN_POINT ( 'NONE',  ( -13.37499999999998401, -19.49999999999998934, 3.146526952850934755 ) ) ;
#12146=CARTESIAN_POINT ( 'NONE',  ( -13.86833701876684088, 3.913519447696059750, 6.741146579470268740 ) ) ;
#12148=CARTESIAN_POINT ( 'NONE',  ( 5.777808582316795949, -21.02099543870833998, 3.035098964749253003 ) ) ;
#12149=CARTESIAN_POINT ( 'NONE',  ( 10.75344141768317741, -21.94931252712233061, 2.499999999999999112 ) ) ;
#12150=CARTESIAN_POINT ( 'NONE',  ( -9.059058582316794173, -20.72672167713054137, 4.701595411283463477 ) ) ;
#12152=CARTESIAN_POINT ( 'NONE',  ( 12.62506359033936754, -19.49678868786235597, 4.541393094775662220 ) ) ;
#12159=CARTESIAN_POINT ( 'NONE',  ( -12.62499999999998224, -20.24999999999998934, 4.166666666666636765 ) ) ;
#12161=CARTESIAN_POINT ( 'NONE',  ( -13.85528666703740619, 4.004476685417483139, 5.993048563355776182 ) ) ;
#12168=CARTESIAN_POINT ( 'NONE',  ( -0.9854920305337621089, -9.114917468222230923, 2.372643865078341019 ) ) ;
#12169=CARTESIAN_POINT ( 'NONE',  ( -8.871558582316795949, -19.49999999999998934, 3.449312527122348371 ) ) ;
#12170=CARTESIAN_POINT ( 'NONE',  ( -1.619022621591186928, -8.364917468222230923, 1.622643865078341907 ) ) ;
#12172=CARTESIAN_POINT ( 'NONE',  ( -13.42766088059286922, -16.84062553004338625, 4.794749963382423985 ) ) ;
#12174=CARTESIAN_POINT ( 'NONE',  ( 11.40969141768317918, -21.01515356694492098, 6.020995438708349745 ) ) ;
#12175=CARTESIAN_POINT ( 'NONE',  ( -9.815941417683177406, -21.32873467460645145, 4.242948236979555254 ) ) ;
#12177=CARTESIAN_POINT ( 'NONE',  ( 13.66279757975024722, -5.716222222589476765, 5.784013032957989964 ) ) ;
#12183=CARTESIAN_POINT ( 'NONE',  ( -13.87470623115321899, 4.985164673244912414, 4.958488177337359026 ) ) ;
#12185=CARTESIAN_POINT ( 'NONE',  ( 2.513306525444908512, -9.622685169956881168, 2.503048754562789746 ) ) ;
#12189=CARTESIAN_POINT ( 'NONE',  ( 3.722205087890566144, -11.52065056559861134, 2.433099166587254558 ) ) ;
#12191=CARTESIAN_POINT ( 'NONE',  ( 13.09546733092777160, 2.758600211853326822, 6.730829579156167419 ) ) ;
#12192=CARTESIAN_POINT ( 'NONE',  ( 3.944195004867014909, -21.61378581760806128, 5.207602947182413011 ) ) ;
#12197=CARTESIAN_POINT ( 'NONE',  ( 10.75344141768317741, -21.94931252712233061, 2.499999999999999112 ) ) ;
#12199=CARTESIAN_POINT ( 'NONE',  ( -9.434058582316795949, -22.67126532539354855, 4.242948236979545484 ) ) ;
#12200=CARTESIAN_POINT ( 'NONE',  ( -9.065941417683177406, -23.73192549717336064, 1.696391591240623331 ) ) ;
#12202=CARTESIAN_POINT ( 'NONE',  ( 12.62499994688180749, -19.50000268246798640, 4.473800639250938183 ) ) ;
#12203=CARTESIAN_POINT ( 'NONE',  ( -13.10431844137356627, 3.955581289335645234, 6.006545679920360925 ) ) ;
#12208=CARTESIAN_POINT ( 'NONE',  ( 1.700193846275138032, -9.865151716929458914, 2.372704024825938340 ) ) ;
#12216=CARTESIAN_POINT ( 'NONE',  ( -1.619022621591186928, -9.864917468222230923, 1.622643865078341907 ) ) ;
#12220=CARTESIAN_POINT ( 'NONE',  ( 11.12844141768317741, -19.49999999999998934, 3.550687472877664952 ) ) ;
#12221=CARTESIAN_POINT ( 'NONE',  ( -12.74043380832193684, -14.42059267975384529, 5.611358176248560703 ) ) ;
#12222=EDGE_CURVE ( 'NONE', #10614, #8228, #3036, .T. ) ;
#12223=CARTESIAN_POINT ( 'NONE',  ( -11.22219141768317741, -20.27099543870833998, 4.275561207030583510 ) ) ;
#12225=CARTESIAN_POINT ( 'NONE',  ( 11.68405858231679417, -20.79840458871652942, 2.226721677130544030 ) ) ;
#12227=CARTESIAN_POINT ( 'NONE',  ( -13.39169349927020569, -20.15697828685464188, 6.009339318877812808 ) ) ;
#12228=CARTESIAN_POINT ( 'NONE',  ( 10.84030858231679240, -22.67418626127525982, 5.270995438708342640 ) ) ;
#12232=CARTESIAN_POINT ( 'NONE',  ( 13.37499964066394043, -21.00001814646822496, 4.442866346476199269 ) ) ;
#12237=CARTESIAN_POINT ( 'NONE',  ( -8.496558582316794173, -22.05068747287764452, 1.749999999999998446 ) ) ;
#12239=CYLINDRICAL_SURFACE ( 'NONE', #2177, 0.3749999999999997224 ) ;
#12240=CARTESIAN_POINT ( 'NONE',  ( 1.798207051321043304, -8.367281747657623114, 1.623251059268568053 ) ) ;
#12243=CARTESIAN_POINT ( 'NONE',  ( -13.37499999999998224, -19.49999999999998934, 4.291666666666699825 ) ) ;
#12244=CARTESIAN_POINT ( 'NONE',  ( 13.09030858231679417, -21.32581373872472597, 1.729004561291657582 ) ) ;
#12245=CARTESIAN_POINT ( 'NONE',  ( -13.37500000000002132, -20.99999999999450395, 3.833333333368183382 ) ) ;
#12246=ADVANCED_FACE ( 'NONE', ( #11245 ), #20473, .F. ) ;
#12248=CARTESIAN_POINT ( 'NONE',  ( 12.24655858231679240, -21.94931252712234482, 5.250000000000000888 ) ) ;
#12249=CARTESIAN_POINT ( 'NONE',  ( 5.690941417683176518, -23.27327832286946219, 4.701595411283453707 ) ) ;
#12250=CARTESIAN_POINT ( 'NONE',  ( -6.246558582316794173, -21.94931252712234482, 5.250000000000000888 ) ) ;
#12252=CARTESIAN_POINT ( 'NONE',  ( 13.37499999999998401, -19.49999999999998934, 2.439580858552613751 ) ) ;
#12257=PRODUCT_DEFINITION ( 'UNKNOWN', '', #17378, #3161 ) ;
#12258=CARTESIAN_POINT ( 'NONE',  ( -13.09532840572934376, 3.501584489333809724, 5.996774842915142401 ) ) ;
#12260=CARTESIAN_POINT ( 'NONE',  ( -13.38800411018677572, -19.59329243556743805, 5.436267741224407146 ) ) ;
#12265=CARTESIAN_POINT ( 'NONE',  ( 4.687312169500630787, -21.51559725698340131, 5.182386163300424009 ) ) ;
#12266=CARTESIAN_POINT ( 'NONE',  ( -8.309058582316795949, -23.80360840875935935, 1.768074502826626260 ) ) ;
#12267=CARTESIAN_POINT ( 'NONE',  ( -1.852280067228949445, -9.126254559850970338, 1.625555456689752321 ) ) ;
#12269=CARTESIAN_POINT ( 'NONE',  ( -13.37741471237955260, -20.12805702483293757, 4.993653275319895890 ) ) ;
#12272=APPLICATION_CONTEXT ( 'automotive_design' ) ;
#12273=CARTESIAN_POINT ( 'NONE',  ( 12.62844141768317741, -19.49999999999998934, 3.550687472877664952 ) ) ;
#12274=CARTESIAN_POINT ( 'NONE',  ( -9.440941417683177406, -21.25705176302044208, 2.828734674606458555 ) ) ;
#12276=CARTESIAN_POINT ( 'NONE',  ( 13.86106797245302147, 4.296432608878145487, 5.947261916831099171 ) ) ;
#12277=CARTESIAN_POINT ( 'NONE',  ( 12.62515553039088090, -20.24214571525854467, 4.629702272822510345 ) ) ;
#12282=CARTESIAN_POINT ( 'NONE',  ( -13.87470602645761808, 4.985154336109792972, 4.000000000000000000 ) ) ;
#12290=CARTESIAN_POINT ( 'NONE',  ( 2.708677329869237482, -9.785633270066144362, 1.794897081886200230 ) ) ;
#12292=CARTESIAN_POINT ( 'NONE',  ( 13.12526104302547836, 5.013182672784613381, 5.066812735559260261 ) ) ;
#12296=CARTESIAN_POINT ( 'NONE',  ( 8.878441417683177406, -22.99999999999999645, 3.449312527122335048 ) ) ;
#12297=CARTESIAN_POINT ( 'NONE',  ( -13.11145189917479392, 4.315820908324673688, 5.961432613039677086 ) ) ;
#12298=CARTESIAN_POINT ( 'NONE',  ( -7.371558582316795949, -20.99999999999999645, 3.449312527122348371 ) ) ;
#12300=CARTESIAN_POINT ( 'NONE',  ( -11.40969141768317918, -21.01515356694492098, 6.020995438708349745 ) ) ;
#12303=CARTESIAN_POINT ( 'NONE',  ( 12.62966097655984754, -19.26462068372267566, 4.756751955311774083 ) ) ;
#12304=CARTESIAN_POINT ( 'NONE',  ( -13.11740841389447709, 4.616624901677048420, 5.813473370769506765 ) ) ;
#12308=CARTESIAN_POINT ( 'NONE',  ( 1.791727654783324741, -9.894249715907907472, 2.380176972254574697 ) ) ;
#12315=CARTESIAN_POINT ( 'NONE',  ( -1.744064896197293324, -9.868721669903177229, 1.623620860066563365 ) ) ;
#12319=CARTESIAN_POINT ( 'NONE',  ( 5.409691417683178294, -21.01515356694492098, 6.020995438708349745 ) ) ;
#12320=CARTESIAN_POINT ( 'NONE',  ( -12.64691428603184242, -19.14332855539073464, 5.509795676248469221 ) ) ;
#12321=CARTESIAN_POINT ( 'NONE',  ( -11.40969141768318096, -21.32581373872474373, 5.270995438708348857 ) ) ;
#12325=CARTESIAN_POINT ( 'NONE',  ( 12.99655858231679417, -22.05068747287764452, 1.749999999999998446 ) ) ;
#12327=CARTESIAN_POINT ( 'NONE',  ( -13.37499999999998224, -20.99999999999998934, 4.291666666666699825 ) ) ;
#12329=CARTESIAN_POINT ( 'NONE',  ( 6.152808582316795949, -21.53509896474924901, 4.479004561291659137 ) ) ;
#12334=CARTESIAN_POINT ( 'NONE',  ( 13.38172782443493602, -20.66024486603417643, 5.557997437521964734 ) ) ;
#12342=CARTESIAN_POINT ( 'NONE',  ( -12.52780858231679595, -23.72900456129165647, 4.275561207030568411 ) ) ;
#12345=CARTESIAN_POINT ( 'NONE',  ( 1.852280067228949445, -9.126254559850970338, 1.625555456689752321 ) ) ;
#12348=CARTESIAN_POINT ( 'NONE',  ( -13.37908441539295801, -19.29373702265862889, 4.740102594697787275 ) ) ;
#12349=CARTESIAN_POINT ( 'NONE',  ( 13.37155858231679417, -20.24999999999999289, 3.449312527122348371 ) ) ;
#12350=CARTESIAN_POINT ( 'NONE',  ( -13.37526900345969771, -20.98641532528209908, 4.724331462949078464 ) ) ;
#12355=CARTESIAN_POINT ( 'NONE',  ( 6.340308582316796837, -22.36352608949544418, 4.520995438708343528 ) ) ;
#12356=CARTESIAN_POINT ( 'NONE',  ( 9.722191417683177406, -21.02099543870834353, 3.964901035250761208 ) ) ;
#12357=CARTESIAN_POINT ( 'NONE',  ( -11.31594141768317741, -20.79840458871654363, 4.773278322869464851 ) ) ;
#12359=CARTESIAN_POINT ( 'NONE',  ( 13.37500751150753864, -19.49962066887028556, 4.515663405036051792 ) ) ;
#12367=CARTESIAN_POINT ( 'NONE',  ( -12.62672070884157804, -20.24999999999991473, 3.550922209436377042 ) ) ;
#12368=CARTESIAN_POINT ( 'NONE',  ( -1.957016269584227031, -9.152392576945766578, 2.382268221639079364 ) ) ;
#12369=CARTESIAN_POINT ( 'NONE',  ( -13.87470602645761986, 4.985154336109792972, 4.916666666666650087 ) ) ;
#12371=CARTESIAN_POINT ( 'NONE',  ( -12.62499999998404121, -20.24999999996810729, 2.793053905886972998 ) ) ;
#12376=CARTESIAN_POINT ( 'NONE',  ( -13.09030858231679417, -21.01515356694490322, 0.9790045612916562501 ) ) ;
#12377=CARTESIAN_POINT ( 'NONE',  ( -2.282685604506861754, -11.80366834561962364, 2.120553820834011116 ) ) ;
#12379=CARTESIAN_POINT ( 'NONE',  ( -13.37500000000002132, -20.24999999999450040, 3.833333333368183382 ) ) ;
#12380=AXIS2_PLACEMENT_3D ( 'NONE', #10412, #7174, #2350 ) ;
#12383=CARTESIAN_POINT ( 'NONE',  ( 6.152808582316795949, -20.91377862118960351, 5.979004561291660913 ) ) ;
#12384=CARTESIAN_POINT ( 'NONE',  ( -5.972191417683178294, -22.97900456129165292, 3.035098964749240125 ) ) ;
#12386=CARTESIAN_POINT ( 'NONE',  ( 13.37499999999998401, -20.99999999999999645, 3.146526952850934755 ) ) ;
#12391=CARTESIAN_POINT ( 'NONE',  ( -13.66279757975024722, -5.716222222589476765, 5.784013032957989964 ) ) ;
#12395=CARTESIAN_POINT ( 'NONE',  ( 2.817596665886821672, -11.50588678273290988, 2.986692549455723267 ) ) ;
#12400=CARTESIAN_POINT ( 'NONE',  ( 0.5631383031621635116, -8.364917468222230923, 1.622643865078341907 ) ) ;
#12406=CARTESIAN_POINT ( 'NONE',  ( 12.99655858231679595, -22.05068747287764452, 2.499999999999999112 ) ) ;
#12407=CARTESIAN_POINT ( 'NONE',  ( -13.12529397354238192, 5.014845663890295846, 3.666666666666500873 ) ) ;
#12408=CARTESIAN_POINT ( 'NONE',  ( -7.746558582316795949, -21.94931252712234127, 4.499999999999999112 ) ) ;
#12409=CARTESIAN_POINT ( 'NONE',  ( -4.847191417683177406, -20.91377862118959285, 1.020995438708345082 ) ) ;
#12411=CARTESIAN_POINT ( 'NONE',  ( 13.37514942709654164, -19.49245393162283690, 4.562067678168288509 ) ) ;
#12417=CARTESIAN_POINT ( 'NONE',  ( 1.862510824048270619, -9.990417728039201251, 2.404874838918925395 ) ) ;
#12421=ADVANCED_FACE ( 'NONE', ( #13603 ), #4412, .T. ) ;
#12422=CARTESIAN_POINT ( 'NONE',  ( -1.982945319006538032, -10.83166796549307520, 2.620924705558935308 ) ) ;
#12429=CARTESIAN_POINT ( 'NONE',  ( 4.003441417683175629, -22.05068747287766229, 6.000000000000001776 ) ) ;
#12430=CARTESIAN_POINT ( 'NONE',  ( -9.440941417683177406, -20.72672167713052715, 2.298404588716546293 ) ) ;
#12431=ORIENTED_EDGE ( 'NONE', *, *, #12582, .F. ) ;
#12432=CARTESIAN_POINT ( 'NONE',  ( 8.684058582316794173, -20.79840458871652942, 2.226721677130544030 ) ) ;
#12434=CARTESIAN_POINT ( 'NONE',  ( -12.62672826945118665, -20.91272239271162903, 5.058631648758789900 ) ) ;
#12440=CARTESIAN_POINT ( 'NONE',  ( 13.77324158252158171, -0.8888000826463379189, 6.637859435864801760 ) ) ;
#12447=CARTESIAN_POINT ( 'NONE',  ( -12.71530858231679240, -23.77099543870833998, 2.825813738724734847 ) ) ;
#12450=FACE_OUTER_BOUND ( 'NONE', #16455, .T. ) ;
#12451=CARTESIAN_POINT ( 'NONE',  ( 2.708677329869237482, -9.785633270066144362, 1.794897081886200230 ) ) ;
#12453=CARTESIAN_POINT ( 'NONE',  ( -13.07840392524817474, 3.396898225032857432, 5.244490940007585422 ) ) ;
#12454=CARTESIAN_POINT ( 'NONE',  ( 9.902808582316794173, -22.77556120703056308, 1.770995438708339975 ) ) ;
#12455=CARTESIAN_POINT ( 'NONE',  ( -12.65346245025441263, -19.56264626215117275, 6.228892365149262922 ) ) ;
#12458=CARTESIAN_POINT ( 'NONE',  ( 12.62155858231679417, -23.74999999999999645, 3.550687472877651629 ) ) ;
#12460=CARTESIAN_POINT ( 'NONE',  ( 9.253441417683177406, -21.94931252712233061, 2.499999999999999112 ) ) ;
#12461=CARTESIAN_POINT ( 'NONE',  ( -4.746558582316793284, -21.94931252712234482, 5.250000000000000888 ) ) ;
#12463=CARTESIAN_POINT ( 'NONE',  ( 13.38449802415168932, -19.02034978033825396, 4.747874963382372471 ) ) ;
#12464=CARTESIAN_POINT ( 'NONE',  ( -2.739050625766161762, -9.875938058683834342, 1.818089155622620412 ) ) ;
#12468=CARTESIAN_POINT ( 'NONE',  ( -13.10192273101908000, 3.834597916462216816, 6.003936301248457674 ) ) ;
#12471=CARTESIAN_POINT ( 'NONE',  ( -4.181771508648414404, -14.78356139460145968, 3.271079850667843125 ) ) ;
#12472=CARTESIAN_POINT ( 'NONE',  ( -13.85788212999909419, 4.135547564954428879, 5.982801014393342776 ) ) ;
#12473=EDGE_CURVE ( 'NONE', #18369, #8256, #4687, .T. ) ;
#12479=CARTESIAN_POINT ( 'NONE',  ( -10.09030858231679595, -21.01515356694490322, 0.9790045612916562501 ) ) ;
#12480=CARTESIAN_POINT ( 'NONE',  ( -1.865667289525601680, -9.999006358835732300, 2.407080570882605297 ) ) ;
#12482=CARTESIAN_POINT ( 'NONE',  ( -13.84501469867711698, 4.235742283194553259, 4.666666666666618113 ) ) ;
#12485=CARTESIAN_POINT ( 'NONE',  ( 6.527808582316795949, -24.47900456129166358, 4.586221378810390270 ) ) ;
#12486=CARTESIAN_POINT ( 'NONE',  ( -6.722191417683176518, -21.02099543870834353, 3.964901035250761208 ) ) ;
#12488=CARTESIAN_POINT ( 'NONE',  ( 13.41175265982446696, -19.14399067886409256, 6.245281310864100988 ) ) ;
#12489=CARTESIAN_POINT ( 'NONE',  ( 12.62500016093973620, -20.24999187254239175, 4.532396751752561848 ) ) ;
#12493=ORIENTED_EDGE ( 'NONE', *, *, #2951, .T. ) ;
#12494=CARTESIAN_POINT ( 'NONE',  ( -13.87444723674697755, 4.972085455720938185, 5.163895512850782410 ) ) ;
#12495=CARTESIAN_POINT ( 'NONE',  ( 0.9854920305337621089, -9.114917468222230923, 2.372643865078341019 ) ) ;
#12498=CARTESIAN_POINT ( 'NONE',  ( 2.623717082130370137, -10.12934627674766830, 2.633169448359191644 ) ) ;
#12500=CARTESIAN_POINT ( 'NONE',  ( 1.754777266914451461, -9.116337928146160507, 1.623008667563337726 ) ) ;
#12502=CARTESIAN_POINT ( 'NONE',  ( 13.12503131243110843, 5.001581277770153378, 5.166347330538456184 ) ) ;
#12506=CARTESIAN_POINT ( 'NONE',  ( 6.534691417683177406, -20.97900456129164581, 3.136473910504570917 ) ) ;
#12507=CARTESIAN_POINT ( 'NONE',  ( -13.10431844137356627, 3.955581289335645234, 6.006545679920360925 ) ) ;
#12508=CARTESIAN_POINT ( 'NONE',  ( -10.55905858231679595, -21.25705176302045274, 4.171265325393551215 ) ) ;
#12510=CARTESIAN_POINT ( 'NONE',  ( -4.190941417683176518, -23.80360840875937001, 5.231925497173365081 ) ) ;
#12512=CARTESIAN_POINT ( 'NONE',  ( 13.09559422631463654, 4.265008428887424152, 5.017082219073495608 ) ) ;
#12517=CARTESIAN_POINT ( 'NONE',  ( 1.668644041176298387, -9.864915931696323526, 2.372643470467795890 ) ) ;
#12519=EDGE_LOOP ( 'NONE', ( #6162, #7558, #13517, #19245, #916 ) ) ;
#12523=CARTESIAN_POINT ( 'NONE',  ( -0.5631383031621635116, -9.114917468222230923, 1.622643865078341463 ) ) ;
#12526=CARTESIAN_POINT ( 'NONE',  ( 8.972191417683177406, -24.47900456129165292, 2.413778621189595963 ) ) ;
#12527=CARTESIAN_POINT ( 'NONE',  ( 13.50000000000000178, 5.000000000000047962, 2.000000000000000000 ) ) ;
#12528=CARTESIAN_POINT ( 'NONE',  ( -9.722191417683177406, -20.27099543870833998, 4.275561207030583510 ) ) ;
#12530=CARTESIAN_POINT ( 'NONE',  ( 13.18405858231679595, -20.26807450282662160, 1.696391591240633101 ) ) ;
#12532=CARTESIAN_POINT ( 'NONE',  ( -12.92761177809936513, -5.718105205959081339, 6.548537912490751900 ) ) ;
#12534=CARTESIAN_POINT ( 'NONE',  ( 4.934058582316793284, -23.20159541128345992, 4.773278322869455970 ) ) ;
#12543=CARTESIAN_POINT ( 'NONE',  ( -13.37155858231679417, -20.24999999999999289, 3.449312527122348371 ) ) ;
#12546=CARTESIAN_POINT ( 'NONE',  ( 2.916276642307554123, -11.05036367517186058, 2.119705115445599475 ) ) ;
#12548=CARTESIAN_POINT ( 'NONE',  ( -13.37732542738919328, -19.38256591684242025, 4.710253041318374301 ) ) ;
#12549=CARTESIAN_POINT ( 'NONE',  ( 9.809058582316794173, -23.27327832286945153, 2.298404588716537411 ) ) ;
#12550=CARTESIAN_POINT ( 'NONE',  ( -12.62500000000002132, -20.99999999999450395, 3.833333333368183382 ) ) ;
#12552=CARTESIAN_POINT ( 'NONE',  ( 6.996558582316793284, -22.05068747287764452, 1.749999999999998446 ) ) ;
#12554=CARTESIAN_POINT ( 'NONE',  ( 5.878441417683177406, -22.99999999999999645, 3.449312527122335048 ) ) ;
#12555=CARTESIAN_POINT ( 'NONE',  ( -4.717959273841178636, -21.72818306014730183, 5.243595146365860771 ) ) ;
#12557=CARTESIAN_POINT ( 'NONE',  ( 13.09560264576187905, 4.265433610975056133, 4.791666666666684726 ) ) ;
#12558=CARTESIAN_POINT ( 'NONE',  ( -1.407845757905374695, -9.114917468222230923, 1.622643865078341463 ) ) ;
#12561=( BOUNDED_SURFACE ( )  B_SPLINE_SURFACE ( 3, 3, ( 
 ( #5511, #4150, #5613, #18387, #10217, #18588, #5409, #8651, #15231, #4050, #10433, #17008, #905, #10631, #7404, #1013, #5728, #18489, #15023, #10533, #2685, #16902, #11883, #9071, #11783, #3937, #18175, #16585, #2262, #10325, #6138, #2893, #18801, #10744, #19114, #17426, #17114, #7505, #13868, #7811, #17313, #4562, #20678, #1430, #9574, #10852, #14271, #2796, #10947, #20267, #2998, #7706, #1127, #6341, #17215, #18694, #9374, #4360, #12507, #3102, #6035, #4467, #14173, #5926, #12297, #11053, #15545, #9170, #12712, #9479, #1330, #4767, #1225, #7600, #11152, #9269, #12603, #17522, #20580, #15849, #13967, #1528, #20372, #12407, #3203, #15748 ),
 ( #15641, #14074, #20482, #18905, #6233, #19006, #4662, #7907, #16267, #8121, #375, #5177, #2046, #11247, #477, #11350, #11556, #4868, #1837, #8319, #14382, #260, #8009, #18045, #8222, #1935, #19524, #17936, #12912, #1629, #9680, #3605, #17841, #6651, #6851, #9986, #14798, #14585, #13222, #16367, #13021, #8431, #9886, #19619, #5277, #3717, #16066, #14693, #11653, #6758, #3298, #19424, #17626, #13127, #165, #15947, #65, #6451, #5081, #12815, #19214, #11457, #17741, #1739, #14488, #3405, #6548, #19315, #3506, #4971, #9787, #16173, #2239, #15206, #20036, #573, #15105, #18560, #18358, #16777, #10295, #8934, #14895, #11760, #8627, #8737 ),
 ( #5698, #7168, #16564, #2446, #782, #13531, #678, #985, #10095, #5487, #5590, #10406, #15305, #18151, #11860, #10194, #882, #2343, #2547, #19834, #14997, #20141, #16470, #19933, #8838, #7267, #7373, #11961, #2143, #13737, #13325, #5801, #7065, #3915, #13428, #13627, #6953, #16667, #12172, #10506, #3816, #4021, #18253, #8525, #19724, #5385, #12072, #18462, #4125, #16876, #1501, #6112, #15824, #4633, #20556, #4536, #2866, #5899, #13938, #17394, #18875, #9144, #14045, #6308, #15514, #16978, #1404, #20455, #3077, #9243, #6004, #1198, #13838, #7882, #6207, #20241, #10605, #2655, #10921, #12482, #7676, #9452, #17285, #12682, #20340, #14242 ),
 ( #2968, #10824, #4224, #20649, #12379, #1097, #9344, #7477, #15613, #12576, #7575, #18774, #15721, #9042, #15414, #14149, #18663, #12269, #4332, #18977, #4439, #10714, #17088, #2766, #17188, #1296, #7786, #11026, #19396, #14667, #4843, #347, #1599, #7978, #15054, #8196, #14562, #3483, #5054, #8098, #1811, #11431, #6525, #3578, #236, #16612, #737, #6624, #9858, #8683, #17816, #15922, #8293, #17911, #19500, #6424, #14461, #19292, #3380, #12994, #7120, #14352, #1712, #37, #6732, #16243, #1911, #19083, #13099, #11224, #12787, #5153, #11532, #19189, #4944, #17600, #9959, #4740, #3273, #2291, #11324, #17711, #9651, #11126, #17496, #16036 ),
 ( #3176, #141, #9550, #12888, #9761, #16146, #17038, #12327, #20093, #18723, #7529, #10561, #20295, #7431, #5952, #4392, #15569, #7219, #5857, #17142, #12227, #836, #5756, #2401, #18617, #18415, #1252, #2717, #4279, #2603, #2821, #13485, #18518, #8891, #19983, #10773, #935, #5644, #8792, #1047, #8992, #19886, #13792, #12018, #10663, #9097, #3966, #4179, #5542, #20197, #15469, #13682, #9194, #18302, #15160, #4077, #12126, #10354, #11912, #13581, #1152, #16931, #10463, #13893, #15364, #16728, #16832, #2496, #15258, #7321, #3130, #7930, #12840, #9297, #3028, #7739, #12741, #20605, #94, #17345, #14102, #17654, #7627, #6257, #20709, #19144 ),
 ( #11273, #10877, #19244, #6165, #1457, #18930, #6371, #18829, #7836, #4894, #8044, #1356, #4691, #9405, #3327, #20403, #12434, #15777, #13994, #9599, #14410, #9709, #6480, #2920, #16096, #14198, #3228, #17241, #12631, #4797, #6066, #19036, #4491, #15672, #11081, #14297, #11178, #17552, #4587, #20511, #17452, #15977, #9504, #12532, #15877, #10975, #1552, #1659, #6880, #11789, #14826, #19344, #11680, #601, #2169, #9814, #11488, #1966, #6784, #11584, #10222, #4999, #5108, #11378, #18078, #16396, #8458, #1765, #5206, #14613, #16200, #10125, #500, #17768, #8349, #3436, #14923, #8152, #291, #19647, #14724, #402, #1865, #6987, #14515, #8247 ),
 ( #18180, #3635, #13356, #8553, #3745, #2074, #13154, #6681, #17867, #19756, #13249, #13050, #17964, #3842, #19451, #192, #5306, #10017, #5416, #19551, #3537, #9913, #16294, #6575, #16497, #12940, #2267, #8656, #2579, #12105, #20069, #15448, #16908, #4366, #5620, #9077, #5516, #5734, #15028, #18494, #2476, #16590, #1132, #11994, #13460, #4156, #19864, #7296, #18593, #813, #13559, #8964, #709, #7095, #5834, #10330, #11888, #7510, #12203, #16808, #13873, #16699, #2377, #5931, #19960, #7409, #12304, #15338, #4257, #8767, #10638, #18280, #3943, #18700, #10538, #1019, #13771, #20174, #18392, #4055, #15138, #7197, #10439, #8868, #17013, #2690 ) ),
 .UNSPECIFIED., .T., .F., .F. ) 
 B_SPLINE_SURFACE_WITH_KNOTS ( ( 4, 3, 4 ),
 ( 4, 2, 2, 2, 2, 2, 2, 2, 2, 2, 2, 2, 2, 2, 2, 2, 2, 2, 2, 2, 2, 2, 2, 2, 2, 2, 2, 2, 2, 2, 2, 2, 2, 2, 2, 2, 2, 2, 2, 2, 2, 2, 4 ),
 ( 0.000000000000000000, 0.5000000000000000000, 1.000000000000000000 ),
 ( 0.000000000000000000, 0.03481082764294501225, 0.05122453910963481460, 0.05943139484297971231, 0.06353482270965216117, 0.06763825057632461002, 0.07081696859385246123, 0.07399568661138031245, 0.08035312264643601488, 0.09306799471654741973, 0.1057828667866588246, 0.1121403028217145270, 0.1153190208392423644, 0.1184977388567702156, 0.1214804596100246270, 0.1244631803632790246, 0.1304286218697878197, 0.1423595048828054099, 0.1662212709088405904, 0.2139448029609109514, 0.3093918670650516733, 0.5002859952733331728, 0.6911801234816146167, 0.7866271875857553386, 0.8343507196378256996, 0.8582124856638608801, 0.8701433686768784703, 0.8761088101833873765, 0.8790915309366418295, 0.8820742516898961716, 0.8853411830926052328, 0.8886081144953141830, 0.8951419773007323055, 0.9082097029115685505, 0.9212774285224047954, 0.9278112913278229179, 0.9310782227305318681, 0.9343451541332409294, 0.9384485819999133227, 0.9425520098665858271, 0.9507588655999306138, 0.9671725770666204092, 1.000000000000000000 ),
 .UNSPECIFIED. ) 
 GEOMETRIC_REPRESENTATION_ITEM ( )  RATIONAL_B_SPLINE_SURFACE ( (
 ( 1.000000000000000000, 1.000000000000000000, 1.000000000000000000, 1.000000000000000000, 1.000000000000000000, 1.000000000000000000, 1.000000000000000000, 1.000000000000000000, 1.000000000000000000, 1.000000000000000000, 1.000000000000000000, 1.000000000000000000, 1.000000000000000000, 1.000000000000000000, 1.000000000000000000, 1.000000000000000000, 1.000000000000000000, 1.000000000000000000, 1.000000000000000000, 1.000000000000000000, 1.000000000000000000, 1.000000000000000000, 1.000000000000000000, 1.000000000000000000, 1.000000000000000000, 1.000000000000000000, 1.000000000000000000, 1.000000000000000000, 1.000000000000000000, 1.000000000000000000, 1.000000000000000000, 1.000000000000000000, 1.000000000000000000, 1.000000000000000000, 1.000000000000000000, 1.000000000000000000, 1.000000000000000000, 1.000000000000000000, 1.000000000000000000, 1.000000000000000000, 1.000000000000000000, 1.000000000000000000, 1.000000000000000000, 1.000000000000000000, 1.000000000000000000, 1.000000000000000000, 1.000000000000000000, 1.000000000000000000, 1.000000000000000000, 1.000000000000000000, 1.000000000000000000, 1.000000000000000000, 1.000000000000000000, 1.000000000000000000, 1.000000000000000000, 1.000000000000000000, 1.000000000000000000, 1.000000000000000000, 1.000000000000000000, 1.000000000000000000, 1.000000000000000000, 1.000000000000000000, 1.000000000000000000, 1.000000000000000000, 1.000000000000000000, 1.000000000000000000, 1.000000000000000000, 1.000000000000000000, 1.000000000000000000, 1.000000000000000000, 1.000000000000000000, 1.000000000000000000, 1.000000000000000000, 1.000000000000000000, 1.000000000000000000, 1.000000000000000000, 1.000000000000000000, 1.000000000000000000, 1.000000000000000000, 1.000000000000000000, 1.000000000000000000, 1.000000000000000000, 1.000000000000000000, 1.000000000000000000, 1.000000000000000000, 1.000000000000000000),
 ( 0.3333333333333333703, 0.3333333333333333703, 0.3333333333333333703, 0.3333333333333333703, 0.3333333333333333703, 0.3333333333333333703, 0.3333333333333333703, 0.3333333333333333703, 0.3333333333333333703, 0.3333333333333333703, 0.3333333333333333703, 0.3333333333333333703, 0.3333333333333333703, 0.3333333333333333703, 0.3333333333333333703, 0.3333333333333333703, 0.3333333333333333703, 0.3333333333333333703, 0.3333333333333333703, 0.3333333333333333703, 0.3333333333333333703, 0.3333333333333333703, 0.3333333333333333703, 0.3333333333333333703, 0.3333333333333333703, 0.3333333333333333703, 0.3333333333333333703, 0.3333333333333333703, 0.3333333333333333703, 0.3333333333333333703, 0.3333333333333333703, 0.3333333333333333703, 0.3333333333333333703, 0.3333333333333333703, 0.3333333333333333703, 0.3333333333333333703, 0.3333333333333333703, 0.3333333333333333703, 0.3333333333333333703, 0.3333333333333333703, 0.3333333333333333703, 0.3333333333333333703, 0.3333333333333333703, 0.3333333333333333703, 0.3333333333333333703, 0.3333333333333333703, 0.3333333333333333703, 0.3333333333333333703, 0.3333333333333333703, 0.3333333333333333703, 0.3333333333333333703, 0.3333333333333333703, 0.3333333333333333703, 0.3333333333333333703, 0.3333333333333333703, 0.3333333333333333703, 0.3333333333333333703, 0.3333333333333333703, 0.3333333333333333703, 0.3333333333333333703, 0.3333333333333333703, 0.3333333333333333703, 0.3333333333333333703, 0.3333333333333333703, 0.3333333333333333703, 0.3333333333333333703, 0.3333333333333333703, 0.3333333333333333703, 0.3333333333333333703, 0.3333333333333333703, 0.3333333333333333703, 0.3333333333333333703, 0.3333333333333333703, 0.3333333333333333703, 0.3333333333333333703, 0.3333333333333333703, 0.3333333333333333703, 0.3333333333333333703, 0.3333333333333333703, 0.3333333333333333703, 0.3333333333333333703, 0.3333333333333333703, 0.3333333333333333703, 0.3333333333333333703, 0.3333333333333333703, 0.3333333333333333703),
 ( 0.3333333333333333703, 0.3333333333333333703, 0.3333333333333333703, 0.3333333333333333703, 0.3333333333333333703, 0.3333333333333333703, 0.3333333333333333703, 0.3333333333333333703, 0.3333333333333333703, 0.3333333333333333703, 0.3333333333333333703, 0.3333333333333333703, 0.3333333333333333703, 0.3333333333333333703, 0.3333333333333333703, 0.3333333333333333703, 0.3333333333333333703, 0.3333333333333333703, 0.3333333333333333703, 0.3333333333333333703, 0.3333333333333333703, 0.3333333333333333703, 0.3333333333333333703, 0.3333333333333333703, 0.3333333333333333703, 0.3333333333333333703, 0.3333333333333333703, 0.3333333333333333703, 0.3333333333333333703, 0.3333333333333333703, 0.3333333333333333703, 0.3333333333333333703, 0.3333333333333333703, 0.3333333333333333703, 0.3333333333333333703, 0.3333333333333333703, 0.3333333333333333703, 0.3333333333333333703, 0.3333333333333333703, 0.3333333333333333703, 0.3333333333333333703, 0.3333333333333333703, 0.3333333333333333703, 0.3333333333333333703, 0.3333333333333333703, 0.3333333333333333703, 0.3333333333333333703, 0.3333333333333333703, 0.3333333333333333703, 0.3333333333333333703, 0.3333333333333333703, 0.3333333333333333703, 0.3333333333333333703, 0.3333333333333333703, 0.3333333333333333703, 0.3333333333333333703, 0.3333333333333333703, 0.3333333333333333703, 0.3333333333333333703, 0.3333333333333333703, 0.3333333333333333703, 0.3333333333333333703, 0.3333333333333333703, 0.3333333333333333703, 0.3333333333333333703, 0.3333333333333333703, 0.3333333333333333703, 0.3333333333333333703, 0.3333333333333333703, 0.3333333333333333703, 0.3333333333333333703, 0.3333333333333333703, 0.3333333333333333703, 0.3333333333333333703, 0.3333333333333333703, 0.3333333333333333703, 0.3333333333333333703, 0.3333333333333333703, 0.3333333333333333703, 0.3333333333333333703, 0.3333333333333333703, 0.3333333333333333703, 0.3333333333333333703, 0.3333333333333333703, 0.3333333333333333703, 0.3333333333333333703),
 ( 1.000000000000000000, 1.000000000000000000, 1.000000000000000000, 1.000000000000000000, 1.000000000000000000, 1.000000000000000000, 1.000000000000000000, 1.000000000000000000, 1.000000000000000000, 1.000000000000000000, 1.000000000000000000, 1.000000000000000000, 1.000000000000000000, 1.000000000000000000, 1.000000000000000000, 1.000000000000000000, 1.000000000000000000, 1.000000000000000000, 1.000000000000000000, 1.000000000000000000, 1.000000000000000000, 1.000000000000000000, 1.000000000000000000, 1.000000000000000000, 1.000000000000000000, 1.000000000000000000, 1.000000000000000000, 1.000000000000000000, 1.000000000000000000, 1.000000000000000000, 1.000000000000000000, 1.000000000000000000, 1.000000000000000000, 1.000000000000000000, 1.000000000000000000, 1.000000000000000000, 1.000000000000000000, 1.000000000000000000, 1.000000000000000000, 1.000000000000000000, 1.000000000000000000, 1.000000000000000000, 1.000000000000000000, 1.000000000000000000, 1.000000000000000000, 1.000000000000000000, 1.000000000000000000, 1.000000000000000000, 1.000000000000000000, 1.000000000000000000, 1.000000000000000000, 1.000000000000000000, 1.000000000000000000, 1.000000000000000000, 1.000000000000000000, 1.000000000000000000, 1.000000000000000000, 1.000000000000000000, 1.000000000000000000, 1.000000000000000000, 1.000000000000000000, 1.000000000000000000, 1.000000000000000000, 1.000000000000000000, 1.000000000000000000, 1.000000000000000000, 1.000000000000000000, 1.000000000000000000, 1.000000000000000000, 1.000000000000000000, 1.000000000000000000, 1.000000000000000000, 1.000000000000000000, 1.000000000000000000, 1.000000000000000000, 1.000000000000000000, 1.000000000000000000, 1.000000000000000000, 1.000000000000000000, 1.000000000000000000, 1.000000000000000000, 1.000000000000000000, 1.000000000000000000, 1.000000000000000000, 1.000000000000000000, 1.000000000000000000),
 ( 0.3333333333333333703, 0.3333333333333333703, 0.3333333333333333703, 0.3333333333333333703, 0.3333333333333333703, 0.3333333333333333703, 0.3333333333333333703, 0.3333333333333333703, 0.3333333333333333703, 0.3333333333333333703, 0.3333333333333333703, 0.3333333333333333703, 0.3333333333333333703, 0.3333333333333333703, 0.3333333333333333703, 0.3333333333333333703, 0.3333333333333333703, 0.3333333333333333703, 0.3333333333333333703, 0.3333333333333333703, 0.3333333333333333703, 0.3333333333333333703, 0.3333333333333333703, 0.3333333333333333703, 0.3333333333333333703, 0.3333333333333333703, 0.3333333333333333703, 0.3333333333333333703, 0.3333333333333333703, 0.3333333333333333703, 0.3333333333333333703, 0.3333333333333333703, 0.3333333333333333703, 0.3333333333333333703, 0.3333333333333333703, 0.3333333333333333703, 0.3333333333333333703, 0.3333333333333333703, 0.3333333333333333703, 0.3333333333333333703, 0.3333333333333333703, 0.3333333333333333703, 0.3333333333333333703, 0.3333333333333333703, 0.3333333333333333703, 0.3333333333333333703, 0.3333333333333333703, 0.3333333333333333703, 0.3333333333333333703, 0.3333333333333333703, 0.3333333333333333703, 0.3333333333333333703, 0.3333333333333333703, 0.3333333333333333703, 0.3333333333333333703, 0.3333333333333333703, 0.3333333333333333703, 0.3333333333333333703, 0.3333333333333333703, 0.3333333333333333703, 0.3333333333333333703, 0.3333333333333333703, 0.3333333333333333703, 0.3333333333333333703, 0.3333333333333333703, 0.3333333333333333703, 0.3333333333333333703, 0.3333333333333333703, 0.3333333333333333703, 0.3333333333333333703, 0.3333333333333333703, 0.3333333333333333703, 0.3333333333333333703, 0.3333333333333333703, 0.3333333333333333703, 0.3333333333333333703, 0.3333333333333333703, 0.3333333333333333703, 0.3333333333333333703, 0.3333333333333333703, 0.3333333333333333703, 0.3333333333333333703, 0.3333333333333333703, 0.3333333333333333703, 0.3333333333333333703, 0.3333333333333333703),
 ( 0.3333333333333333703, 0.3333333333333333703, 0.3333333333333333703, 0.3333333333333333703, 0.3333333333333333703, 0.3333333333333333703, 0.3333333333333333703, 0.3333333333333333703, 0.3333333333333333703, 0.3333333333333333703, 0.3333333333333333703, 0.3333333333333333703, 0.3333333333333333703, 0.3333333333333333703, 0.3333333333333333703, 0.3333333333333333703, 0.3333333333333333703, 0.3333333333333333703, 0.3333333333333333703, 0.3333333333333333703, 0.3333333333333333703, 0.3333333333333333703, 0.3333333333333333703, 0.3333333333333333703, 0.3333333333333333703, 0.3333333333333333703, 0.3333333333333333703, 0.3333333333333333703, 0.3333333333333333703, 0.3333333333333333703, 0.3333333333333333703, 0.3333333333333333703, 0.3333333333333333703, 0.3333333333333333703, 0.3333333333333333703, 0.3333333333333333703, 0.3333333333333333703, 0.3333333333333333703, 0.3333333333333333703, 0.3333333333333333703, 0.3333333333333333703, 0.3333333333333333703, 0.3333333333333333703, 0.3333333333333333703, 0.3333333333333333703, 0.3333333333333333703, 0.3333333333333333703, 0.3333333333333333703, 0.3333333333333333703, 0.3333333333333333703, 0.3333333333333333703, 0.3333333333333333703, 0.3333333333333333703, 0.3333333333333333703, 0.3333333333333333703, 0.3333333333333333703, 0.3333333333333333703, 0.3333333333333333703, 0.3333333333333333703, 0.3333333333333333703, 0.3333333333333333703, 0.3333333333333333703, 0.3333333333333333703, 0.3333333333333333703, 0.3333333333333333703, 0.3333333333333333703, 0.3333333333333333703, 0.3333333333333333703, 0.3333333333333333703, 0.3333333333333333703, 0.3333333333333333703, 0.3333333333333333703, 0.3333333333333333703, 0.3333333333333333703, 0.3333333333333333703, 0.3333333333333333703, 0.3333333333333333703, 0.3333333333333333703, 0.3333333333333333703, 0.3333333333333333703, 0.3333333333333333703, 0.3333333333333333703, 0.3333333333333333703, 0.3333333333333333703, 0.3333333333333333703, 0.3333333333333333703),
 ( 1.000000000000000000, 1.000000000000000000, 1.000000000000000000, 1.000000000000000000, 1.000000000000000000, 1.000000000000000000, 1.000000000000000000, 1.000000000000000000, 1.000000000000000000, 1.000000000000000000, 1.000000000000000000, 1.000000000000000000, 1.000000000000000000, 1.000000000000000000, 1.000000000000000000, 1.000000000000000000, 1.000000000000000000, 1.000000000000000000, 1.000000000000000000, 1.000000000000000000, 1.000000000000000000, 1.000000000000000000, 1.000000000000000000, 1.000000000000000000, 1.000000000000000000, 1.000000000000000000, 1.000000000000000000, 1.000000000000000000, 1.000000000000000000, 1.000000000000000000, 1.000000000000000000, 1.000000000000000000, 1.000000000000000000, 1.000000000000000000, 1.000000000000000000, 1.000000000000000000, 1.000000000000000000, 1.000000000000000000, 1.000000000000000000, 1.000000000000000000, 1.000000000000000000, 1.000000000000000000, 1.000000000000000000, 1.000000000000000000, 1.000000000000000000, 1.000000000000000000, 1.000000000000000000, 1.000000000000000000, 1.000000000000000000, 1.000000000000000000, 1.000000000000000000, 1.000000000000000000, 1.000000000000000000, 1.000000000000000000, 1.000000000000000000, 1.000000000000000000, 1.000000000000000000, 1.000000000000000000, 1.000000000000000000, 1.000000000000000000, 1.000000000000000000, 1.000000000000000000, 1.000000000000000000, 1.000000000000000000, 1.000000000000000000, 1.000000000000000000, 1.000000000000000000, 1.000000000000000000, 1.000000000000000000, 1.000000000000000000, 1.000000000000000000, 1.000000000000000000, 1.000000000000000000, 1.000000000000000000, 1.000000000000000000, 1.000000000000000000, 1.000000000000000000, 1.000000000000000000, 1.000000000000000000, 1.000000000000000000, 1.000000000000000000, 1.000000000000000000, 1.000000000000000000, 1.000000000000000000, 1.000000000000000000, 1.000000000000000000) ) ) 
 REPRESENTATION_ITEM ( '' )  SURFACE ( )  );
#12565=CARTESIAN_POINT ( 'NONE',  ( -3.257364212367626966, -9.501732542047829355, 2.664600686199549706 ) ) ;
#12566=CARTESIAN_POINT ( 'NONE',  ( -13.83544900551672185, 3.002674778589386140, 5.971513032956590195 ) ) ;
#12570=CARTESIAN_POINT ( 'NONE',  ( 10.27780858231679417, -20.27099543870833642, 2.724438792969431589 ) ) ;
#12572=CARTESIAN_POINT ( 'NONE',  ( 13.02352923685845631, -0.8742735386340954040, 6.652704579156702991 ) ) ;
#12573=CARTESIAN_POINT ( 'NONE',  ( -5.965308582316795949, -19.47900456129164937, 4.484846433055089676 ) ) ;
#12574=CARTESIAN_POINT ( 'NONE',  ( -1.824218240560544047, -9.921717538097572842, 2.387231257717697286 ) ) ;
#12576=CARTESIAN_POINT ( 'NONE',  ( -13.37499999999998224, -20.25000000000006395, 4.416666666666681174 ) ) ;
#12579=CARTESIAN_POINT ( 'NONE',  ( 6.815941417683177406, -20.26807450282663225, 5.303608408759377113 ) ) ;
#12580=CARTESIAN_POINT ( 'NONE',  ( -11.49655858231679595, -22.05068747287764452, 2.499999999999999112 ) ) ;
#12582=EDGE_CURVE ( 'NONE', #19275, #12628, #4815, .T. ) ;
#12583=CARTESIAN_POINT ( 'NONE',  ( 13.37499999999998224, -20.99999999999998934, 4.291666666666699825 ) ) ;
#12591=ORIENTED_EDGE ( 'NONE', *, *, #3651, .F. ) ;
#12592=CARTESIAN_POINT ( 'NONE',  ( -4.218479777801761088, -21.67082477469113755, 4.835082305552395709 ) ) ;
#12594=CARTESIAN_POINT ( 'NONE',  ( -13.12499999999999645, 5.000000000000047073, 3.999999999999996447 ) ) ;
#12595=CARTESIAN_POINT ( 'NONE',  ( -2.693754455098655409, -10.04853567022903782, 2.237415670251142519 ) ) ;
#12596=CARTESIAN_POINT ( 'NONE',  ( 2.195822829018478473, -9.226849102155203042, 1.651390144731336163 ) ) ;
#12602=CARTESIAN_POINT ( 'NONE',  ( 4.472191417683178294, -22.97900456129165292, 3.035098964749240125 ) ) ;
#12603=CARTESIAN_POINT ( 'NONE',  ( -13.12529397354238192, 5.014845663890295846, 4.916666666666650087 ) ) ;
#12604=CARTESIAN_POINT ( 'NONE',  ( -9.340308582316795949, -22.36352608949544418, 4.520995438708343528 ) ) ;
#12605=CARTESIAN_POINT ( 'NONE',  ( -6.253441417683175629, -21.94931252712233061, 0.9999999999999978906 ) ) ;
#12608=CARTESIAN_POINT ( 'NONE',  ( 13.07121011584135672, 3.033610849983475521, 5.236678440007632496 ) ) ;
#12614=CARTESIAN_POINT ( 'NONE',  ( 2.559937518207947793, -9.746075135043517079, 2.534737762559237773 ) ) ;
#12617=CARTESIAN_POINT ( 'NONE',  ( 11.78469141768317563, -23.77099543870834353, 4.174186261275251830 ) ) ;
#12620=CARTESIAN_POINT ( 'NONE',  ( -1.903957340438703572, -10.27085516675799148, 2.476896775482616331 ) ) ;
#12622=CARTESIAN_POINT ( 'NONE',  ( -12.52780858231679595, -23.72900456129165292, 4.275561207030568411 ) ) ;
#12625=CARTESIAN_POINT ( 'NONE',  ( 4.940941417683177406, -20.19639159124061933, 1.768074502826635586 ) ) ;
#12626=DIRECTION ( 'NONE',  ( -1.000000000000000000, 0.000000000000000000, 0.000000000000000000 ) ) ;
#12627=CARTESIAN_POINT ( 'NONE',  ( -9.628441417683177406, -20.24999999999999289, 3.550687472877664952 ) ) ;
#12628=VERTEX_POINT ( 'NONE', #14219 ) ;
#12629=CARTESIAN_POINT ( 'NONE',  ( 9.152808582316794173, -21.22443879296942626, 5.229004561291659137 ) ) ;
#12631=CARTESIAN_POINT ( 'NONE',  ( -12.66024186180961308, -19.22028597861421417, 6.258173329156003106 ) ) ;
#12633=CARTESIAN_POINT ( 'NONE',  ( 9.152808582316794173, -21.22443879296942626, 5.229004561291659137 ) ) ;
#12635=ORIENTED_EDGE ( 'NONE', *, *, #15979, .F. ) ;
#12641=ORIENTED_EDGE ( 'NONE', *, *, #1059, .T. ) ;
#12642=CARTESIAN_POINT ( 'NONE',  ( -7.840308582316794173, -22.67418626127525982, 5.270995438708342640 ) ) ;
#12645=CARTESIAN_POINT ( 'NONE',  ( 2.282685604506861754, -11.80366834561962364, 2.120553820834011116 ) ) ;
#12648=CARTESIAN_POINT ( 'NONE',  ( -13.47561960997282071, -14.41870969638424071, 4.846833296715798767 ) ) ;
#12651=CARTESIAN_POINT ( 'NONE',  ( 9.246558582316794173, -21.94931252712234482, 5.250000000000000888 ) ) ;
#12652=CARTESIAN_POINT ( 'NONE',  ( -12.65986935584910000, -19.23909752961862907, 6.257782094979345899 ) ) ;
#12655=CARTESIAN_POINT ( 'NONE',  ( 5.309058582316794173, -23.27327832286945153, 2.298404588716537411 ) ) ;
#12656=CARTESIAN_POINT ( 'NONE',  ( 6.253441417683175629, -21.94931252712233061, 2.499999999999999112 ) ) ;
#12657=CARTESIAN_POINT ( 'NONE',  ( -10.94094141768317741, -20.72672167713052715, 2.298404588716546293 ) ) ;
#12659=CARTESIAN_POINT ( 'NONE',  ( 13.37732542738919328, -19.38256591684242025, 4.710253041318374301 ) ) ;
#12666=CARTESIAN_POINT ( 'NONE',  ( -13.12529418130016445, 5.014856155665242454, 4.958178834604180629 ) ) ;
#12669=CARTESIAN_POINT ( 'NONE',  ( -3.779650890485476200, -11.92851441922421607, 2.537846752097290715 ) ) ;
#12672=CARTESIAN_POINT ( 'NONE',  ( 2.768424032093183662, -10.00067216410020166, 1.850123365707658785 ) ) ;
#12673=CARTESIAN_POINT ( 'NONE',  ( -12.62499999999998224, -20.24999999999991829, 4.333333333333343695 ) ) ;
#12676=CARTESIAN_POINT ( 'NONE',  ( 13.15492785973632017, 5.761356916681801721, 5.116543252045025802 ) ) ;
#12677=CARTESIAN_POINT ( 'NONE',  ( -11.50344141768317741, -22.05068747287766229, 6.000000000000001776 ) ) ;
#12678=CARTESIAN_POINT ( 'NONE',  ( -2.044552395631970665, -10.13052631352519306, 1.690857522621936226 ) ) ;
#12682=CARTESIAN_POINT ( 'NONE',  ( -13.84501469867711698, 4.235742283194553259, 3.666666666666500873 ) ) ;
#12684=CARTESIAN_POINT ( 'NONE',  ( 8.409691417683177406, -21.01515356694492098, 6.020995438708349745 ) ) ;
#12685=( BOUNDED_CURVE ( )  B_SPLINE_CURVE ( 3, ( #8642, #10006, #11573, #15016 ),
 .UNSPECIFIED., .F., .F. ) 
 B_SPLINE_CURVE_WITH_KNOTS ( ( 4, 4 ),
 ( 0.001172421487176120289, 0.001187255941418635012 ),
 .UNSPECIFIED. ) 
 CURVE ( )  GEOMETRIC_REPRESENTATION_ITEM ( )  RATIONAL_B_SPLINE_CURVE ( ( 0.9999999999999996669, 0.9870550161812248202, 0.9743613912715525238, 0.9619191252709827777 ) ) 
 REPRESENTATION_ITEM ( '' )  );
#12686=CARTESIAN_POINT ( 'NONE',  ( -5.878441417683177406, -22.99999999999999645, 3.449312527122335048 ) ) ;
#12688=ORIENTED_EDGE ( 'NONE', *, *, #1611, .T. ) ;
#12689=CARTESIAN_POINT ( 'NONE',  ( 13.37499999999998224, -20.99999999999991829, 4.333333333333343695 ) ) ;
#12699=CARTESIAN_POINT ( 'NONE',  ( 2.203959450683124377, -9.262433282444222371, 2.410528873095051594 ) ) ;
#12702=CARTESIAN_POINT ( 'NONE',  ( 1.639793706121975614, -8.364901960018411131, 1.622639882261793343 ) ) ;
#12710=CARTESIAN_POINT ( 'NONE',  ( -2.602174906157317835, -9.976397331638239052, 2.593889103792902606 ) ) ;
#12711=CARTESIAN_POINT ( 'NONE',  ( 5.222191417683177406, -21.02099543870834353, 3.964901035250761208 ) ) ;
#12712=CARTESIAN_POINT ( 'NONE',  ( -13.12270769621861355, 4.884238659038159902, 5.513847264053151065 ) ) ;
#12713=CARTESIAN_POINT ( 'NONE',  ( -6.809058582316796837, -22.74294823697954016, 2.828734674606448785 ) ) ;
#12714=CARTESIAN_POINT ( 'NONE',  ( -11.97219141768317563, -23.72900456129165292, 2.724438792969417822 ) ) ;
#12716=CARTESIAN_POINT ( 'NONE',  ( 13.09123688038123490, 4.044962459253448550, 5.255034774807352704 ) ) ;
#12727=CARTESIAN_POINT ( 'NONE',  ( 11.97219141768317563, -23.72900456129164937, 2.724438792969417378 ) ) ;
#12731=CARTESIAN_POINT ( 'NONE',  ( -1.904508877737772998, -9.138371295333994837, 2.378667276417936627 ) ) ;
#12734=CARTESIAN_POINT ( 'NONE',  ( 6.722191417683176518, -19.52099543870834353, 4.586221378810406257 ) ) ;
#12736=CARTESIAN_POINT ( 'NONE',  ( -5.878441417683177406, -23.74999999999999645, 3.449312527122335492 ) ) ;
#12739=CARTESIAN_POINT ( 'NONE',  ( 7.090308582316794173, -21.32581373872472597, 1.729004561291657582 ) ) ;
#12741=CARTESIAN_POINT ( 'NONE',  ( -13.90439735423812273, 5.734566389025032684, 4.916666666666649199 ) ) ;
#12747=( NAMED_UNIT ( * ) SI_UNIT ( $, .STERADIAN. ) SOLID_ANGLE_UNIT ( ) );
#12751=CARTESIAN_POINT ( 'NONE',  ( -6.715308582316794173, -23.77099543870833998, 2.825813738724734847 ) ) ;
#12753=CARTESIAN_POINT ( 'NONE',  ( 12.62499999999998224, -20.24999999999998934, 4.166666666666636765 ) ) ;
#12755=CARTESIAN_POINT ( 'NONE',  ( 2.057814715640970515, -10.20705538578787852, 1.710511717200805304 ) ) ;
#12758=CARTESIAN_POINT ( 'NONE',  ( -13.83051420738022763, 3.503467472703414742, 5.232249963382380464 ) ) ;
#12759=CARTESIAN_POINT ( 'NONE',  ( 7.465308582316795061, -20.22900456129164937, 4.174186261275266929 ) ) ;
#12760=CARTESIAN_POINT ( 'NONE',  ( -12.67822638532683577, -18.31206754099172684, 6.277704579156187847 ) ) ;
#12762=CARTESIAN_POINT ( 'NONE',  ( -6.527808582316795949, -24.47900456129166358, 4.586221378810390270 ) ) ;
#12763=CARTESIAN_POINT ( 'NONE',  ( 7.465308582316795061, -20.22900456129164937, 4.174186261275266929 ) ) ;
#12766=CARTESIAN_POINT ( 'NONE',  ( 4.190941417683176518, -22.74294823697955081, 4.171265325393542334 ) ) ;
#12767=CARTESIAN_POINT ( 'NONE',  ( -5.222191417683177406, -20.27099543870833998, 4.275561207030583510 ) ) ;
#12769=CARTESIAN_POINT ( 'NONE',  ( 13.84167967300649238, 4.067323486828401613, 5.231641758301140754 ) ) ;
#12770=DIRECTION ( 'NONE',  ( 0.1351665943404306014, 0.9596796555888912339, -0.2464649070825229438 ) ) ;
#12777=CARTESIAN_POINT ( 'NONE',  ( -3.336296098497695262, -9.936854405034125648, 2.776348673047012383 ) ) ;
#12780=CARTESIAN_POINT ( 'NONE',  ( 2.195822829018478473, -9.226849102155203042, 1.651390144731336163 ) ) ;
#12781=CARTESIAN_POINT ( 'NONE',  ( -13.10557919622060652, 4.019249409169220577, 6.007898877577752650 ) ) ;
#12784=CARTESIAN_POINT ( 'NONE',  ( 12.81251082758882376, -11.53070320674076576, 6.423537912489145185 ) ) ;
#12785=CARTESIAN_POINT ( 'NONE',  ( -1.897597015127918230, -9.924601616748528699, 1.637971946730535588 ) ) ;
#12787=CARTESIAN_POINT ( 'NONE',  ( -13.87406079471522347, 4.952570133121557028, 5.260711232101737522 ) ) ;
#12789=CARTESIAN_POINT ( 'NONE',  ( 8.784691417683177406, -24.52099543870834708, 4.484846433055073689 ) ) ;
#12791=CARTESIAN_POINT ( 'NONE',  ( -11.21530858231679595, -23.02099543870833998, 3.136473910504556262 ) ) ;
#12793=CARTESIAN_POINT ( 'NONE',  ( 12.62499999999998224, -21.00000000000006395, 4.416666666666682062 ) ) ;
#12794=CARTESIAN_POINT ( 'NONE',  ( 13.12529418130016445, 5.014856155665242454, 4.958178834604180629 ) ) ;
#12807=CARTESIAN_POINT ( 'NONE',  ( 2.512468814886674284, -13.43512376012158782, 2.539544162874482591 ) ) ;
#12813=CARTESIAN_POINT ( 'NONE',  ( -2.594671182134835163, -9.923034775318452461, 2.580184533305832861 ) ) ;
#12814=CARTESIAN_POINT ( 'NONE',  ( 11.12155858231679595, -22.99999999999999645, 3.550687472877652073 ) ) ;
#12815=CARTESIAN_POINT ( 'NONE',  ( -13.09080647246885576, 4.023226859705822278, 5.257958009367514229 ) ) ;
#12816=CARTESIAN_POINT ( 'NONE',  ( -4.717959273841179524, -21.82295283170803302, 4.493595146365858994 ) ) ;
#12817=CARTESIAN_POINT ( 'NONE',  ( -5.597191417683177406, -23.08622137881040359, 5.979004561291654696 ) ) ;
#12819=CARTESIAN_POINT ( 'NONE',  ( 13.37499994994395891, -19.50000252782794519, 4.474109982178703149 ) ) ;
#12828=CARTESIAN_POINT ( 'NONE',  ( 9.440941417683177406, -20.72672167713052715, 2.298404588716546293 ) ) ;
#12829=CARTESIAN_POINT ( 'NONE',  ( -4.315753587183824180, -21.56469153729574018, 5.194994555241421175 ) ) ;
#12830=CARTESIAN_POINT ( 'NONE',  ( -2.579281110863027582, -9.822567596814183233, 2.554382554832406615 ) ) ;
#12834=CARTESIAN_POINT ( 'NONE',  ( 8.128441417683175629, -20.24999999999999289, 3.550687472877664952 ) ) ;
#12836=CARTESIAN_POINT ( 'NONE',  ( -12.53469141768317741, -20.97900456129164581, 3.136473910504570917 ) ) ;
#12838=CARTESIAN_POINT ( 'NONE',  ( 7.371558582316795949, -19.49999999999998934, 3.449312527122348371 ) ) ;
#12840=CARTESIAN_POINT ( 'NONE',  ( -13.90411326029870409, 5.720219645086723759, 5.230514352905474063 ) ) ;
#12842=CARTESIAN_POINT ( 'NONE',  ( 4.687312169500632564, -21.51559725698341197, 5.182386163300427562 ) ) ;
#12848=( LENGTH_UNIT ( ) NAMED_UNIT ( * ) SI_UNIT ( .MILLI., .METRE. ) );
#12852=CARTESIAN_POINT ( 'NONE',  ( -5.684058582316794173, -20.79840458871652942, 2.226721677130544030 ) ) ;
#12855=CARTESIAN_POINT ( 'NONE',  ( 2.050137595624097031, -10.15260257655714504, 1.696527147986202522 ) ) ;
#12856=CARTESIAN_POINT ( 'NONE',  ( 12.64195242771744709, -19.39390240027112000, 5.496549442168085164 ) ) ;
#12858=CARTESIAN_POINT ( 'NONE',  ( -13.38269957179998038, -19.11117162410040038, 4.745921838382382241 ) ) ;
#12859=CARTESIAN_POINT ( 'NONE',  ( 8.965308582316794173, -20.22900456129164937, 4.174186261275266929 ) ) ;
#12860=CARTESIAN_POINT ( 'NONE',  ( -13.90439735423812273, 5.734566389025032684, 4.916666666666649199 ) ) ;
#12862=CARTESIAN_POINT ( 'NONE',  ( -10.27780858231679595, -19.52099543870833642, 2.413778621189609286 ) ) ;
#12863=CARTESIAN_POINT ( 'NONE',  ( 4.687312169500632564, -21.51559725698341197, 5.182386163300427562 ) ) ;
#12866=CARTESIAN_POINT ( 'NONE',  ( 7.659691417683177406, -22.36352608949543352, 2.479004561291652031 ) ) ;
#12867=CARTESIAN_POINT ( 'NONE',  ( -6.909691417683177406, -21.32581373872474373, 5.270995438708348857 ) ) ;
#12870=CARTESIAN_POINT ( 'NONE',  ( 13.37499999999998224, -20.25000000000006395, 4.416666666666681174 ) ) ;
#12878=CARTESIAN_POINT ( 'NONE',  ( 0.000000000000000000, -9.114917468222230923, 2.372643865078340575 ) ) ;
#12881=FACE_OUTER_BOUND ( 'NONE', #18476, .T. ) ;
#12882=CARTESIAN_POINT ( 'NONE',  ( -13.10192273101908000, 3.834597916462216816, 6.003936301248457674 ) ) ;
#12883=CARTESIAN_POINT ( 'NONE',  ( 12.52780858231679595, -23.72900456129165292, 4.275561207030568411 ) ) ;
#12885=CARTESIAN_POINT ( 'NONE',  ( 13.15498530132288479, 5.764257716805535559, 4.333333333333380999 ) ) ;
#12886=CARTESIAN_POINT ( 'NONE',  ( -1.991511895312070957, -10.01421418592441448, 1.660986244685804136 ) ) ;
#12888=CARTESIAN_POINT ( 'NONE',  ( -13.37499999999998401, -20.99999999999999645, 3.666666666666654084 ) ) ;
#12890=CARTESIAN_POINT ( 'NONE',  ( 5.034691417683177406, -19.47900456129164581, 2.515153566944927199 ) ) ;
#12891=CARTESIAN_POINT ( 'NONE',  ( -9.621558582316795949, -22.99999999999999645, 3.550687472877652073 ) ) ;
#12893=CARTESIAN_POINT ( 'NONE',  ( 13.90394305879618386, 5.711624469205903942, 5.287712306078340418 ) ) ;
#12894=CARTESIAN_POINT ( 'NONE',  ( 12.68288333306630378, -17.32689168014509207, 5.548858176248425700 ) ) ;
#12902=CARTESIAN_POINT ( 'NONE',  ( 2.041623931606483033, -10.12028065167953272, 1.688226231982305370 ) ) ;
#12904=AXIS2_PLACEMENT_3D ( 'NONE', #5262, #13308, #3805 ) ;
#12910=CARTESIAN_POINT ( 'NONE',  ( -1.126276606324276619, -9.114917468222230923, 2.372643865078341019 ) ) ;
#12912=CARTESIAN_POINT ( 'NONE',  ( -12.63118877378512828, -19.18746692385052555, 4.758813856674282583 ) ) ;
#12913=CARTESIAN_POINT ( 'NONE',  ( -5.027808582316795949, -22.97900456129165647, 3.964901035250747885 ) ) ;
#12914=CARTESIAN_POINT ( 'NONE',  ( -5.597191417683179182, -22.77556120703057729, 5.229004561291655584 ) ) ;
#12916=CARTESIAN_POINT ( 'NONE',  ( 13.84051394328565365, 4.008454135954084840, 5.243107695145536873 ) ) ;
#12926=CARTESIAN_POINT ( 'NONE',  ( 10.56594141768317741, -23.20159541128344927, 2.226721677130534705 ) ) ;
#12928=CARTESIAN_POINT ( 'NONE',  ( 0.000000000000000000, -9.114917468222230923, 2.372643865078340575 ) ) ;
#12930=CARTESIAN_POINT ( 'NONE',  ( -11.96530858231679417, -20.22900456129164937, 4.174186261275266929 ) ) ;
#12933=CARTESIAN_POINT ( 'NONE',  ( 11.69094141768317563, -23.27327832286946219, 4.701595411283453707 ) ) ;
#12935=CARTESIAN_POINT ( 'NONE',  ( -10.84719141768317741, -21.53509896474923835, 2.520995438708346192 ) ) ;
#12937=CARTESIAN_POINT ( 'NONE',  ( 10.46530858231679595, -19.47900456129164937, 4.484846433055089676 ) ) ;
#12938=ADVANCED_FACE ( 'NONE', ( #16830 ), #18994, .F. ) ;
#12939=CARTESIAN_POINT ( 'NONE',  ( 13.10756170493883310, 4.119366099410778581, 6.001761809183453700 ) ) ;
#12940=CARTESIAN_POINT ( 'NONE',  ( -12.64323021897839006, -19.32937394158751943, 5.504219675487169283 ) ) ;
#12944=CARTESIAN_POINT ( 'NONE',  ( 13.12509927631103501, 5.009931486494128450, 3.999999999999983125 ) ) ;
#12952=CARTESIAN_POINT ( 'NONE',  ( -12.24655858231679595, -21.94931252712234127, 6.000000000000001776 ) ) ;
#12956=CARTESIAN_POINT ( 'NONE',  ( 1.711347482507859397, -9.865394108634699677, 1.622766275858107621 ) ) ;
#12959=CARTESIAN_POINT ( 'NONE',  ( 13.05696142222617695, 1.564051822406025583, 5.955108176248398166 ) ) ;
#12961=CARTESIAN_POINT ( 'NONE',  ( -13.84501469867711698, 4.235742283194553259, 4.791666666666684726 ) ) ;
#12962=CARTESIAN_POINT ( 'NONE',  ( 8.309058582316795949, -23.80360840875935935, 1.768074502826626260 ) ) ;
#12963=CARTESIAN_POINT ( 'NONE',  ( -13.13728495444130751, 4.870390199291127153, 6.548325014280736767 ) ) ;
#12967=CARTESIAN_POINT ( 'NONE',  ( 3.974842109207560537, -21.92432777746334693, 4.506404853634142782 ) ) ;
#12968=CARTESIAN_POINT ( 'NONE',  ( -9.628441417683177406, -20.24999999999999289, 3.550687472877664952 ) ) ;
#12972=CARTESIAN_POINT ( 'NONE',  ( 13.83411111208379474, 3.685111160228107252, 5.236156213382356484 ) ) ;
#12983=CARTESIAN_POINT ( 'NONE',  ( 0.000000000000000000, -8.364917468222230923, 1.622643865078341241 ) ) ;
#12988=CARTESIAN_POINT ( 'NONE',  ( -13.10624331898488037, 4.052787608736739600, 6.006964772046813117 ) ) ;
#12991=CARTESIAN_POINT ( 'NONE',  ( 12.64751377014909828, -19.11305460747000495, 5.510446717915143289 ) ) ;
#12992=CARTESIAN_POINT ( 'NONE',  ( -0.5631383031621635116, -9.864917468222230923, 2.372643865078341019 ) ) ;
#12994=CARTESIAN_POINT ( 'NONE',  ( -13.85528666703740619, 4.004476685417483139, 5.993048563355776182 ) ) ;
#12996=CARTESIAN_POINT ( 'NONE',  ( 6.347191417683176518, -20.91377862118959285, 1.020995438708345082 ) ) ;
#12997=CARTESIAN_POINT ( 'NONE',  ( -4.934058582316795061, -22.67126532539354855, 4.242948236979545484 ) ) ;
#12999=CARTESIAN_POINT ( 'NONE',  ( 13.60059015675642513, -9.607697083824668027, 6.450359435862663027 ) ) ;
#13000=CARTESIAN_POINT ( 'NONE',  ( 13.10012427866737639, 3.743776072700027324, 6.001983176248468332 ) ) ;
#13009=CARTESIAN_POINT ( 'NONE',  ( -13.37327929115833491, -20.24999999560066399, 3.449077790995343840 ) ) ;
#13012=CARTESIAN_POINT ( 'NONE',  ( 1.859341899742023463, -9.902476528685241419, 1.632289782122827271 ) ) ;
#13019=CARTESIAN_POINT ( 'NONE',  ( -12.80487140268466817, -20.58484656434375637, 3.526619154972564285 ) ) ;
#13021=CARTESIAN_POINT ( 'NONE',  ( -12.72590726430969532, -14.40418315237199742, 4.861678440007700885 ) ) ;
#13022=CARTESIAN_POINT ( 'NONE',  ( -4.934058582316795061, -22.67126532539354855, 4.242948236979545484 ) ) ;
#13024=CARTESIAN_POINT ( 'NONE',  ( -6.159691417683176518, -22.67418626127524917, 1.729004561291651809 ) ) ;
#13026=CARTESIAN_POINT ( 'NONE',  ( 13.84476264919594612, 4.223013784394161974, 5.079233071712400793 ) ) ;
#13028=VERTEX_POINT ( 'NONE', #18182 ) ;
#13035=AXIS2_PLACEMENT_3D ( 'NONE', #125, #6713, #6510 ) ;
#13040=CARTESIAN_POINT ( 'NONE',  ( -1.668644041176298387, -9.864915931696323526, 2.372643470467795890 ) ) ;
#13041=CARTESIAN_POINT ( 'NONE',  ( 2.109407804498405703, -9.207748739546751438, 2.396484790045401603 ) ) ;
#13042=CARTESIAN_POINT ( 'NONE',  ( -11.40280858231679595, -22.77556120703056308, 1.770995438708340197 ) ) ;
#13044=CARTESIAN_POINT ( 'NONE',  ( 6.815941417683176518, -20.79840458871654363, 4.773278322869464851 ) ) ;
#13046=CARTESIAN_POINT ( 'NONE',  ( -10.56594141768317741, -22.67126532539353789, 2.757051763020445634 ) ) ;
#13048=CARTESIAN_POINT ( 'NONE',  ( 9.902808582316795949, -23.08622137881038938, 1.020995438708339309 ) ) ;
#13049=CARTESIAN_POINT ( 'NONE',  ( 12.64571531779736979, -19.20387645123237164, 5.508493592915143289 ) ) ;
#13050=CARTESIAN_POINT ( 'NONE',  ( -12.62500016093973620, -20.24999187254239175, 4.532396751752561848 ) ) ;
#13062=CARTESIAN_POINT ( 'NONE',  ( -11.40280858231679595, -23.08622137881038938, 1.020995438708339309 ) ) ;
#13063=CARTESIAN_POINT ( 'NONE',  ( 13.06655316810189227, 2.048434989138931961, 5.965524842914772030 ) ) ;
#13068=CARTESIAN_POINT ( 'NONE',  ( 12.95145221759166354, -3.764163011652346569, 5.840524842913703552 ) ) ;
#13070=CARTESIAN_POINT ( 'NONE',  ( -13.37500000000002132, -20.24999999999450040, 3.833333333368183382 ) ) ;
#13071=CARTESIAN_POINT ( 'NONE',  ( 12.05905858231679595, -20.19639159124062999, 5.231925497173373074 ) ) ;
#13072=CARTESIAN_POINT ( 'NONE',  ( -12.62499999999998579, -20.24999999999999289, 3.146526952850934755 ) ) ;
#13073=CARTESIAN_POINT ( 'NONE',  ( -6.152808582316795949, -20.91377862118960351, 5.979004561291660913 ) ) ;
#13076=CARTESIAN_POINT ( 'NONE',  ( 8.402808582316797725, -22.46490103525074034, 2.520995438708341307 ) ) ;
#13077=CARTESIAN_POINT ( 'NONE',  ( -7.753441417683176518, -21.94931252712233061, 1.749999999999998446 ) ) ;
#13080=CARTESIAN_POINT ( 'NONE',  ( 13.38238173943565990, -19.87722215849730034, 5.285856107751903288 ) ) ;
#13089=CARTESIAN_POINT ( 'NONE',  ( 13.37499979530394967, -20.25001033714808329, 4.458488164327452097 ) ) ;
#13092=CARTESIAN_POINT ( 'NONE',  ( -12.64571531779736979, -19.20387645123237164, 5.508493592915143289 ) ) ;
#13093=CARTESIAN_POINT ( 'NONE',  ( 4.934058582316793284, -23.20159541128345992, 4.773278322869455970 ) ) ;
#13095=CARTESIAN_POINT ( 'NONE',  ( 13.10252221513633941, 3.864871864382954048, 6.004587342915129966 ) ) ;
#13097=CARTESIAN_POINT ( 'NONE',  ( -3.047379876266447685, -13.13734219723468755, 3.405682891496055742 ) ) ;
#13099=CARTESIAN_POINT ( 'NONE',  ( -13.87215786865436762, 4.856472367046606564, 5.506273593909547515 ) ) ;
#13101=CARTESIAN_POINT ( 'NONE',  ( 9.909691417683179182, -21.32581373872474373, 5.270995438708348857 ) ) ;
#13102=CARTESIAN_POINT ( 'NONE',  ( -10.65280858231679595, -21.53509896474924901, 4.479004561291659137 ) ) ;
#13104=CARTESIAN_POINT ( 'NONE',  ( 13.87824226375436965, 4.413734319597230282, 6.694665752684481497 ) ) ;
#13105=CARTESIAN_POINT ( 'NONE',  ( 13.02818618459764188, 0.1109023222084986743, 5.923858176248589125 ) ) ;
#13118=CARTESIAN_POINT ( 'NONE',  ( 0.2815691515810352930, -9.114917468222230923, 1.622643865078524206 ) ) ;
#13124=CARTESIAN_POINT ( 'NONE',  ( -8.215308582316792396, -23.77099543870833998, 2.825813738724734847 ) ) ;
#13125=CARTESIAN_POINT ( 'NONE',  ( -3.211992482548209349, -9.366834950279640637, 2.629956289783360823 ) ) ;
#13127=CARTESIAN_POINT ( 'NONE',  ( -13.08439876642066935, 3.699637704240349656, 5.251001356674258602 ) ) ;
#13128=CARTESIAN_POINT ( 'NONE',  ( -10.27780858231679417, -20.27099543870833642, 2.724438792969431589 ) ) ;
#13130=CARTESIAN_POINT ( 'NONE',  ( -9.065941417683177406, -23.20159541128344927, 2.226721677130534705 ) ) ;
#13132=CARTESIAN_POINT ( 'NONE',  ( 13.64827103573800571, -5.699812695207630675, 5.034333296717131034 ) ) ;
#13141=CARTESIAN_POINT ( 'NONE',  ( 4.378441417683176518, -23.74999999999999645, 3.449312527122335492 ) ) ;
#13148=CARTESIAN_POINT ( 'NONE',  ( 11.59719141768317563, -22.77556120703057729, 5.229004561291655584 ) ) ;
#13150=CARTESIAN_POINT ( 'NONE',  ( -10.09719141768317741, -22.46490103525075810, 4.479004561291653808 ) ) ;
#13152=CARTESIAN_POINT ( 'NONE',  ( 8.684058582316795949, -20.26807450282662160, 1.696391591240633101 ) ) ;
#13153=CARTESIAN_POINT ( 'NONE',  ( 12.65650603190776025, -18.65894538865861563, 5.520212342915047365 ) ) ;
#13154=CARTESIAN_POINT ( 'NONE',  ( -12.62499999999998224, -20.24999999999998934, 4.166666666666636765 ) ) ;
#13164=CARTESIAN_POINT ( 'NONE',  ( 13.12529397354238192, 5.014845663890295846, 4.791666666666685614 ) ) ;
#13166=CARTESIAN_POINT ( 'NONE',  ( 13.15498530132288479, 5.764257716805535559, 4.333333333333380999 ) ) ;
#13168=CARTESIAN_POINT ( 'NONE',  ( -13.37499999999998224, -20.24999999999998934, 4.291666666666698937 ) ) ;
#13169=CARTESIAN_POINT ( 'NONE',  ( 12.43405858231679595, -23.73192549717337130, 5.303608408759367343 ) ) ;
#13170=CARTESIAN_POINT ( 'NONE',  ( -12.62499999999998224, -20.24999999999991829, 4.333333333333343695 ) ) ;
#13171=CARTESIAN_POINT ( 'NONE',  ( -12.06594141768317741, -23.73192549717336064, 1.696391591240623331 ) ) ;
#13175=CARTESIAN_POINT ( 'NONE',  ( 9.059058582316795949, -21.25705176302045274, 4.171265325393551215 ) ) ;
#13176=CARTESIAN_POINT ( 'NONE',  ( -4.565941417683176518, -23.20159541128344927, 2.226721677130534705 ) ) ;
#13180=CARTESIAN_POINT ( 'NONE',  ( 13.39107665282975645, -19.43812903209671461, 5.476542851584349947 ) ) ;
#13188=CARTESIAN_POINT ( 'NONE',  ( 13.80667376788930056, 1.549525278393783179, 5.940263032956496048 ) ) ;
#13190=CARTESIAN_POINT ( 'NONE',  ( 1.548630333695928396, -9.114917468222230923, 2.372643865078341019 ) ) ;
#13192=CARTESIAN_POINT ( 'NONE',  ( -12.67794853492974561, -16.82609898603114118, 4.809595106674325216 ) ) ;
#13193=CARTESIAN_POINT ( 'NONE',  ( 8.965308582316794173, -20.22900456129164937, 4.174186261275266929 ) ) ;
#13195=CARTESIAN_POINT ( 'NONE',  ( 12.63943061533661982, -19.52125392549825733, 5.470334935344855154 ) ) ;
#13197=CARTESIAN_POINT ( 'NONE',  ( -2.367358971471363649, -9.400572650371021410, 2.446005822389718087 ) ) ;
#13198=CARTESIAN_POINT ( 'NONE',  ( 10.18405858231679595, -21.32873467460644079, 2.757051763020455404 ) ) ;
#13199=CARTESIAN_POINT ( 'NONE',  ( 11.78469141768317563, -23.77099543870834353, 4.174186261275252718 ) ) ;
#13200=CARTESIAN_POINT ( 'NONE',  ( -5.777808582316795949, -21.02099543870833998, 3.035098964749253003 ) ) ;
#13202=CARTESIAN_POINT ( 'NONE',  ( 12.62499999999998401, -20.99999999999999645, 3.666666666666654084 ) ) ;
#13203=CARTESIAN_POINT ( 'NONE',  ( 12.64931222250080545, -19.02223276370786209, 5.512399842915133519 ) ) ;
#13204=CARTESIAN_POINT ( 'NONE',  ( -13.84667963294518778, 4.277765388965502957, 4.000000000000000888 ) ) ;
#13212=CARTESIAN_POINT ( 'NONE',  ( 2.057814715640970515, -10.20705538578787852, 1.710511717200805304 ) ) ;
#13215=CARTESIAN_POINT ( 'NONE',  ( 12.72644768880819477, -20.50652430979270946, 3.537312097732761895 ) ) ;
#13216=CARTESIAN_POINT ( 'NONE',  ( -2.367358971471363649, -9.400572650371021410, 2.446005822389718087 ) ) ;
#13217=CARTESIAN_POINT ( 'NONE',  ( -6.527808582316794173, -23.72900456129165647, 4.275561207030568411 ) ) ;
#13219=CARTESIAN_POINT ( 'NONE',  ( -3.951988298270009636, -13.15210598010094323, 2.852089508627633219 ) ) ;
#13222=CARTESIAN_POINT ( 'NONE',  ( -12.67794853492974561, -16.82609898603114118, 4.809595106674325216 ) ) ;
#13223=CARTESIAN_POINT ( 'NONE',  ( -7.934058582316792396, -23.20159541128345992, 4.773278322869455970 ) ) ;
#13224=CARTESIAN_POINT ( 'NONE',  ( -7.472191417683176518, -23.72900456129165292, 2.724438792969417822 ) ) ;
#13226=CARTESIAN_POINT ( 'NONE',  ( 13.68663801924254741, -3.762280028282741551, 5.075999963380942503 ) ) ;
#13232=CARTESIAN_POINT ( 'NONE',  ( -13.39170256340046095, -19.40652054827866380, 5.481861153867630065 ) ) ;
#13235=CARTESIAN_POINT ( 'NONE',  ( 4.659691417683178294, -22.67418626127524917, 1.729004561291651587 ) ) ;
#13239=CARTESIAN_POINT ( 'NONE',  ( -5.777808582316794173, -20.27099543870833642, 2.724438792969431589 ) ) ;
#13243=CARTESIAN_POINT ( 'NONE',  ( 11.12844141768317741, -20.24999999999999289, 3.550687472877664952 ) ) ;
#13245=CARTESIAN_POINT ( 'NONE',  ( -5.690941417683177406, -22.74294823697955081, 4.171265325393542334 ) ) ;
#13246=CARTESIAN_POINT ( 'NONE',  ( -9.715308582316795949, -24.52099543870834708, 2.515153566944913432 ) ) ;
#13248=CARTESIAN_POINT ( 'NONE',  ( 12.66849571425264287, -18.05346643024382303, 5.533233176248494978 ) ) ;
#13249=CARTESIAN_POINT ( 'NONE',  ( -12.62499979224180180, -20.25001049178813162, 4.458178821399696012 ) ) ;
#13258=CARTESIAN_POINT ( 'NONE',  ( 2.579281110863027582, -9.822567596814183233, 2.554382554832406615 ) ) ;
#13261=CARTESIAN_POINT ( 'NONE',  ( 12.91308523408712183, -5.701695678577235249, 5.798858176249892082 ) ) ;
#13262=CARTESIAN_POINT ( 'NONE',  ( 1.513434189748285696, -9.114917468222230923, 2.372643865078341019 ) ) ;
#13264=CARTESIAN_POINT ( 'NONE',  ( 12.64387510712649565, -19.29680709011273976, 5.506486987317513737 ) ) ;
#13266=CARTESIAN_POINT ( 'NONE',  ( 8.121558582316795949, -24.50000000000000000, 3.550687472877651629 ) ) ;
#13267=CARTESIAN_POINT ( 'NONE',  ( -12.62515553039088090, -20.24214571525854467, 4.629702272822510345 ) ) ;
#13268=CARTESIAN_POINT ( 'NONE',  ( -12.34719141768317741, -20.91377862118959285, 1.020995438708345082 ) ) ;
#13271=CARTESIAN_POINT ( 'NONE',  ( 7.746558582316795949, -21.94931252712234127, 4.499999999999999112 ) ) ;
#13275=CARTESIAN_POINT ( 'NONE',  ( 13.87470602645761986, 4.985154336109792972, 4.583333333333296622 ) ) ;
#13284=CARTESIAN_POINT ( 'NONE',  ( 13.85163507668220539, 3.820071372449974412, 5.989091157956555556 ) ) ;
#13287=CARTESIAN_POINT ( 'NONE',  ( 3.034277558025862298, -9.029550313327863620, 2.543334857076493094 ) ) ;
#13289=CARTESIAN_POINT ( 'NONE',  ( -12.62837453896009876, -19.32958578251692572, 4.742959489302074338 ) ) ;
#13290=CARTESIAN_POINT ( 'NONE',  ( 5.402808582316794173, -22.77556120703056308, 1.770995438708340197 ) ) ;
#13292=CARTESIAN_POINT ( 'NONE',  ( 13.12512971825177033, 5.006550771716304915, 5.133277049491872468 ) ) ;
#13294=CARTESIAN_POINT ( 'NONE',  ( -0.5631383031621635116, -9.114917468222230923, 2.372643865078341019 ) ) ;
#13295=CARTESIAN_POINT ( 'NONE',  ( 11.59030858231679595, -21.63647391050454871, 2.479004561291657804 ) ) ;
#13296=CARTESIAN_POINT ( 'NONE',  ( 7.659691417683177406, -22.67418626127524917, 1.729004561291651809 ) ) ;
#13297=CARTESIAN_POINT ( 'NONE',  ( -6.527808582316795949, -22.97900456129165647, 3.964901035250747885 ) ) ;
#13299=CARTESIAN_POINT ( 'NONE',  ( 12.92761177809936513, -5.718105205959081339, 6.548537912490751900 ) ) ;
#13300=CARTESIAN_POINT ( 'NONE',  ( 13.09173631808601002, 4.070184063342107805, 5.250510817581989009 ) ) ;
#13308=DIRECTION ( 'NONE',  ( -0.000000000000000000, -0.000000000000000000, -1.000000000000000000 ) ) ;
#13313=CARTESIAN_POINT ( 'NONE',  ( -4.218479777801761976, -21.48426400496073541, 5.561508543513003389 ) ) ;
#13314=CARTESIAN_POINT ( 'NONE',  ( 3.162271481458107658, -13.95306990448253437, 3.615178062515473911 ) ) ;
#13318=CARTESIAN_POINT ( 'NONE',  ( 13.25392420457524878, -20.52600657937462358, 3.465375001445726966 ) ) ;
#13320=CARTESIAN_POINT ( 'NONE',  ( -5.684058582316794173, -20.79840458871652942, 2.226721677130544030 ) ) ;
#13322=CARTESIAN_POINT ( 'NONE',  ( -1.337453470010121714, -8.364917468222230923, 2.372643865078341019 ) ) ;
#13325=CARTESIAN_POINT ( 'NONE',  ( -13.38269957179998038, -19.11117162410040038, 4.745921838382382241 ) ) ;
#13326=CARTESIAN_POINT ( 'NONE',  ( -7.559058582316794173, -20.72672167713054137, 4.701595411283463477 ) ) ;
#13327=CARTESIAN_POINT ( 'NONE',  ( -8.409691417683177406, -21.32581373872474373, 5.270995438708348857 ) ) ;
#13330=CARTESIAN_POINT ( 'NONE',  ( 13.38238173943565990, -19.87722215849730034, 5.285856107751903288 ) ) ;
#13340=CARTESIAN_POINT ( 'NONE',  ( 7.003441417683177406, -22.05068747287765873, 5.250000000000000888 ) ) ;
#13345=CARTESIAN_POINT ( 'NONE',  ( 4.181771508648414404, -14.78356139460145968, 3.271079850667843125 ) ) ;
#13346=CARTESIAN_POINT ( 'NONE',  ( -6.902808582316795061, -22.77556120703056308, 1.770995438708340197 ) ) ;
#13347=CARTESIAN_POINT ( 'NONE',  ( 12.62499999999998224, -20.99999999999991829, 4.333333333333343695 ) ) ;
#13349=CARTESIAN_POINT ( 'NONE',  ( 12.15969141768317918, -22.36352608949543352, 2.479004561291652031 ) ) ;
#13352=CARTESIAN_POINT ( 'NONE',  ( -9.253441417683177406, -21.94931252712233061, 2.499999999999999112 ) ) ;
#13353=CARTESIAN_POINT ( 'NONE',  ( -6.340308582316796837, -22.98484643305508612, 6.020995438708344416 ) ) ;
#13355=CARTESIAN_POINT ( 'NONE',  ( 13.10431844137356627, 3.955581289335645234, 6.006545679920360925 ) ) ;
#13356=CARTESIAN_POINT ( 'NONE',  ( -12.62499999999998579, -20.24999999999999289, 3.146526952850934755 ) ) ;
#13367=CARTESIAN_POINT ( 'NONE',  ( 13.12119116326504908, 4.807653744879115010, 5.626470997801169105 ) ) ;
#13368=CARTESIAN_POINT ( 'NONE',  ( -1.639793706121975614, -8.364901960018411131, 1.622639882261793343 ) ) ;
#13369=CARTESIAN_POINT ( 'NONE',  ( 0.9854920305337621089, -9.114917468222230923, 2.372643865078341019 ) ) ;
#13374=CARTESIAN_POINT ( 'NONE',  ( 11.59030858231679595, -21.01515356694490322, 0.9790045612916562501 ) ) ;
#13375=CARTESIAN_POINT ( 'NONE',  ( -13.15498530132288479, 5.764257716805535559, 4.666666666666618113 ) ) ;
#13377=CARTESIAN_POINT ( 'NONE',  ( -5.128441417683177406, -19.49999999999998934, 3.550687472877664952 ) ) ;
#13382=CARTESIAN_POINT ( 'NONE',  ( 6.715308582316796837, -23.02099543870833998, 3.136473910504556262 ) ) ;
#13386=CARTESIAN_POINT ( 'NONE',  ( 13.37499999998404299, -20.99999999996810729, 2.793053905886972998 ) ) ;
#13394=CARTESIAN_POINT ( 'NONE',  ( 13.84863765609603625, 3.668701632846259830, 5.985835949623216301 ) ) ;
#13397=CARTESIAN_POINT ( 'NONE',  ( 3.537356407578672535, -11.36437789272258669, 3.142965222332344766 ) ) ;
#13399=CARTESIAN_POINT ( 'NONE',  ( -13.01365964058540037, 0.1273118495903458325, 5.174178440007729307 ) ) ;
#13402=CARTESIAN_POINT ( 'NONE',  ( 12.62524871736568954, -20.23743977303344010, 4.661898514667671023 ) ) ;
#13404=CARTESIAN_POINT ( 'NONE',  ( -1.548630333695928618, -9.864917468222230923, 2.372643865078341019 ) ) ;
#13405=CARTESIAN_POINT ( 'NONE',  ( 9.152808582316795949, -21.53509896474924901, 4.479004561291659137 ) ) ;
#13407=CARTESIAN_POINT ( 'NONE',  ( 6.909691417683177406, -21.32581373872474373, 5.270995438708348857 ) ) ;
#13408=CARTESIAN_POINT ( 'NONE',  ( -8.965308582316794173, -20.22900456129164937, 4.174186261275266929 ) ) ;
#13410=CARTESIAN_POINT ( 'NONE',  ( 13.13084019862132479, 4.544930030374419339, 6.677052771569639944 ) ) ;
#13411=CARTESIAN_POINT ( 'NONE',  ( 12.64197948789552051, -18.64253586127677309, 4.770532606674187548 ) ) ;
#13420=CARTESIAN_POINT ( 'NONE',  ( 2.559937518207947793, -9.746075135043517079, 2.534737762559237773 ) ) ;
#13423=CARTESIAN_POINT ( 'NONE',  ( 12.75858672021238860, -20.53879859376904093, 3.532933081582447787 ) ) ;
#13425=CARTESIAN_POINT ( 'NONE',  ( -8.309058582316792396, -23.27327832286945153, 2.298404588716537411 ) ) ;
#13426=CARTESIAN_POINT ( 'NONE',  ( -3.486710468562268961, -9.848741751643258269, 2.003719583429115492 ) ) ;
#13428=CARTESIAN_POINT ( 'NONE',  ( -13.39169183355864590, -18.65706240528901105, 4.755687463382285429 ) ) ;
#13430=CARTESIAN_POINT ( 'NONE',  ( -6.059058582316793284, -20.72672167713054137, 4.701595411283463477 ) ) ;
#13432=CARTESIAN_POINT ( 'NONE',  ( -11.03469141768317741, -20.97900456129164581, 3.136473910504570917 ) ) ;
#13434=CARTESIAN_POINT ( 'NONE',  ( 13.39296152110871851, -19.34294318400601753, 5.489418334493660012 ) ) ;
#13435=DIRECTION ( 'NONE',  ( 0.1351665943404306014, 0.9596796555888912339, -0.2464649070825229438 ) ) ;
#13441=CARTESIAN_POINT ( 'NONE',  ( -13.37499999999998224, -20.24999999999991829, 4.333333333333343695 ) ) ;
#13445=CARTESIAN_POINT ( 'NONE',  ( 4.472191417683177406, -23.72900456129164937, 2.724438792969417378 ) ) ;
#13448=CARTESIAN_POINT ( 'NONE',  ( 1.619022621591186928, -8.364917468222230923, 2.372643865078341019 ) ) ;
#13449=CARTESIAN_POINT ( 'NONE',  ( -5.871558582316794173, -20.24999999999999289, 3.449312527122348371 ) ) ;
#13451=CARTESIAN_POINT ( 'NONE',  ( 12.62499999999998401, -20.99999999999999645, 3.666666666666654084 ) ) ;
#13453=CARTESIAN_POINT ( 'NONE',  ( 9.628441417683177406, -20.99999999999999645, 3.550687472877664952 ) ) ;
#13455=CARTESIAN_POINT ( 'NONE',  ( -5.878441417683177406, -22.99999999999999645, 3.449312527122335048 ) ) ;
#13457=CARTESIAN_POINT ( 'NONE',  ( -8.402808582316797725, -23.08622137881038938, 1.020995438708339309 ) ) ;
#13459=CARTESIAN_POINT ( 'NONE',  ( 12.62868952012632207, -19.31367923361656480, 4.748088538831167327 ) ) ;
#13460=CARTESIAN_POINT ( 'NONE',  ( -12.95145221759166354, -3.764163011652346569, 5.840524842913703552 ) ) ;
#13471=CARTESIAN_POINT ( 'NONE',  ( 13.12529397354238192, 5.014845663890297622, 3.999999999999981792 ) ) ;
#13472=CARTESIAN_POINT ( 'NONE',  ( -1.619022621591186928, -8.364917468222230923, 1.622643865078341907 ) ) ;
#13475=CARTESIAN_POINT ( 'NONE',  ( 13.10557919622060652, 4.019249409169220577, 6.007898877577752650 ) ) ;
#13477=CARTESIAN_POINT ( 'NONE',  ( 9.909691417683175629, -21.01515356694492098, 6.020995438708349745 ) ) ;
#13478=CARTESIAN_POINT ( 'NONE',  ( -12.65051119073526564, -18.96168486786632457, 5.513701926248478102 ) ) ;
#13479=CARTESIAN_POINT ( 'NONE',  ( -6.440941417683175629, -20.19639159124061933, 1.768074502826635586 ) ) ;
#13485=CARTESIAN_POINT ( 'NONE',  ( -13.41355111217617413, -19.05316883510194614, 6.247234435864091218 ) ) ;
#13486=CARTESIAN_POINT ( 'NONE',  ( 5.215308582316795949, -23.02099543870833998, 3.136473910504556262 ) ) ;
#13490=CARTESIAN_POINT ( 'NONE',  ( 13.83065313257865370, 2.760483195222930952, 5.966304699623404595 ) ) ;
#13499=CARTESIAN_POINT ( 'NONE',  ( 13.39902456816392906, -19.03675930772010361, 5.497554699623231400 ) ) ;
#13501=CARTESIAN_POINT ( 'NONE',  ( 3.722205087890566144, -11.52065056559861134, 2.433099166587254558 ) ) ;
#13503=CARTESIAN_POINT ( 'NONE',  ( -13.12529397354238192, 5.014845663890295846, 4.166666666666765551 ) ) ;
#13506=CARTESIAN_POINT ( 'NONE',  ( -13.87470602645761986, 4.985154336109792972, 3.666666666666500873 ) ) ;
#13508=CARTESIAN_POINT ( 'NONE',  ( 13.50000000000000178, 5.000000000000047962, 4.000000000000000000 ) ) ;
#13509=CARTESIAN_POINT ( 'NONE',  ( 9.340308582316795949, -22.36352608949544418, 4.520995438708343528 ) ) ;
#13510=CARTESIAN_POINT ( 'NONE',  ( 6.440941417683176518, -20.72672167713052715, 2.298404588716546293 ) ) ;
#13511=CARTESIAN_POINT ( 'NONE',  ( -10.93405858231679417, -23.20159541128345992, 4.773278322869455970 ) ) ;
#13513=CARTESIAN_POINT ( 'NONE',  ( 13.10985494974158705, 3.485174961951963191, 6.746454579156001330 ) ) ;
#13514=CARTESIAN_POINT ( 'NONE',  ( 12.62746768552656285, -19.37538188090202596, 4.723115281690125400 ) ) ;
#13517=ORIENTED_EDGE ( 'NONE', *, *, #17734, .T. ) ;
#13523=CARTESIAN_POINT ( 'NONE',  ( 2.534747216115884161, -9.671180236796224960, 2.515503256513427210 ) ) ;
#13526=CARTESIAN_POINT ( 'NONE',  ( 12.93483012243689068, -20.62499177937328199, 3.508889823513372086 ) ) ;
#13527=CARTESIAN_POINT ( 'NONE',  ( -2.596731678114175157, -9.937710376390764822, 2.583953520835782225 ) ) ;
#13528=CARTESIAN_POINT ( 'NONE',  ( -5.777808582316794173, -20.27099543870833642, 2.724438792969431589 ) ) ;
#13529=CARTESIAN_POINT ( 'NONE',  ( -3.451003380014874722, -9.682417022083358304, 1.961004070207825523 ) ) ;
#13531=CARTESIAN_POINT ( 'NONE',  ( -13.37500000000002132, -19.50000000000273559, 4.083333333315724012 ) ) ;
#13532=CARTESIAN_POINT ( 'NONE',  ( -5.684058582316794173, -20.79840458871652942, 2.226721677130544030 ) ) ;
#13533=CARTESIAN_POINT ( 'NONE',  ( 10.74655858231679595, -21.94931252712234127, 6.000000000000001776 ) ) ;
#13534=CARTESIAN_POINT ( 'NONE',  ( -12.15969141768317918, -22.36352608949543352, 2.479004561291652031 ) ) ;
#13536=CARTESIAN_POINT ( 'NONE',  ( 13.40621837757088564, -18.67347193267085714, 5.505367199623145247 ) ) ;
#13542=VERTEX_POINT ( 'NONE', #3006 ) ;
#13549=CARTESIAN_POINT ( 'NONE',  ( 1.126276606324276619, -9.114917468222230923, 2.372643865078341019 ) ) ;
#13550=CARTESIAN_POINT ( 'NONE',  ( -6.809058582316794173, -23.27327832286945153, 2.298404588716537411 ) ) ;
#13551=CARTESIAN_POINT ( 'NONE',  ( 12.62499963760179256, -21.00001830110826972, 4.442557003548452066 ) ) ;
#13552=FACE_OUTER_BOUND ( 'NONE', #17629, .T. ) ;
#13553=CARTESIAN_POINT ( 'NONE',  ( 4.753441417683176518, -21.94931252712233061, 1.749999999999998446 ) ) ;
#13555=CARTESIAN_POINT ( 'NONE',  ( -4.940941417683177406, -21.25705176302044208, 2.828734674606458555 ) ) ;
#13556=CARTESIAN_POINT ( 'NONE',  ( -4.840308582316795061, -22.98484643305508612, 6.020995438708344416 ) ) ;
#13558=CARTESIAN_POINT ( 'NONE',  ( 12.62837453896009876, -19.32958578251692572, 4.742959489302074338 ) ) ;
#13559=CARTESIAN_POINT ( 'NONE',  ( -13.08573665985359824, 3.017201322601628100, 5.986358176248492313 ) ) ;
#13563=VERTEX_POINT ( 'NONE', #1440 ) ;
#13569=CARTESIAN_POINT ( 'NONE',  ( -2.226467333542268445, -8.440126719678968215, 1.641959103308203716 ) ) ;
#13575=CARTESIAN_POINT ( 'NONE',  ( 12.62844141768317741, -19.49999999999998934, 3.550687472877664952 ) ) ;
#13576=CARTESIAN_POINT ( 'NONE',  ( -12.64323021897839006, -19.32937394158751943, 5.504219675487169283 ) ) ;
#13577=CARTESIAN_POINT ( 'NONE',  ( -9.065941417683177406, -23.73192549717336064, 1.696391591240623331 ) ) ;
#13581=CARTESIAN_POINT ( 'NONE',  ( -13.87005939078915873, 4.000499234880882327, 6.742989431566016378 ) ) ;
#13583=CARTESIAN_POINT ( 'NONE',  ( 12.43405858231679417, -23.20159541128345992, 4.773278322869455970 ) ) ;
#13587=CARTESIAN_POINT ( 'NONE',  ( 13.39170256340046095, -19.40652054827866380, 5.481861153867630065 ) ) ;
#13589=EDGE_LOOP ( 'NONE', ( #19032, #5936, #15219, #14081, #15837 ) ) ;
#13597=CARTESIAN_POINT ( 'NONE',  ( 3.607313482701580476, -10.70492285834919244, 2.223603995567122293 ) ) ;
#13599=CARTESIAN_POINT ( 'NONE',  ( -13.12529397354238192, 5.014845663890295846, 3.000000000000000000 ) ) ;
#13601=CARTESIAN_POINT ( 'NONE',  ( 11.49655858231679417, -22.05068747287764452, 1.749999999999998446 ) ) ;
#13602=CARTESIAN_POINT ( 'NONE',  ( -13.37499964066394043, -21.00001814646822496, 4.442866346476199269 ) ) ;
#13603=FACE_OUTER_BOUND ( 'NONE', #9794, .T. ) ;
#13604=CARTESIAN_POINT ( 'NONE',  ( 4.934058582316795061, -22.67126532539354855, 4.242948236979545484 ) ) ;
#13606=CARTESIAN_POINT ( 'NONE',  ( 4.847191417683178294, -21.22443879296941915, 1.770995438708345748 ) ) ;
#13607=CARTESIAN_POINT ( 'NONE',  ( -13.18405858231679417, -20.79840458871652942, 2.226721677130544030 ) ) ;
#13609=CARTESIAN_POINT ( 'NONE',  ( 13.09546733092777160, 2.758600211853326822, 6.730829579156167419 ) ) ;
#13610=CARTESIAN_POINT ( 'NONE',  ( 12.62599452815238443, -19.44977632830967806, 4.656396506304353977 ) ) ;
#13620=CARTESIAN_POINT ( 'NONE',  ( 0.2815691515810352930, -9.114917468222230923, 2.372643865078523984 ) ) ;
#13624=CARTESIAN_POINT ( 'NONE',  ( -10.55905858231679595, -20.19639159124062999, 5.231925497173373074 ) ) ;
#13625=CARTESIAN_POINT ( 'NONE',  ( -2.532303758294933704, -8.551221675625164664, 1.670490507339845054 ) ) ;
#13627=CARTESIAN_POINT ( 'NONE',  ( -13.39888564296547635, -18.29377503024027263, 4.763499963382565205 ) ) ;
#13628=CARTESIAN_POINT ( 'NONE',  ( -9.246558582316794173, -21.94931252712234482, 5.250000000000000888 ) ) ;
#13630=CARTESIAN_POINT ( 'NONE',  ( 9.534691417683177406, -19.47900456129164581, 2.515153566944927199 ) ) ;
#13631=CARTESIAN_POINT ( 'NONE',  ( -8.972191417683177406, -22.97900456129165292, 3.035098964749240125 ) ) ;
#13633=CARTESIAN_POINT ( 'NONE',  ( 13.84863765609603625, 3.668701632846259830, 5.985835949623216301 ) ) ;
#13640=CARTESIAN_POINT ( 'NONE',  ( -13.37499979530394967, -20.25001033714808329, 4.458488164327452097 ) ) ;
#13646=CARTESIAN_POINT ( 'NONE',  ( 1.824488249492779879, -9.124319963227819130, 2.375058613629473570 ) ) ;
#13648=CARTESIAN_POINT ( 'NONE',  ( 12.64183575740756993, -20.14979425091403087, 6.022201559249563907 ) ) ;
#13652=CARTESIAN_POINT ( 'NONE',  ( 5.690941417683176518, -23.27327832286946219, 4.701595411283453707 ) ) ;
#13654=CARTESIAN_POINT ( 'NONE',  ( -9.440941417683177406, -21.25705176302044208, 2.828734674606458555 ) ) ;
#13655=ADVANCED_FACE ( 'NONE', ( #17634 ), #1944, .F. ) ;
#13656=CARTESIAN_POINT ( 'NONE',  ( -11.12844141768317741, -19.49999999999998934, 3.550687472877664952 ) ) ;
#13658=CARTESIAN_POINT ( 'NONE',  ( 12.63598464672302590, -18.94527534048458151, 4.764022190007618285 ) ) ;
#13671=CARTESIAN_POINT ( 'NONE',  ( -2.309828811027716977, -9.292785183284841821, 1.668323847571005603 ) ) ;
#13676=CARTESIAN_POINT ( 'NONE',  ( 10.19094141768317741, -23.80360840875937001, 5.231925497173365081 ) ) ;
#13677=CARTESIAN_POINT ( 'NONE',  ( -12.64571531779736979, -19.20387645123237164, 5.508493592915143289 ) ) ;
#13678=CARTESIAN_POINT ( 'NONE',  ( -5.409691417683178294, -21.01515356694492098, 6.020995438708349745 ) ) ;
#13680=CARTESIAN_POINT ( 'NONE',  ( 11.49655858231679417, -22.05068747287764452, 1.749999999999998446 ) ) ;
#13682=CARTESIAN_POINT ( 'NONE',  ( -13.85716935893578317, 3.349552626256921517, 6.729005269197402939 ) ) ;
#13685=CARTESIAN_POINT ( 'NONE',  ( 10.93405858231679417, -23.20159541128345992, 4.773278322869455970 ) ) ;
#13689=CARTESIAN_POINT ( 'NONE',  ( 13.87470623115321899, 4.985164673244912414, 4.958488177337359026 ) ) ;
#13697=CARTESIAN_POINT ( 'NONE',  ( -11.02780858231679595, -23.72900456129165647, 4.275561207030568411 ) ) ;
#13701=CARTESIAN_POINT ( 'NONE',  ( 0.5631383031621635116, -8.364917468222230923, 1.622643865078341907 ) ) ;
#13705=CARTESIAN_POINT ( 'NONE',  ( -13.09560264576187905, 4.265433610975056133, 4.833333333333343695 ) ) ;
#13706=CARTESIAN_POINT ( 'NONE',  ( 10.37155858231679417, -20.24999999999999289, 3.449312527122348371 ) ) ;
#13707=CARTESIAN_POINT ( 'NONE',  ( -13.85716935893578317, 3.349552626256921517, 6.729005269197402939 ) ) ;
#13709=CARTESIAN_POINT ( 'NONE',  ( 13.18405858231679417, -20.79840458871652942, 2.226721677130544030 ) ) ;
#13711=CARTESIAN_POINT ( 'NONE',  ( 4.753441417683176518, -21.94931252712233061, 1.749999999999998446 ) ) ;
#13712=CARTESIAN_POINT ( 'NONE',  ( -11.40280858231679417, -22.77556120703056308, 1.770995438708339975 ) ) ;
#13714=CARTESIAN_POINT ( 'NONE',  ( 12.63598464672302590, -18.94527534048458151, 4.764022190007618285 ) ) ;
#13723=CARTESIAN_POINT ( 'NONE',  ( -12.62500000000001954, -20.24999999999506173, 3.850307403176420618 ) ) ;
#13724=CARTESIAN_POINT ( 'NONE',  ( -2.817596665886821672, -11.50588678273290988, 2.986692549455723267 ) ) ;
#13725=CARTESIAN_POINT ( 'NONE',  ( -13.85593616229004610, 4.037276195647738319, 5.992122970672676630 ) ) ;
#13728=CARTESIAN_POINT ( 'NONE',  ( 1.853238653218509890, -9.965882697426144077, 2.398573752920997837 ) ) ;
#13733=CARTESIAN_POINT ( 'NONE',  ( -1.548630333695928396, -9.114917468222230923, 2.372643865078341019 ) ) ;
#13734=CARTESIAN_POINT ( 'NONE',  ( -8.496558582316795949, -22.05068747287764452, 0.9999999999999978906 ) ) ;
#13735=CARTESIAN_POINT ( 'NONE',  ( -1.337453470010121714, -8.364917468222230923, 1.622643865078341907 ) ) ;
#13737=CARTESIAN_POINT ( 'NONE',  ( -13.38210008768272630, -19.14144557202113006, 4.745270796715706396 ) ) ;
#13740=CARTESIAN_POINT ( 'NONE',  ( 5.309058582316795949, -23.80360840875935935, 1.768074502826626260 ) ) ;
#13741=CARTESIAN_POINT ( 'NONE',  ( -12.53469141768317741, -20.97900456129164581, 3.136473910504570917 ) ) ;
#13744=CARTESIAN_POINT ( 'NONE',  ( 13.37503071710846925, -20.24844878602346299, 4.564052989354591361 ) ) ;
#13751=CARTESIAN_POINT ( 'NONE',  ( -13.87454419214980739, 4.976981703567351367, 5.131312659523921127 ) ) ;
#13758=CARTESIAN_POINT ( 'NONE',  ( 1.932703420524435112, -8.381852853175612239, 2.376993210252662969 ) ) ;
#13760=CARTESIAN_POINT ( 'NONE',  ( 12.66204031416134335, -19.12946413485185104, 6.260126454156002218 ) ) ;
#13764=CARTESIAN_POINT ( 'NONE',  ( 4.659691417683178294, -22.67418626127524917, 1.729004561291651809 ) ) ;
#13766=CARTESIAN_POINT ( 'NONE',  ( -9.715308582316795949, -23.02099543870833998, 3.136473910504556262 ) ) ;
#13768=CARTESIAN_POINT ( 'NONE',  ( -12.34719141768317741, -20.91377862118959285, 1.020995438708345082 ) ) ;
#13770=CARTESIAN_POINT ( 'NONE',  ( 13.11514659413808737, 4.502403003978772134, 5.887634658581065494 ) ) ;
#13771=CARTESIAN_POINT ( 'NONE',  ( -13.12529397354238192, 5.014845663890295846, 4.916666666666650087 ) ) ;
#13776=CARTESIAN_POINT ( 'NONE',  ( 1.863950040896528604, -9.995453039732266731, 2.406168007552154098 ) ) ;
#13782=CARTESIAN_POINT ( 'NONE',  ( -1.513434189748285918, -9.864917468222230923, 1.622643865078341907 ) ) ;
#13786=CARTESIAN_POINT ( 'NONE',  ( 12.06594141768317741, -23.73192549717336064, 1.696391591240623331 ) ) ;
#13787=CARTESIAN_POINT ( 'NONE',  ( -12.63819864697926754, -19.58346832754827105, 5.450273968536036406 ) ) ;
#13788=CARTESIAN_POINT ( 'NONE',  ( -4.940941417683177406, -20.19639159124061933, 1.768074502826635586 ) ) ;
#13792=CARTESIAN_POINT ( 'NONE',  ( -13.60059015675642513, -9.607697083824668027, 6.450359435862663027 ) ) ;
#13794=CARTESIAN_POINT ( 'NONE',  ( 6.059058582316795949, -21.25705176302045274, 4.171265325393551215 ) ) ;
#13798=CARTESIAN_POINT ( 'NONE',  ( 13.48548920624593883, -15.42029508461213716, 6.325359435864005064 ) ) ;
#13803=CARTESIAN_POINT ( 'NONE',  ( -8.777808582316792396, -20.27099543870833642, 2.724438792969431589 ) ) ;
#13807=CARTESIAN_POINT ( 'NONE',  ( 2.887553741010006281, -10.84643174835951207, 2.067331322690557638 ) ) ;
#13810=CARTESIAN_POINT ( 'NONE',  ( -13.09455366754861139, 4.212460211200554916, 5.160171780694988719 ) ) ;
#13812=CARTESIAN_POINT ( 'NONE',  ( -13.48548920624593883, -15.42029508461213716, 6.325359435864005064 ) ) ;
#13814=CARTESIAN_POINT ( 'NONE',  ( 10.09030858231679595, -21.32581373872472597, 1.729004561291657582 ) ) ;
#13816=CARTESIAN_POINT ( 'NONE',  ( 4.190941417683176518, -23.27327832286946219, 4.701595411283453707 ) ) ;
#13817=CARTESIAN_POINT ( 'NONE',  ( -8.496558582316794173, -22.05068747287764452, 1.749999999999998446 ) ) ;
#13819=CARTESIAN_POINT ( 'NONE',  ( 13.53317008522746434, -11.51241069598931510, 4.909333296715523431 ) ) ;
#13824=CARTESIAN_POINT ( 'NONE',  ( -12.65650603190776025, -18.65894538865861563, 5.520212342915047365 ) ) ;
#13825=CARTESIAN_POINT ( 'NONE',  ( -2.583953725994688533, -9.847075946378776479, 2.560676788604062004 ) ) ;
#13826=CARTESIAN_POINT ( 'NONE',  ( -13.87470586348985258, 4.985146106231644225, 5.033049509202228933 ) ) ;
#13829=CARTESIAN_POINT ( 'NONE',  ( -12.62499999999998224, -20.24999999999998934, 4.166666666666636765 ) ) ;
#13831=CARTESIAN_POINT ( 'NONE',  ( -13.12499999999999645, 5.000000000000047073, 3.999999999999996447 ) ) ;
#13833=CARTESIAN_POINT ( 'NONE',  ( -9.059058582316795949, -20.19639159124062999, 5.231925497173373074 ) ) ;
#13834=CARTESIAN_POINT ( 'NONE',  ( -2.780192134145684779, -10.08406280675441735, 1.871539748636713130 ) ) ;
#13838=CARTESIAN_POINT ( 'NONE',  ( -13.84497512400090891, 4.233743762047977199, 5.032110966142367303 ) ) ;
#13840=CARTESIAN_POINT ( 'NONE',  ( 5.121558582316795061, -24.50000000000000000, 3.550687472877651629 ) ) ;
#13841=CARTESIAN_POINT ( 'NONE',  ( -8.690941417683177406, -22.74294823697955081, 4.171265325393542334 ) ) ;
#13843=CARTESIAN_POINT ( 'NONE',  ( 13.37499964066394043, -21.00001814646822496, 4.442866346476199269 ) ) ;
#13850=CARTESIAN_POINT ( 'NONE',  ( -13.77789853026076550, 0.09637577819625635367, 5.909013032956687006 ) ) ;
#13851=CARTESIAN_POINT ( 'NONE',  ( 2.203959450683124377, -9.262433282444222371, 2.410528873095051594 ) ) ;
#13858=CARTESIAN_POINT ( 'NONE',  ( 3.462011766956747394, -14.92507028461178287, 3.114807177791267812 ) ) ;
#13859=DIRECTION ( 'NONE',  ( 0.1351665943404306014, -0.9596796555888911229, 0.2464649070825229160 ) ) ;
#13861=CARTESIAN_POINT ( 'NONE',  ( 13.10012427866737639, 3.743776072700027324, 6.001983176248468332 ) ) ;
#13867=CARTESIAN_POINT ( 'NONE',  ( 7.284691417683176518, -23.02099543870834353, 3.863526089495429972 ) ) ;
#13868=CARTESIAN_POINT ( 'NONE',  ( -12.69247507894198712, -16.84250851341299082, 5.559274842915185033 ) ) ;
#13869=CARTESIAN_POINT ( 'NONE',  ( -8.684058582316795949, -21.32873467460644079, 2.757051763020455404 ) ) ;
#13870=CARTESIAN_POINT ( 'NONE',  ( -9.909691417683175629, -21.01515356694492098, 6.020995438708349745 ) ) ;
#13872=CARTESIAN_POINT ( 'NONE',  ( 13.12529397354238192, 5.014845663890295846, 3.666666666666500873 ) ) ;
#13873=CARTESIAN_POINT ( 'NONE',  ( -13.10624331898488037, 4.052787608736739600, 6.006964772046813117 ) ) ;
#13877=CARTESIAN_POINT ( 'NONE',  ( 0.000000000000000000, -9.864917468222230923, 2.372643865078341019 ) ) ;
#13883=CARTESIAN_POINT ( 'NONE',  ( -2.022757268986824730, -10.07035769906783784, 1.675405020440470238 ) ) ;
#13887=CARTESIAN_POINT ( 'NONE',  ( 5.965308582316795949, -19.47900456129164937, 4.484846433055089676 ) ) ;
#13888=CARTESIAN_POINT ( 'NONE',  ( -12.62888984277510218, -20.05356293986039873, 5.111704976569332537 ) ) ;
#13889=CARTESIAN_POINT ( 'NONE',  ( -8.409691417683177406, -21.32581373872474373, 5.270995438708348857 ) ) ;
#13893=CARTESIAN_POINT ( 'NONE',  ( -13.87824226375436965, 4.413734319597230282, 6.694665752684481497 ) ) ;
#13896=CARTESIAN_POINT ( 'NONE',  ( 9.715308582316794173, -23.77099543870833998, 2.825813738724734847 ) ) ;
#13900=CARTESIAN_POINT ( 'NONE',  ( 13.37543017851028893, -20.97827598523083026, 4.780017688621249761 ) ) ;
#13905=CARTESIAN_POINT ( 'NONE',  ( -12.99655858231679417, -22.05068747287764452, 1.749999999999998446 ) ) ;
#13908=CARTESIAN_POINT ( 'NONE',  ( 2.012076196476103362, -9.160103213191565175, 1.634248467062433541 ) ) ;
#13910=CARTESIAN_POINT ( 'NONE',  ( -13.09553549038190567, 4.262042264285192950, 5.042530537310905281 ) ) ;
#13911=CARTESIAN_POINT ( 'NONE',  ( 12.05905858231679417, -20.72672167713054137, 4.701595411283463477 ) ) ;
#13912=CARTESIAN_POINT ( 'NONE',  ( -13.39169349927020569, -20.15697828685464188, 6.009339318877812808 ) ) ;
#13914=CARTESIAN_POINT ( 'NONE',  ( 4.746558582316795061, -21.94931252712234127, 4.499999999999999112 ) ) ;
#13916=CARTESIAN_POINT ( 'NONE',  ( 9.909691417683175629, -21.63647391050456648, 4.520995438708348857 ) ) ;
#13917=CARTESIAN_POINT ( 'NONE',  ( -7.277808582316794173, -20.27099543870833642, 2.724438792969431589 ) ) ;
#13919=CARTESIAN_POINT ( 'NONE',  ( 13.39888564296547635, -18.29377503024027263, 4.763499963382565205 ) ) ;
#13921=CARTESIAN_POINT ( 'NONE',  ( -2.747777887823422471, -9.906471667804277459, 1.825930796414880763 ) ) ;
#13922=EDGE_LOOP ( 'NONE', ( #12591, #2804, #14044, #7843, #5472, #9577 ) ) ;
#13926=CARTESIAN_POINT ( 'NONE',  ( -13.10557919622060652, 4.019249409169220577, 6.007898877577752650 ) ) ;
#13928=CARTESIAN_POINT ( 'NONE',  ( -13.81626551376501588, 2.033908445126689557, 5.950679699622869911 ) ) ;
#13934=CARTESIAN_POINT ( 'NONE',  ( -10.37155858231679595, -19.49999999999998934, 3.449312527122348371 ) ) ;
#13935=CARTESIAN_POINT ( 'NONE',  ( -1.819865260185086875, -9.122006307963404836, 1.624464420737683046 ) ) ;
#13938=CARTESIAN_POINT ( 'NONE',  ( -13.83973345681288158, 3.969039569021246550, 5.242263935944164288 ) ) ;
#13940=CARTESIAN_POINT ( 'NONE',  ( 12.34719141768317741, -20.91377862118959285, 1.020995438708345082 ) ) ;
#13941=CARTESIAN_POINT ( 'NONE',  ( -3.974842109207560537, -21.92432777746334693, 4.506404853634142782 ) ) ;
#13943=CARTESIAN_POINT ( 'NONE',  ( 13.85980676119184629, 4.232741440188380722, 5.965367510457697975 ) ) ;
#13959=CARTESIAN_POINT ( 'NONE',  ( 2.309828811027716977, -9.292785183284841821, 1.668323847571005603 ) ) ;
#13966=CARTESIAN_POINT ( 'NONE',  ( 4.565941417683176518, -22.67126532539353789, 2.757051763020445634 ) ) ;
#13967=CARTESIAN_POINT ( 'NONE',  ( -13.12529397354238192, 5.014845663890295846, 4.583333333333296622 ) ) ;
#13968=CARTESIAN_POINT ( 'NONE',  ( -12.24655858231679595, -21.94931252712234127, 4.499999999999999112 ) ) ;
#13969=CARTESIAN_POINT ( 'NONE',  ( -9.253441417683177406, -21.94931252712233061, 0.9999999999999978906 ) ) ;
#13972=CARTESIAN_POINT ( 'NONE',  ( 13.09560269887985307, 4.265436293439658577, 4.973800642626965640 ) ) ;
#13978=CARTESIAN_POINT ( 'NONE',  ( 1.853238653218509890, -9.965882697426144077, 2.398573752920997837 ) ) ;
#13983=CARTESIAN_POINT ( 'NONE',  ( -1.963707630584672570, -9.980492102769451535, 1.652325740065381909 ) ) ;
#13988=CARTESIAN_POINT ( 'NONE',  ( 8.597191417683177406, -23.08622137881040359, 5.979004561291654696 ) ) ;
#13989=CARTESIAN_POINT ( 'NONE',  ( -13.12529397354238192, 5.014845663890295846, 3.666666666666500873 ) ) ;
#13990=CARTESIAN_POINT ( 'NONE',  ( -8.222191417683175629, -20.27099543870833998, 4.275561207030583510 ) ) ;
#13992=CARTESIAN_POINT ( 'NONE',  ( 8.215308582316792396, -23.77099543870833998, 2.825813738724734847 ) ) ;
#13994=CARTESIAN_POINT ( 'NONE',  ( -12.63178515739782348, -20.65734955141111584, 5.567013446834313761 ) ) ;
#13998=CARTESIAN_POINT ( 'NONE',  ( 7.371558582316794173, -20.24999999999999289, 3.449312527122348371 ) ) ;
#14004=ORIENTED_EDGE ( 'NONE', *, *, #20615, .T. ) ;
#14005=CARTESIAN_POINT ( 'NONE',  ( 13.37671366598624800, -20.91345986769124465, 5.053911344471881506 ) ) ;
#14012=CARTESIAN_POINT ( 'NONE',  ( 2.693754455098655409, -10.04853567022903782, 2.237415670251142519 ) ) ;
#14013=CARTESIAN_POINT ( 'NONE',  ( 0.000000000000000000, -8.364917468222230923, 1.622643865078341241 ) ) ;
#14017=CARTESIAN_POINT ( 'NONE',  ( -13.08080186171710224, 3.517994016715657146, 5.247095106674282583 ) ) ;
#14019=CARTESIAN_POINT ( 'NONE',  ( 6.152808582316793284, -21.22443879296942626, 5.229004561291659137 ) ) ;
#14020=CARTESIAN_POINT ( 'NONE',  ( -12.67103257592000176, -18.67535491604046172, 6.269892079155907183 ) ) ;
#14023=CARTESIAN_POINT ( 'NONE',  ( 4.840308582316795061, -22.36352608949544418, 4.520995438708343528 ) ) ;
#14024=CARTESIAN_POINT ( 'NONE',  ( 9.347191417683177406, -21.53509896474923835, 2.520995438708346192 ) ) ;
#14025=CARTESIAN_POINT ( 'NONE',  ( -6.340308582316793284, -22.67418626127525982, 5.270995438708342640 ) ) ;
#14027=CARTESIAN_POINT ( 'NONE',  ( 13.38929389708972195, -18.77815819697223887, 4.753083296715700179 ) ) ;
#14028=CARTESIAN_POINT ( 'NONE',  ( -0.5631383031621635116, -9.114917468222230923, 1.622643865078341463 ) ) ;
#14030=( BOUNDED_CURVE ( )  B_SPLINE_CURVE ( 3, ( #17359, #7849, #15791, #5870 ),
 .UNSPECIFIED., .F., .F. ) 
 B_SPLINE_CURVE_WITH_KNOTS ( ( 4, 4 ),
 ( 0.001187255941418635012, 0.002344578398797381343 ),
 .UNSPECIFIED. ) 
 CURVE ( )  GEOMETRIC_REPRESENTATION_ITEM ( )  RATIONAL_B_SPLINE_CURVE ( ( 0.9619191252709787809, 0.3335846922424358096, 0.3462783171521095493, 1.000000000000000000 ) ) 
 REPRESENTATION_ITEM ( '' )  );
#14034=CARTESIAN_POINT ( 'NONE',  ( -12.69247507894198712, -16.84250851341299082, 5.559274842915185033 ) ) ;
#14035=CARTESIAN_POINT ( 'NONE',  ( -1.717920576997000737, -9.114924032904250240, 2.372645551019823884 ) ) ;
#14036=CARTESIAN_POINT ( 'NONE',  ( -13.86470821076586368, 4.480264643675554659, 5.874551681240599343 ) ) ;
#14042=CARTESIAN_POINT ( 'NONE',  ( -11.30905858231679595, -23.80360840875935935, 1.768074502826626260 ) ) ;
#14043=CARTESIAN_POINT ( 'NONE',  ( -3.347120161770001268, -14.10934257735911146, 2.905312006771028077 ) ) ;
#14044=ORIENTED_EDGE ( 'NONE', *, *, #11822, .F. ) ;
#14045=CARTESIAN_POINT ( 'NONE',  ( -13.84090061271218985, 4.027980941966571748, 5.240332426532912535 ) ) ;
#14048=CARTESIAN_POINT ( 'NONE',  ( 9.815941417683177406, -20.26807450282663225, 5.303608408759377113 ) ) ;
#14049=CARTESIAN_POINT ( 'NONE',  ( -4.003441417683175629, -22.05068747287766229, 4.499999999999999112 ) ) ;
#14052=CARTESIAN_POINT ( 'NONE',  ( 13.41115317570721110, -19.17426462678482579, 6.244630269197427808 ) ) ;
#14053=CARTESIAN_POINT ( 'NONE',  ( 12.62499999999998224, -20.24999999999991829, 4.333333333333343695 ) ) ;
#14058=CARTESIAN_POINT ( 'NONE',  ( -13.40621837757088564, -18.67347193267085714, 5.505367199623145247 ) ) ;
#14059=CARTESIAN_POINT ( 'NONE',  ( 1.126276606324276619, -9.114917468222230923, 2.372643865078341019 ) ) ;
#14061=CARTESIAN_POINT ( 'NONE',  ( -3.944195004867013132, -21.63820656525943775, 5.112513974992745958 ) ) ;
#14066=CARTESIAN_POINT ( 'NONE',  ( 2.682825141213236009, -9.727160171598653093, 1.779880022082258373 ) ) ;
#14068=CARTESIAN_POINT ( 'NONE',  ( 13.12529397354238192, 5.014845663890295846, 4.833333333333344584 ) ) ;
#14073=CARTESIAN_POINT ( 'NONE',  ( 12.90280858231679595, -22.46490103525074034, 2.520995438708341307 ) ) ;
#14074=CARTESIAN_POINT ( 'NONE',  ( -12.62499999998404299, -19.49999999996810729, 2.793053905886972998 ) ) ;
#14075=CARTESIAN_POINT ( 'NONE',  ( -12.71530858231679417, -23.02099543870833998, 3.136473910504556262 ) ) ;
#14076=CARTESIAN_POINT ( 'NONE',  ( -6.440941417683175629, -20.19639159124061933, 1.768074502826635586 ) ) ;
#14079=CARTESIAN_POINT ( 'NONE',  ( 13.09106898171683930, 4.036483576700608644, 5.256123545019964816 ) ) ;
#14081=ORIENTED_EDGE ( 'NONE', *, *, #5397, .F. ) ;
#14086=CARTESIAN_POINT ( 'NONE',  ( 2.659620708751979645, -10.38426118526329489, 2.698636689302993830 ) ) ;
#14090=CARTESIAN_POINT ( 'NONE',  ( -1.126276606324276619, -9.864917468222230923, 1.622643865078341907 ) ) ;
#14096=CARTESIAN_POINT ( 'NONE',  ( 12.53469141768317741, -20.22900456129164581, 2.825813738724747726 ) ) ;
#14098=CARTESIAN_POINT ( 'NONE',  ( -12.25344141768317741, -21.94931252712233061, 1.749999999999998446 ) ) ;
#14100=CARTESIAN_POINT ( 'NONE',  ( 5.871558582316794173, -20.24999999999999289, 3.449312527122348371 ) ) ;
#14102=CARTESIAN_POINT ( 'NONE',  ( -13.90439735423812273, 5.734566389025032684, 4.583333333333295734 ) ) ;
#14105=CARTESIAN_POINT ( 'NONE',  ( 5.402808582316794173, -22.77556120703056308, 1.770995438708339975 ) ) ;
#14115=CARTESIAN_POINT ( 'NONE',  ( -11.40280858231679417, -22.77556120703056308, 1.770995438708339975 ) ) ;
#14118=CARTESIAN_POINT ( 'NONE',  ( 1.337453470010121714, -8.364917468222230923, 1.622643865078341907 ) ) ;
#14122=CARTESIAN_POINT ( 'NONE',  ( -13.09560264576187905, 4.265433610975056133, 4.166666666666765551 ) ) ;
#14123=CARTESIAN_POINT ( 'NONE',  ( 5.309058582316794173, -23.27327832286945153, 2.298404588716537411 ) ) ;
#14124=CARTESIAN_POINT ( 'NONE',  ( -12.62499999999998401, -20.99999999999998934, 2.439580858552613751 ) ) ;
#14126=CARTESIAN_POINT ( 'NONE',  ( -13.12529397354238192, 5.014845663890297622, 3.999999999999981792 ) ) ;
#14127=CARTESIAN_POINT ( 'NONE',  ( 7.652808582316795061, -21.22443879296942626, 5.229004561291659137 ) ) ;
#14128=CARTESIAN_POINT ( 'NONE',  ( 8.409691417683177406, -21.63647391050456648, 4.520995438708348857 ) ) ;
#14129=CARTESIAN_POINT ( 'NONE',  ( -5.215308582316793284, -23.77099543870833998, 2.825813738724734847 ) ) ;
#14131=CARTESIAN_POINT ( 'NONE',  ( 13.37500000000002132, -19.49999999999450040, 3.833333333368183382 ) ) ;
#14132=CARTESIAN_POINT ( 'NONE',  ( -1.513434189748285696, -9.114917468222230923, 1.622643865078341463 ) ) ;
#14137=CARTESIAN_POINT ( 'NONE',  ( -12.63819864697926754, -19.58346832754827105, 5.450273968536036406 ) ) ;
#14138=CARTESIAN_POINT ( 'NONE',  ( -3.365018999794965548, -10.14078633184679923, 2.828722465802024910 ) ) ;
#14139=CARTESIAN_POINT ( 'NONE',  ( -13.75871503850933841, -0.8723905552644914962, 5.888179699623941943 ) ) ;
#14145=CARTESIAN_POINT ( 'NONE',  ( 12.92761177809936513, -5.718105205959081339, 6.548537912490751900 ) ) ;
#14146=CARTESIAN_POINT ( 'NONE',  ( -11.59719141768317741, -23.08622137881040359, 5.979004561291654696 ) ) ;
#14147=CARTESIAN_POINT ( 'NONE',  ( -1.862510824048270619, -9.990417728039201251, 2.404874838918925395 ) ) ;
#14148=ORIENTED_EDGE ( 'NONE', *, *, #19539, .F. ) ;
#14149=CARTESIAN_POINT ( 'NONE',  ( -13.37561105820882013, -20.21914156045197686, 4.753815841436231260 ) ) ;
#14151=CARTESIAN_POINT ( 'NONE',  ( 7.190941417683177406, -23.80360840875937001, 5.231925497173365081 ) ) ;
#14152=CARTESIAN_POINT ( 'NONE',  ( -12.80905858231679417, -22.74294823697954016, 2.828734674606448785 ) ) ;
#14154=CARTESIAN_POINT ( 'NONE',  ( 13.87470586348985258, 4.985146106231644225, 5.033049509202228933 ) ) ;
#14155=CARTESIAN_POINT ( 'NONE',  ( 12.62888984277510218, -20.05356293986039873, 5.111704976569332537 ) ) ;
#14164=CARTESIAN_POINT ( 'NONE',  ( 2.367358971471363649, -9.400572650371021410, 2.446005822389718087 ) ) ;
#14166=CARTESIAN_POINT ( 'NONE',  ( 1.513434189748285696, -9.114917468222230923, 1.622643865078341463 ) ) ;
#14172=CARTESIAN_POINT ( 'NONE',  ( 7.097191417683176518, -22.46490103525075810, 4.479004561291653808 ) ) ;
#14173=CARTESIAN_POINT ( 'NONE',  ( -13.10821839766814279, 4.152529082241303904, 5.997503362667785609 ) ) ;
#14174=CARTESIAN_POINT ( 'NONE',  ( -8.309058582316795949, -22.74294823697954016, 2.828734674606448785 ) ) ;
#14175=CARTESIAN_POINT ( 'NONE',  ( -12.53469141768317741, -20.22900456129164581, 2.825813738724747726 ) ) ;
#14177=CARTESIAN_POINT ( 'NONE',  ( 13.09560264576187905, 4.265433610975056133, 4.833333333333343695 ) ) ;
#14182=CARTESIAN_POINT ( 'NONE',  ( 0.9854920305337622199, -9.864917468222230923, 2.372643865078341019 ) ) ;
#14185=CARTESIAN_POINT ( 'NONE',  ( 7.847191417683176518, -21.22443879296941915, 1.770995438708345748 ) ) ;
#14188=CARTESIAN_POINT ( 'NONE',  ( -1.862510824048270619, -9.990417728039201251, 2.404874838918925395 ) ) ;
#14190=CARTESIAN_POINT ( 'NONE',  ( -11.77780858231679773, -20.27099543870833642, 2.724438792969431589 ) ) ;
#14192=CARTESIAN_POINT ( 'NONE',  ( 7.472191417683177406, -24.47900456129165292, 2.413778621189595963 ) ) ;
#14194=CARTESIAN_POINT ( 'NONE',  ( -6.815941417683176518, -20.79840458871654363, 4.773278322869464851 ) ) ;
#14196=CARTESIAN_POINT ( 'NONE',  ( 6.621558582316794173, -23.74999999999999645, 3.550687472877651629 ) ) ;
#14198=CARTESIAN_POINT ( 'NONE',  ( -12.65679946139692902, -19.39412719945235253, 6.251687395662565372 ) ) ;
#14200=CARTESIAN_POINT ( 'NONE',  ( 7.652808582316795061, -21.22443879296942626, 5.229004561291659137 ) ) ;
#14208=CARTESIAN_POINT ( 'NONE',  ( -5.871558582316794173, -20.24999999999999289, 3.449312527122348371 ) ) ;
#14212=CARTESIAN_POINT ( 'NONE',  ( 2.512468814886674284, -13.43512376012158782, 2.539544162874482591 ) ) ;
#14215=CARTESIAN_POINT ( 'NONE',  ( -13.84311479963346869, 4.139797381492562600, 5.195993353439945395 ) ) ;
#14217=CARTESIAN_POINT ( 'NONE',  ( 4.746558582316793284, -21.94931252712234482, 5.250000000000000888 ) ) ;
#14218=CARTESIAN_POINT ( 'NONE',  ( -12.62927505847832776, -20.78410954684871825, 5.373974324164845662 ) ) ;
#14219=CARTESIAN_POINT ( 'NONE',  ( -13.12529397354238192, 5.014845663890297622, 3.999999999999981792 ) ) ;
#14220=CARTESIAN_POINT ( 'NONE',  ( 6.059058582316793284, -20.72672167713054137, 4.701595411283463477 ) ) ;
#14221=CARTESIAN_POINT ( 'NONE',  ( 4.284691417683177406, -23.02099543870834353, 3.863526089495429972 ) ) ;
#14222=CARTESIAN_POINT ( 'NONE',  ( -12.25344141768317741, -21.94931252712233061, 1.749999999999998446 ) ) ;
#14224=CARTESIAN_POINT ( 'NONE',  ( 13.64827103573800571, -5.699812695207630675, 5.034333296717131034 ) ) ;
#14231=CARTESIAN_POINT ( 'NONE',  ( -3.951988298270009636, -13.15210598010094323, 2.852089508627633219 ) ) ;
#14232=CARTESIAN_POINT ( 'NONE',  ( 1.407845757905374695, -9.114917468222230923, 2.372643865078341019 ) ) ;
#14233=CYLINDRICAL_SURFACE ( 'NONE', #7394, 0.3749999999999997224 ) ;
#14235=CARTESIAN_POINT ( 'NONE',  ( 10.84030858231679240, -22.67418626127525982, 5.270995438708342640 ) ) ;
#14237=CARTESIAN_POINT ( 'NONE',  ( 12.96597876160390683, -3.780572539034193102, 6.590204579154564257 ) ) ;
#14239=CARTESIAN_POINT ( 'NONE',  ( -10.56594141768317741, -23.73192549717336064, 1.696391591240623331 ) ) ;
#14240=CARTESIAN_POINT ( 'NONE',  ( -0.9854920305337622199, -9.864917468222230923, 1.622643865078341907 ) ) ;
#14241=ORIENTED_EDGE ( 'NONE', *, *, #9614, .F. ) ;
#14242=CARTESIAN_POINT ( 'NONE',  ( -13.84501469867711698, 4.235742283194553259, 2.999999999999999556 ) ) ;
#14244=CARTESIAN_POINT ( 'NONE',  ( 12.44094141768317741, -20.72672167713052715, 2.298404588716546293 ) ) ;
#14245=CARTESIAN_POINT ( 'NONE',  ( -10.84030858231679595, -22.36352608949544418, 4.520995438708343528 ) ) ;
#14247=CARTESIAN_POINT ( 'NONE',  ( 13.87470602645761986, 4.985154336109792972, 4.666666666666619889 ) ) ;
#14248=CARTESIAN_POINT ( 'NONE',  ( 12.64195242771744709, -19.39390240027112000, 5.496549442168085164 ) ) ;
#14258=CARTESIAN_POINT ( 'NONE',  ( -4.315753587183824180, -21.65797192216093947, 4.831781436261117335 ) ) ;
#14259=CARTESIAN_POINT ( 'NONE',  ( 2.731427961995660958, -10.89409100229510052, 2.829571171190552015 ) ) ;
#14261=CARTESIAN_POINT ( 'NONE',  ( 1.548630333695928618, -8.364917468222230923, 1.622643865078341907 ) ) ;
#14266=DIRECTION ( 'NONE',  ( 0.000000000000000000, 0.2487476929738665354, 0.9685683172808094987 ) ) ;
#14268=CARTESIAN_POINT ( 'NONE',  ( -11.96530858231679595, -20.22900456129164937, 4.174186261275266929 ) ) ;
#14270=CARTESIAN_POINT ( 'NONE',  ( 6.815941417683177406, -21.32873467460645145, 4.242948236979555254 ) ) ;
#14271=CARTESIAN_POINT ( 'NONE',  ( -13.02818618459764188, 0.1109023222084986743, 5.923858176248589125 ) ) ;
#14272=CARTESIAN_POINT ( 'NONE',  ( -12.62155858231679417, -23.74999999999999645, 3.550687472877651629 ) ) ;
#14273=CARTESIAN_POINT ( 'NONE',  ( -11.87844141768317563, -23.74999999999999645, 3.449312527122335492 ) ) ;
#14275=CARTESIAN_POINT ( 'NONE',  ( 13.37500000000002132, -19.50000000000273559, 4.083333333315724012 ) ) ;
#14283=CARTESIAN_POINT ( 'NONE',  ( 11.22219141768317741, -20.27099543870833998, 4.275561207030583510 ) ) ;
#14285=CARTESIAN_POINT ( 'NONE',  ( -1.716273078461125090, -9.866787073280026021, 2.373124017006284170 ) ) ;
#14287=CARTESIAN_POINT ( 'NONE',  ( -13.27780858231679595, -20.27099543870833642, 2.724438792969431589 ) ) ;
#14291=CARTESIAN_POINT ( 'NONE',  ( 8.690941417683177406, -23.80360840875937001, 5.231925497173365081 ) ) ;
#14292=CARTESIAN_POINT ( 'NONE',  ( -13.12529397354238192, 5.014845663890295846, 4.166666666666765551 ) ) ;
#14293=CARTESIAN_POINT ( 'NONE',  ( -10.47219141768317563, -23.72900456129165292, 2.724438792969417822 ) ) ;
#14295=CARTESIAN_POINT ( 'NONE',  ( 9.246558582316794173, -21.94931252712234482, 5.250000000000000888 ) ) ;
#14297=CARTESIAN_POINT ( 'NONE',  ( -12.67822638532683577, -18.31206754099172684, 6.277704579156187847 ) ) ;
#14299=CARTESIAN_POINT ( 'NONE',  ( 8.402808582316794173, -22.77556120703056308, 1.770995438708339975 ) ) ;
#14300=CARTESIAN_POINT ( 'NONE',  ( 13.12529397354238192, 5.014845663890297622, 3.999999999999981792 ) ) ;
#14311=CARTESIAN_POINT ( 'NONE',  ( -12.05905858231679595, -20.19639159124062999, 5.231925497173373074 ) ) ;
#14312=CARTESIAN_POINT ( 'NONE',  ( 12.64323021897839006, -19.32937394158751943, 5.504219675487169283 ) ) ;
#14314=CARTESIAN_POINT ( 'NONE',  ( 2.442511739767545098, -14.09457879449248807, 3.458905389639174821 ) ) ;
#14317=CARTESIAN_POINT ( 'NONE',  ( -13.38569699238614952, -18.95980188449660986, 4.749177046715717054 ) ) ;
#14319=CARTESIAN_POINT ( 'NONE',  ( 7.371558582316794173, -20.24999999999999289, 3.449312527122348371 ) ) ;
#14320=CARTESIAN_POINT ( 'NONE',  ( -12.66144083004408571, -19.15973808277258073, 6.259475412489329038 ) ) ;
#14324=CARTESIAN_POINT ( 'NONE',  ( -5.309058582316795949, -23.80360840875935935, 1.768074502826626260 ) ) ;
#14325=CARTESIAN_POINT ( 'NONE',  ( 7.184058582316794173, -20.79840458871652942, 2.226721677130544030 ) ) ;
#14326=CARTESIAN_POINT ( 'NONE',  ( 8.034691417683175629, -20.97900456129164581, 3.136473910504570917 ) ) ;
#14327=CARTESIAN_POINT ( 'NONE',  ( -11.50344141768317563, -22.05068747287765873, 5.250000000000000888 ) ) ;
#14330=CARTESIAN_POINT ( 'NONE',  ( 13.37515323800563039, -20.24226148071262799, 4.627790572011877934 ) ) ;
#14338=CARTESIAN_POINT ( 'NONE',  ( 13.37327929115833669, -20.24999999707183207, 3.449077790995325632 ) ) ;
#14341=CARTESIAN_POINT ( 'NONE',  ( -3.636036383999129207, -10.90885478516162976, 2.275977788322152584 ) ) ;
#14344=CARTESIAN_POINT ( 'NONE',  ( 2.708677329869237482, -9.785633270066144362, 1.794897081886200230 ) ) ;
#14345=CARTESIAN_POINT ( 'NONE',  ( -13.06655316810189227, 2.048434989138931961, 5.965524842914772030 ) ) ;
#14346=CARTESIAN_POINT ( 'NONE',  ( 9.809058582316794173, -23.27327832286945153, 2.298404588716537411 ) ) ;
#14348=CARTESIAN_POINT ( 'NONE',  ( 13.07148796623841847, 1.547642295024179493, 6.704787912489258872 ) ) ;
#14350=CARTESIAN_POINT ( 'NONE',  ( -2.031432063436913182, -10.08997855658269671, 1.680444048616273722 ) ) ;
#14352=CARTESIAN_POINT ( 'NONE',  ( -13.85723511636018301, 4.102873376188801657, 5.986996695041598926 ) ) ;
#14354=CARTESIAN_POINT ( 'NONE',  ( 9.159691417683175629, -22.98484643305507191, 0.9790045612916508100 ) ) ;
#14355=CARTESIAN_POINT ( 'NONE',  ( -11.30905858231679595, -22.74294823697954016, 2.828734674606448785 ) ) ;
#14358=CARTESIAN_POINT ( 'NONE',  ( 13.90439706815434739, 5.734551941788608609, 5.045486763335835789 ) ) ;
#14359=CARTESIAN_POINT ( 'NONE',  ( 12.74043380832193684, -14.42059267975384529, 5.611358176248560703 ) ) ;
#14368=CARTESIAN_POINT ( 'NONE',  ( -13.12529397354238192, 5.014845663890297622, 3.999999999999981792 ) ) ;
#14370=CARTESIAN_POINT ( 'NONE',  ( 2.327620134574780231, -13.27885108724501251, 3.249410218619480872 ) ) ;
#14376=DIRECTION ( 'NONE',  ( 0.000000000000000000, 0.000000000000000000, 1.000000000000000000 ) ) ;
#14378=CARTESIAN_POINT ( 'NONE',  ( -11.49655858231679417, -22.05068747287764452, 1.749999999999998446 ) ) ;
#14381=CARTESIAN_POINT ( 'NONE',  ( 11.96530858231679773, -20.97900456129165647, 3.863526089495444626 ) ) ;
#14382=CARTESIAN_POINT ( 'NONE',  ( -12.62746768552656285, -19.37538188090202596, 4.723115281690125400 ) ) ;
#14383=CARTESIAN_POINT ( 'NONE',  ( -6.340308582316796837, -22.36352608949544418, 4.520995438708343528 ) ) ;
#14384=CARTESIAN_POINT ( 'NONE',  ( -6.534691417683177406, -19.47900456129164581, 2.515153566944927199 ) ) ;
#14386=CARTESIAN_POINT ( 'NONE',  ( 13.08439876642066935, 3.699637704240349656, 5.251001356674258602 ) ) ;
#14391=CARTESIAN_POINT ( 'NONE',  ( 13.86616162069444691, 3.803661845068127878, 6.738770894197415373 ) ) ;
#14392=VERTEX_POINT ( 'NONE', #1055 ) ;
#14398=CARTESIAN_POINT ( 'NONE',  ( 10.37844141768317741, -23.74999999999999645, 3.449312527122335492 ) ) ;
#14400=CARTESIAN_POINT ( 'NONE',  ( -2.602174906157317835, -9.976397331638239052, 2.593889103792902606 ) ) ;
#14401=CARTESIAN_POINT ( 'NONE',  ( 2.731427961995660958, -10.89409100229510052, 2.829571171190552015 ) ) ;
#14402=CARTESIAN_POINT ( 'NONE',  ( -11.02780858231679595, -23.72900456129165292, 4.275561207030568411 ) ) ;
#14403=CARTESIAN_POINT ( 'NONE',  ( 6.815941417683177406, -20.26807450282663225, 5.303608408759377113 ) ) ;
#14405=CARTESIAN_POINT ( 'NONE',  ( -5.315941417683176518, -20.79840458871654363, 4.773278322869464851 ) ) ;
#14408=CARTESIAN_POINT ( 'NONE',  ( 7.652808582316795061, -21.22443879296942626, 5.229004561291659137 ) ) ;
#14410=CARTESIAN_POINT ( 'NONE',  ( -12.64183575740756993, -20.14979425091403087, 6.022201559249563907 ) ) ;
#14411=ORIENTED_EDGE ( 'NONE', *, *, #14801, .T. ) ;
#14412=CARTESIAN_POINT ( 'NONE',  ( 5.121558582316794173, -23.74999999999999645, 3.550687472877651629 ) ) ;
#14421=CARTESIAN_POINT ( 'NONE',  ( -12.99655858231679595, -22.05068747287764452, 0.9999999999999978906 ) ) ;
#14425=CARTESIAN_POINT ( 'NONE',  ( 2.742252025265078608, -15.06657917462210605, 2.958534504914692942 ) ) ;
#14426=CARTESIAN_POINT ( 'NONE',  ( 13.15498566372047762, 5.764276017890828108, 4.942557026581394730 ) ) ;
#14429=CARTESIAN_POINT ( 'NONE',  ( -13.84501469867711698, 4.235742283194553259, 3.666666666666500873 ) ) ;
#14430=CARTESIAN_POINT ( 'NONE',  ( 8.496558582316794173, -22.05068747287764452, 1.749999999999998446 ) ) ;
#14432=CARTESIAN_POINT ( 'NONE',  ( -12.63178515739782348, -20.65734955141111584, 5.567013446834313761 ) ) ;
#14434=CARTESIAN_POINT ( 'NONE',  ( -10.93405858231679595, -23.73192549717337130, 5.303608408759367343 ) ) ;
#14435=CARTESIAN_POINT ( 'NONE',  ( 7.559058582316794173, -20.72672167713054137, 4.701595411283463477 ) ) ;
#14437=CARTESIAN_POINT ( 'NONE',  ( 13.27780858231679417, -21.02099543870833998, 3.035098964749253003 ) ) ;
#14438=CARTESIAN_POINT ( 'NONE',  ( -5.972191417683177406, -23.72900456129164937, 2.724438792969417378 ) ) ;
#14441=CARTESIAN_POINT ( 'NONE',  ( 13.37524505148396514, -20.23762490005974968, 4.659512268729234741 ) ) ;
#14449=CARTESIAN_POINT ( 'NONE',  ( -2.171407406650392780, -8.432416083433171394, 2.389978857884845986 ) ) ;
#14454=CARTESIAN_POINT ( 'NONE',  ( -13.11740841389447709, 4.616624901677048420, 5.813473370769506765 ) ) ;
#14455=CARTESIAN_POINT ( 'NONE',  ( 12.62155858231679417, -23.74999999999999645, 3.550687472877651629 ) ) ;
#14458=CARTESIAN_POINT ( 'NONE',  ( 13.15498530132288479, 5.764257716805535559, 4.166666666666765551 ) ) ;
#14459=CARTESIAN_POINT ( 'NONE',  ( -1.709849555000590104, -9.864920124259167977, 1.622644547201689713 ) ) ;
#14461=CARTESIAN_POINT ( 'NONE',  ( -13.85223456079946303, 3.850345320370711644, 5.989742199623227847 ) ) ;
#14463=CARTESIAN_POINT ( 'NONE',  ( 9.065941417683177406, -23.73192549717336064, 1.696391591240623331 ) ) ;
#14465=CARTESIAN_POINT ( 'NONE',  ( -9.152808582316795949, -21.53509896474924901, 4.479004561291659137 ) ) ;
#14467=CARTESIAN_POINT ( 'NONE',  ( 12.62543384439201510, -20.97809085820452424, 4.782403934559678937 ) ) ;
#14468=CARTESIAN_POINT ( 'NONE',  ( 13.10252221513633941, 3.864871864382954048, 6.004587342915129966 ) ) ;
#14469=DIRECTION ( 'NONE',  ( 0.000000000000000000, 0.000000000000000000, 1.000000000000000000 ) ) ;
#14479=CARTESIAN_POINT ( 'NONE',  ( 1.665360951492234287, -9.864914341757378580, 1.622643062139706993 ) ) ;
#14486=CARTESIAN_POINT ( 'NONE',  ( -2.731427961995660958, -10.89409100229510052, 2.829571171190552015 ) ) ;
#14487=CARTESIAN_POINT ( 'NONE',  ( 8.027808582316795949, -22.97900456129165647, 3.964901035250747885 ) ) ;
#14488=CARTESIAN_POINT ( 'NONE',  ( -13.09206359972826661, 4.086711786274932479, 5.245812454509717782 ) ) ;
#14489=CARTESIAN_POINT ( 'NONE',  ( -6.621558582316796837, -22.99999999999999645, 3.550687472877652073 ) ) ;
#14490=CARTESIAN_POINT ( 'NONE',  ( -7.003441417683177406, -22.05068747287766229, 6.000000000000001776 ) ) ;
#14491=EDGE_LOOP ( 'NONE', ( #5286, #14148 ) ) ;
#14492=CARTESIAN_POINT ( 'NONE',  ( 13.84311479963346869, 4.139797381492562600, 5.195993353439945395 ) ) ;
#14494=ORIENTED_EDGE ( 'NONE', *, *, #16817, .F. ) ;
#14501=DIRECTION ( 'NONE',  ( 0.1351665943404306014, 0.9596796555888912339, -0.2464649070825229438 ) ) ;
#14503=CARTESIAN_POINT ( 'NONE',  ( -0.2815691515810352930, -9.114917468222230923, 2.372643865078523984 ) ) ;
#14504=CARTESIAN_POINT ( 'NONE',  ( 2.583953725994688533, -9.847075946378776479, 2.560676788604062004 ) ) ;
#14505=CARTESIAN_POINT ( 'NONE',  ( -13.18405858231679417, -20.79840458871652942, 2.226721677130544030 ) ) ;
#14508=CARTESIAN_POINT ( 'NONE',  ( 10.37844141768317741, -23.74999999999999645, 3.449312527122335492 ) ) ;
#14511=CARTESIAN_POINT ( 'NONE',  ( -6.440941417683176518, -20.72672167713052715, 2.298404588716546293 ) ) ;
#14513=CARTESIAN_POINT ( 'NONE',  ( 11.77780858231679595, -19.52099543870833642, 2.413778621189609286 ) ) ;
#14514=CARTESIAN_POINT ( 'NONE',  ( 12.63819864697926754, -19.58346832754827105, 5.450273968536036406 ) ) ;
#14515=CARTESIAN_POINT ( 'NONE',  ( -13.15498530131898214, 5.764257716805535559, 3.333333333333075466 ) ) ;
#14521=PRODUCT_CONTEXT ( 'NONE', #12272, 'mechanical' ) ;
#14528=CARTESIAN_POINT ( 'NONE',  ( -7.371558582316794173, -20.24999999999999289, 3.449312527122348371 ) ) ;
#14531=CARTESIAN_POINT ( 'NONE',  ( 2.627360420079438263, -14.25085146736906339, 2.749039333894452763 ) ) ;
#14532=CARTESIAN_POINT ( 'NONE',  ( 13.15498530132288479, 5.764257716805535559, 3.666666666666500873 ) ) ;
#14534=CARTESIAN_POINT ( 'NONE',  ( -13.84501469867711698, 4.235742283194553259, 4.916666666666649199 ) ) ;
#14535=CARTESIAN_POINT ( 'NONE',  ( 8.871558582316795949, -19.49999999999998934, 3.449312527122348371 ) ) ;
#14536=CARTESIAN_POINT ( 'NONE',  ( -12.62499999999998579, -20.24999999999999289, 3.666666666666653640 ) ) ;
#14539=CARTESIAN_POINT ( 'NONE',  ( 6.152808582316793284, -21.22443879296942626, 5.229004561291659137 ) ) ;
#14542=CARTESIAN_POINT ( 'NONE',  ( 5.315941417683176518, -21.32873467460645145, 4.242948236979555254 ) ) ;
#14543=CARTESIAN_POINT ( 'NONE',  ( -8.878441417683177406, -23.74999999999999645, 3.449312527122335492 ) ) ;
#14546=CARTESIAN_POINT ( 'NONE',  ( 13.37499999999998401, -20.24999999999998934, 2.439580858552613751 ) ) ;
#14552=CARTESIAN_POINT ( 'NONE',  ( -13.11740841389447709, 4.616624901677048420, 5.813473370769506765 ) ) ;
#14553=CARTESIAN_POINT ( 'NONE',  ( -2.121089610268797276, -8.411987239090384705, 1.634732322550447758 ) ) ;
#14556=CARTESIAN_POINT ( 'NONE',  ( -12.69247507894198712, -16.84250851341299082, 5.559274842915185033 ) ) ;
#14557=CARTESIAN_POINT ( 'NONE',  ( 7.090308582316795061, -21.32581373872472952, 1.729004561291657138 ) ) ;
#14559=CARTESIAN_POINT ( 'NONE',  ( 12.62499999999998224, -20.24999999999998934, 4.291666666666698937 ) ) ;
#14560=CARTESIAN_POINT ( 'NONE',  ( -1.711347482507859397, -9.865394108634699677, 1.622766275858107621 ) ) ;
#14562=CARTESIAN_POINT ( 'NONE',  ( -13.41820805991576826, -18.06799297425606454, 5.518388032956592859 ) ) ;
#14565=CARTESIAN_POINT ( 'NONE',  ( 8.878441417683177406, -24.50000000000000000, 3.449312527122335048 ) ) ;
#14566=CARTESIAN_POINT ( 'NONE',  ( -5.309058582316795949, -22.74294823697954016, 2.828734674606448785 ) ) ;
#14568=CARTESIAN_POINT ( 'NONE',  ( 13.86616162069444691, 3.803661845068127878, 6.738770894197415373 ) ) ;
#14569=CARTESIAN_POINT ( 'NONE',  ( 12.64751377014909828, -19.11305460747000495, 5.510446717915143289 ) ) ;
#14577=CARTESIAN_POINT ( 'NONE',  ( 0.5631383031621635116, -9.114917468222230923, 1.622643865078341463 ) ) ;
#14582=CARTESIAN_POINT ( 'NONE',  ( -11.68405858231679417, -20.79840458871652942, 2.226721677130544030 ) ) ;
#14583=CARTESIAN_POINT ( 'NONE',  ( -2.513306525444908512, -9.622685169956881168, 2.503048754562789746 ) ) ;
#14585=CARTESIAN_POINT ( 'NONE',  ( -12.66835678905406049, -17.31048215276408797, 4.799178440007564994 ) ) ;
#14586=CARTESIAN_POINT ( 'NONE',  ( -12.15280858231679595, -21.22443879296942626, 5.229004561291659137 ) ) ;
#14588=CARTESIAN_POINT ( 'NONE',  ( -4.378441417683176518, -23.74999999999999645, 3.449312527122335492 ) ) ;
#14590=CARTESIAN_POINT ( 'NONE',  ( 13.38269957179998038, -19.11117162410040038, 4.745921838382382241 ) ) ;
#14600=CARTESIAN_POINT ( 'NONE',  ( 11.50344141768317563, -22.05068747287765873, 5.250000000000000888 ) ) ;
#14602=CARTESIAN_POINT ( 'NONE',  ( -2.109407804498405703, -9.207748739546751438, 2.396484790045401603 ) ) ;
#14604=CARTESIAN_POINT ( 'NONE',  ( -9.434058582316794173, -23.20159541128345992, 4.773278322869455970 ) ) ;
#14606=CARTESIAN_POINT ( 'NONE',  ( 11.40969141768318096, -21.32581373872474373, 5.270995438708348857 ) ) ;
#14608=CARTESIAN_POINT ( 'NONE',  ( -3.944195004867016241, -21.61378581760806838, 5.207602947182413899 ) ) ;
#14611=CARTESIAN_POINT ( 'NONE',  ( 8.215308582316795949, -24.52099543870834708, 2.515153566944913432 ) ) ;
#14612=CARTESIAN_POINT ( 'NONE',  ( 12.64323021897839006, -19.32937394158751943, 5.504219675487169283 ) ) ;
#14613=CARTESIAN_POINT ( 'NONE',  ( -13.15316049959406364, 5.672105229501871904, 5.573635960501007958 ) ) ;
#14618=VERTEX_POINT ( 'NONE', #9412 ) ;
#14619=SHAPE_REPRESENTATION_RELATIONSHIP ( 'NONE' , 'NONE' ,  #6045, #4794 ) ;
#14624=CARTESIAN_POINT ( 'NONE',  ( -12.71530858231679417, -24.52099543870834708, 2.515153566944913432 ) ) ;
#14625=CARTESIAN_POINT ( 'NONE',  ( 13.11145189917479392, 4.315820908324673688, 5.961432613039677086 ) ) ;
#14628=CARTESIAN_POINT ( 'NONE',  ( 12.62524871736568954, -20.23743977303344010, 4.661898514667671023 ) ) ;
#14630=CARTESIAN_POINT ( 'NONE',  ( -13.84042474920106081, 4.003949834653575124, 5.242612001278796008 ) ) ;
#14631=CARTESIAN_POINT ( 'NONE',  ( 10.46530858231679595, -19.47900456129164937, 4.484846433055089676 ) ) ;
#14632=CARTESIAN_POINT ( 'NONE',  ( -13.15047398821051239, 5.536436404627260721, 5.896317606305554015 ) ) ;
#14633=CARTESIAN_POINT ( 'NONE',  ( -10.09719141768317741, -23.08622137881040359, 5.979004561291654696 ) ) ;
#14635=ADVANCED_FACE ( 'NONE', ( #6169 ), #6485, .T. ) ;
#14638=CLOSED_SHELL ( 'NONE', ( #10610, #11791, #11973, #1464, #5075, #12246, #2582, #11265, #14635, #19191, #3734, #14897, #10806, #8415, #13655, #436, #12938, #15910, #5771, #12421, #18059, #9920 ) ) ;
#14640=CARTESIAN_POINT ( 'NONE',  ( 7.277808582316795061, -21.02099543870833998, 3.035098964749253003 ) ) ;
#14641=CARTESIAN_POINT ( 'NONE',  ( -7.565941417683176518, -23.20159541128344927, 2.226721677130534705 ) ) ;
#14646=CARTESIAN_POINT ( 'NONE',  ( 13.37597619100657198, -20.20070235416671167, 4.815535977982682070 ) ) ;
#14660=CARTESIAN_POINT ( 'NONE',  ( -13.09293046926041626, 3.380488697651010011, 5.994170676248444352 ) ) ;
#14661=CARTESIAN_POINT ( 'NONE',  ( 8.215308582316792396, -23.77099543870833998, 2.825813738724734847 ) ) ;
#14664=CARTESIAN_POINT ( 'NONE',  ( 13.10012427866737639, 3.743776072700027324, 6.001983176248468332 ) ) ;
#14665=CARTESIAN_POINT ( 'NONE',  ( -2.731427961995660958, -10.89409100229510052, 2.829571171190552015 ) ) ;
#14667=CARTESIAN_POINT ( 'NONE',  ( -13.39662663169496781, -19.15785509940297615, 5.494950532956567102 ) ) ;
#14669=CARTESIAN_POINT ( 'NONE',  ( 10.65969141768318096, -22.67418626127524917, 1.729004561291651809 ) ) ;
#14670=CARTESIAN_POINT ( 'NONE',  ( -8.121558582316795949, -22.99999999999999645, 3.550687472877652073 ) ) ;
#14672=CARTESIAN_POINT ( 'NONE',  ( 13.77324158252158171, -0.8888000826463379189, 6.637859435864801760 ) ) ;
#14673=CARTESIAN_POINT ( 'NONE',  ( 13.12512971825177033, 5.006550771716304915, 5.133277049491872468 ) ) ;
#14684=CARTESIAN_POINT ( 'NONE',  ( 1.939860967060266672, -10.52577007527361808, 2.542364016426418516 ) ) ;
#14690=CARTESIAN_POINT ( 'NONE',  ( -10.46530858231679417, -20.22900456129164937, 4.174186261275266929 ) ) ;
#14691=CARTESIAN_POINT ( 'NONE',  ( -3.049989092406311109, -8.938202327316346896, 1.769874869409437279 ) ) ;
#14693=CARTESIAN_POINT ( 'NONE',  ( -13.04243487821393721, 1.580461349787872782, 5.205428440007538349 ) ) ;
#14694=CARTESIAN_POINT ( 'NONE',  ( -10.46530858231679417, -20.22900456129164937, 4.174186261275266929 ) ) ;
#14696=CARTESIAN_POINT ( 'NONE',  ( -7.565941417683176518, -23.20159541128344927, 2.226721677130534705 ) ) ;
#14698=CARTESIAN_POINT ( 'NONE',  ( 13.84501469867711698, 4.235742283194553259, 4.583333333333295734 ) ) ;
#14710=CARTESIAN_POINT ( 'NONE',  ( 4.847191417683178294, -21.22443879296941915, 1.770995438708345748 ) ) ;
#14714=CARTESIAN_POINT ( 'NONE',  ( -2.513306525444908512, -9.622685169956881168, 2.503048754562789746 ) ) ;
#14716=CARTESIAN_POINT ( 'NONE',  ( -5.590308582316794173, -21.32581373872472952, 1.729004561291657138 ) ) ;
#14718=CARTESIAN_POINT ( 'NONE',  ( 8.878441417683177406, -23.74999999999999645, 3.449312527122335492 ) ) ;
#14720=CARTESIAN_POINT ( 'NONE',  ( -6.534691417683176518, -20.22900456129164581, 2.825813738724747726 ) ) ;
#14722=CARTESIAN_POINT ( 'NONE',  ( 12.99655858231679595, -22.05068747287764452, 0.9999999999999978906 ) ) ;
#14723=CARTESIAN_POINT ( 'NONE',  ( 12.64691428603184242, -19.14332855539073464, 5.509795676248469221 ) ) ;
#14724=CARTESIAN_POINT ( 'NONE',  ( -13.15498530132288479, 5.764257716805535559, 4.583333333333295734 ) ) ;
#14738=CARTESIAN_POINT ( 'NONE',  ( 12.66849571425264287, -18.05346643024382303, 5.533233176248494978 ) ) ;
#14742=CARTESIAN_POINT ( 'NONE',  ( 12.62515553039088090, -20.24214571525854467, 4.629702272822510345 ) ) ;
#14744=CARTESIAN_POINT ( 'NONE',  ( -13.37499999999998224, -20.24999999999991829, 4.333333333333343695 ) ) ;
#14745=CARTESIAN_POINT ( 'NONE',  ( 11.02780858231679595, -24.47900456129166358, 4.586221378810390270 ) ) ;
#14746=CARTESIAN_POINT ( 'NONE',  ( -13.15384296923648400, 5.706569946443514674, 5.461568745250741763 ) ) ;
#14747=CARTESIAN_POINT ( 'NONE',  ( -4.934058582316795061, -23.73192549717337130, 5.303608408759367343 ) ) ;
#14750=CARTESIAN_POINT ( 'NONE',  ( 11.30905858231679595, -22.74294823697954016, 2.828734674606448785 ) ) ;
#14751=CARTESIAN_POINT ( 'NONE',  ( -9.909691417683179182, -21.32581373872474373, 5.270995438708348857 ) ) ;
#14754=CARTESIAN_POINT ( 'NONE',  ( 13.83770801678722329, 3.866754847752558621, 5.240062463382368030 ) ) ;
#14761=CARTESIAN_POINT ( 'NONE',  ( 13.37883250981221472, -20.05645825448334563, 5.102688967256983510 ) ) ;
#14765=CARTESIAN_POINT ( 'NONE',  ( 3.996922828336520794, -14.62728872172488437, 3.980945906412841850 ) ) ;
#14766=CARTESIAN_POINT ( 'NONE',  ( 1.948765222931501784, -9.143197003266354983, 1.629906614618163552 ) ) ;
#14767=CARTESIAN_POINT ( 'NONE',  ( -12.62499994688180749, -19.50000268246798640, 4.473800639250938183 ) ) ;
#14768=CARTESIAN_POINT ( 'NONE',  ( 9.152808582316794173, -21.22443879296942626, 5.229004561291660025 ) ) ;
#14770=CARTESIAN_POINT ( 'NONE',  ( 12.62503117662529739, -20.24842558042254836, 4.565011198945062354 ) ) ;
#14772=CARTESIAN_POINT ( 'NONE',  ( -0.9854920305337622199, -9.864917468222230923, 2.372643865078341019 ) ) ;
#14775=CARTESIAN_POINT ( 'NONE',  ( 6.159691417683176518, -22.67418626127524917, 1.729004561291651809 ) ) ;
#14776=CARTESIAN_POINT ( 'NONE',  ( -7.465308582316796837, -20.97900456129165647, 3.863526089495444626 ) ) ;
#14778=CARTESIAN_POINT ( 'NONE',  ( 13.86676110481170632, 3.833935792988865110, 6.739421935864088553 ) ) ;
#14779=CARTESIAN_POINT ( 'NONE',  ( 12.65650603190776025, -18.65894538865861563, 5.520212342915047365 ) ) ;
#14790=CARTESIAN_POINT ( 'NONE',  ( 2.067263844777544435, -10.27417889452513933, 1.727750375171331676 ) ) ;
#14793=CARTESIAN_POINT ( 'NONE',  ( 12.70105350217228413, -20.47677344150786283, 3.540713189489502977 ) ) ;
#14795=CARTESIAN_POINT ( 'NONE',  ( -10.65280858231679240, -21.22443879296942626, 5.229004561291659137 ) ) ;
#14796=CARTESIAN_POINT ( 'NONE',  ( -0.2815691515810352374, -8.364917468222230923, 2.372643865078523540 ) ) ;
#14798=CARTESIAN_POINT ( 'NONE',  ( -12.65396917024039958, -18.03705690286155772, 4.783553440007634272 ) ) ;
#14799=CARTESIAN_POINT ( 'NONE',  ( -8.121558582316792396, -23.74999999999999645, 3.550687472877651629 ) ) ;
#14801=EDGE_CURVE ( 'NONE', #15169, #17122, #11599, .T. ) ;
#14802=CARTESIAN_POINT ( 'NONE',  ( -6.065941417683177406, -23.20159541128344927, 2.226721677130534705 ) ) ;
#14804=CARTESIAN_POINT ( 'NONE',  ( 13.83890698502169059, 3.927302743594121903, 5.241364546715693074 ) ) ;
#14813=CARTESIAN_POINT ( 'NONE',  ( 7.472191417683176518, -23.72900456129164937, 2.724438792969417378 ) ) ;
#14819=CARTESIAN_POINT ( 'NONE',  ( 7.659691417683177406, -22.67418626127524917, 1.729004561291651809 ) ) ;
#14821=CARTESIAN_POINT ( 'NONE',  ( -11.31594141768317741, -21.32873467460645145, 4.242948236979555254 ) ) ;
#14822=CARTESIAN_POINT ( 'NONE',  ( -9.902808582316795949, -23.08622137881038938, 1.020995438708339309 ) ) ;
#14824=CARTESIAN_POINT ( 'NONE',  ( 12.63465172146706728, -19.76258806590802664, 5.372658420469845986 ) ) ;
#14826=CARTESIAN_POINT ( 'NONE',  ( -13.10026320386584153, 3.000791795219782454, 6.736037912489353019 ) ) ;
#14831=( BOUNDED_SURFACE ( )  B_SPLINE_SURFACE ( 3, 2, ( 
 ( #1932, #4658, #11050, #1524, #4764, #4864, #15846, #7904, #11149, #16170, #3293, #17518, #17738, #11244, #8006, #14268, #3403, #3199, #14582, #1625, #14378, #16063, #6448, #8118, #163, #9783, #1833, #257, #3712, #14795, #4018, #14690, #6950, #7061, #11650, #5484, #5381, #11553, #7165, #16774, #8623, #18249, #5274, #9981, #569, #3813, #371, #19521, #474, #5173, #17933, #18148, #19831, #10403, #13425, #13124, #3602, #2140, #16561, #16364, #10092, #2443, #11857, #10191, #6755, #2040, #18041, #8428, #10292, #14993, #674, #6848, #2236, #13217, #19616, #18353, #3912, #16662, #16467, #8522, #19930, #13528, #13320, #14891, #19721, #15102, #2340, #5587, #11757, #8734, #779, #11958, #2651, #18872, #10711 ),
 ( #1293, #10918, #2763, #12376, #20138, #4122, #17185, #879, #4533, #9141, #9238, #7474, #16975, #5798, #8835, #7672, #7263, #1094, #9039, #18660, #15610, #6109, #14042, #10503, #20452, #4221, #4436, #18459, #17280, #18770, #13624, #4328, #13934, #2863, #15302, #12479, #15203, #12069, #5896, #7572, #20032, #16873, #2543, #5694, #15411, #10601, #13833, #8931, #12169, #981, #7370, #20238, #13734, #18557, #12266, #17085, #15511, #1193, #20337, #6001, #10820, #8267, #14844, #3554, #7879, #5331, #6803, #8374, #6204, #8477, #5224, #11022, #11507, #15717, #19080, #11705, #16314, #13073, #2965, #12573, #6305, #18974, #19571, #17887, #9935, #9341, #6702, #15820, #17391, #6900, #14747, #1987, #4628, #3074, #519 ),
 ( #5022, #3657, #424, #13268, #1401, #9449, #13171, #11402, #17787, #19667, #5127, #14146, #12677, #1498, #11602, #3455, #17987, #9833, #10040, #7783, #16417, #20553, #14239, #2093, #16218, #20646, #1887, #14633, #318, #19473, #18298, #7008, #4073, #7215, #18201, #3766, #10146, #10459, #13577, #830, #16925, #18409, #5853, #8788, #12013, #11908, #3961, #8573, #5752, #20086, #19779, #15048, #10241, #14943, #3864, #621, #18101, #2397, #10556, #10349, #2287, #7317, #19979, #8885, #16607, #15254, #13479, #5640, #12122, #20193, #18514, #8678, #15360, #4175, #16828, #931, #7426, #13678, #733, #2599, #13377, #5437, #13788, #7116, #16517, #19882, #8987, #2189, #16722, #2492, #11810, #5538, #15156, #1041, #2711 ),
 ( #4583, #10659, #9093, #20398, #14098, #15463, #7926, #6061, #20291, #1248, #4487, #4686, #7622, #12321, #1548, #12223, #10872, #10971, #9190, #3024, #2916, #1148, #11077, #14293, #6160, #15772, #2816, #7525, #20601, #4273, #20704, #12528, #12627, #17237, #12430, #15565, #18612, #17448, #17033, #9293, #18825, #1352, #19031, #9500, #3126, #13889, #15872, #13990, #7832, #5948, #18719, #1453, #4386, #7733, #17341, #6253, #10769, #17137, #15668, #20507, #18925, #9400, #14194, #15973, #9595, #14720, #14511, #8147, #188, #6367, #9705, #19140, #12736, #17763, #2069, #6476, #8039, #4791, #14405, #8243, #11483, #17863, #11374, #3432, #17960, #6677, #11269, #8454, #9909, #3533, #1655, #11580, #8344, #90, #14608 ),
 ( #11173, #12836, #17547, #3224, #9809, #16290, #16391, #19446, #19239, #4889, #6570, #286, #17650, #1761, #14821, #5104, #16196, #3323, #16091, #12935, #19340, #1961, #13046, #397, #4995, #1861, #6780, #13150, #10012, #19547, #5202, #3631, #597, #5729, #13654, #18176, #13352, #18073, #6983, #3739, #496, #5512, #20065, #7090, #5410, #10434, #16695, #11990, #19752, #18388, #16586, #2373, #2472, #2574, #8863, #11784, #18490, #15232, #3938, #4051, #10534, #16804, #3838, #906, #10121, #16493, #16903, #10218, #19643, #2263, #7291, #6876, #13455, #10326, #13245, #5302, #8652, #11676, #2165, #8762, #5614, #8959, #13555, #8549, #14919, #15024, #15134, #705, #19859, #11884, #19956, #808, #18276, #7192, #12100 ),
 ( #4152, #15334, #18802, #7506, #9072, #19007, #6139, #14075, #17009, #15444, #20581, #7812, #13968, #4663, #10745, #15749, #1331, #6234, #1014, #2686, #2894, #17115, #9171, #11054, #17216, #5830, #18695, #4252, #20483, #15546, #12508, #4361, #3000, #17427, #18906, #7405, #3103, #9375, #7602, #13766, #2797, #20170, #12199, #12604, #1226, #10632, #7707, #4468, #1128, #18589, #13869, #4563, #10853, #9270, #14174, #15643, #20269, #6036, #10948, #20373, #12408, #5927, #1431, #17314, #12298, #11153, #6452, #1630, #6342, #15948, #12713, #9480, #14489, #1936, #16067, #14383, #19425, #4972, #261, #8010, #6652, #4869, #11351, #11458, #11557, #17842, #66, #6759, #3507, #12913, #13022, #19525, #5082, #12816, #9888 ),
 ( #19215, #7908, #11248, #16268, #15850, #1740, #19316, #1529, #14272, #17627, #20679, #19116, #17742, #14586, #5178, #1838, #4768, #17523, #3299, #3406, #3204, #9681, #17938, #8223, #9788, #9575, #8122, #166, #6549, #8320, #16174, #14694, #376, #13128, #16471, #18046, #7268, #15107, #2344, #5278, #3718, #8839, #16779, #2240, #13628, #19725, #4022, #10296, #15207, #9987, #11654, #11861, #5386, #18152, #20037, #5488, #14799, #6954, #13223, #8738, #3817, #783, #13326, #11962, #5699, #7169, #16368, #12073, #18359, #16565, #2047, #11761, #8432, #3606, #883, #10195, #19620, #16668, #13430, #10096, #478, #6852, #13532, #19835, #7066, #2447, #3916, #2144, #14998, #18254, #8628, #679, #8526, #10407, #5591 ) ),
 .UNSPECIFIED., .T., .F., .F. ) 
 B_SPLINE_SURFACE_WITH_KNOTS ( ( 4, 3, 4 ),
 ( 3, 2, 2, 2, 2, 2, 2, 2, 2, 2, 2, 2, 2, 2, 2, 2, 2, 2, 2, 2, 2, 2, 2, 2, 2, 2, 2, 2, 2, 2, 2, 2, 2, 2, 2, 2, 2, 2, 2, 2, 2, 2, 2, 2, 2, 2, 2, 3 ),
 ( 0.000000000000000000, 0.5000000000000000000, 1.000000000000000000 ),
 ( 0.000000000000000000, 0.02083333333333333218, 0.04166666666666666435, 0.06250000000000000000, 0.08333333333333332871, 0.1041666666666666713, 0.1250000000000000000, 0.1458333333333333426, 0.1666666666666666574, 0.1875000000000000000, 0.2083333333333333426, 0.2291666666666666574, 0.2500000000000000000, 0.2708333333333333148, 0.2916666666666666852, 0.3125000000000000000, 0.3333333333333333148, 0.3541666666666666852, 0.3750000000000000000, 0.3958333333333333148, 0.4166666666666666852, 0.4375000000000000000, 0.4583333333333333148, 0.4791666666666666852, 0.5000000000000000000, 0.5208333333333333703, 0.5416666666666666297, 0.5625000000000000000, 0.5833333333333333703, 0.6041666666666666297, 0.6250000000000000000, 0.6458333333333333703, 0.6666666666666666297, 0.6875000000000000000, 0.7083333333333333703, 0.7291666666666666297, 0.7500000000000000000, 0.7708333333333333703, 0.7916666666666666297, 0.8125000000000000000, 0.8333333333333333703, 0.8541666666666666297, 0.8750000000000000000, 0.8958333333333333703, 0.9166666666666666297, 0.9375000000000000000, 0.9583333333333333703, 0.9650437087885355147 ),
 .UNSPECIFIED. ) 
 GEOMETRIC_REPRESENTATION_ITEM ( )  RATIONAL_B_SPLINE_SURFACE ( (
 ( 1.000000000000000000, 0.9238795325112867385, 1.000000000000000000, 0.9238795325112867385, 1.000000000000000000, 0.9238795325112867385, 1.000000000000000000, 0.9238795325112867385, 1.000000000000000000, 0.9238795325112867385, 1.000000000000000000, 0.9238795325112867385, 1.000000000000000000, 0.9238795325112867385, 1.000000000000000000, 0.9238795325112867385, 1.000000000000000000, 0.9238795325112867385, 1.000000000000000000, 0.9238795325112867385, 1.000000000000000000, 0.9238795325112867385, 1.000000000000000000, 0.9238795325112867385, 1.000000000000000000, 0.9238795325112867385, 1.000000000000000000, 0.9238795325112867385, 1.000000000000000000, 0.9238795325112867385, 1.000000000000000000, 0.9238795325112867385, 1.000000000000000000, 0.9238795325112867385, 1.000000000000000000, 0.9238795325112867385, 1.000000000000000000, 0.9238795325112867385, 1.000000000000000000, 0.9238795325112867385, 1.000000000000000000, 0.9238795325112867385, 1.000000000000000000, 0.9238795325112867385, 1.000000000000000000, 0.9238795325112867385, 1.000000000000000000, 0.9238795325112867385, 1.000000000000000000, 0.9238795325112867385, 1.000000000000000000, 0.9238795325112867385, 1.000000000000000000, 0.9238795325112867385, 1.000000000000000000, 0.9238795325112867385, 1.000000000000000000, 0.9238795325112867385, 1.000000000000000000, 0.9238795325112867385, 1.000000000000000000, 0.9238795325112867385, 1.000000000000000000, 0.9238795325112867385, 1.000000000000000000, 0.9238795325112867385, 1.000000000000000000, 0.9238795325112867385, 1.000000000000000000, 0.9238795325112867385, 1.000000000000000000, 0.9238795325112867385, 1.000000000000000000, 0.9238795325112867385, 1.000000000000000000, 0.9238795325112867385, 1.000000000000000000, 0.9238795325112867385, 1.000000000000000000, 0.9238795325112867385, 1.000000000000000000, 0.9238795325112867385, 1.000000000000000000, 0.9238795325112867385, 1.000000000000000000, 0.9238795325112867385, 1.000000000000000000, 0.9238795325112867385, 1.000000000000000000, 0.9238795325112867385, 1.000000000000000000, 0.9238795325112867385, 1.000000000000000000, 0.9754817479996107377, 0.9667580569362973497),
 ( 0.3333333333333333703, 0.3079598441704289313, 0.3333333333333333703, 0.3079598441704289313, 0.3333333333333333703, 0.3079598441704289313, 0.3333333333333333703, 0.3079598441704289313, 0.3333333333333333703, 0.3079598441704289313, 0.3333333333333333703, 0.3079598441704289313, 0.3333333333333333703, 0.3079598441704289313, 0.3333333333333333703, 0.3079598441704289313, 0.3333333333333333703, 0.3079598441704289313, 0.3333333333333333703, 0.3079598441704289313, 0.3333333333333333703, 0.3079598441704289313, 0.3333333333333333703, 0.3079598441704289313, 0.3333333333333333703, 0.3079598441704289313, 0.3333333333333333703, 0.3079598441704289313, 0.3333333333333333703, 0.3079598441704289313, 0.3333333333333333703, 0.3079598441704289313, 0.3333333333333333703, 0.3079598441704289313, 0.3333333333333333703, 0.3079598441704289313, 0.3333333333333333703, 0.3079598441704289313, 0.3333333333333333703, 0.3079598441704289313, 0.3333333333333333703, 0.3079598441704289313, 0.3333333333333333703, 0.3079598441704289313, 0.3333333333333333703, 0.3079598441704289313, 0.3333333333333333703, 0.3079598441704289313, 0.3333333333333333703, 0.3079598441704289313, 0.3333333333333333703, 0.3079598441704289313, 0.3333333333333333703, 0.3079598441704289313, 0.3333333333333333703, 0.3079598441704289313, 0.3333333333333333703, 0.3079598441704289313, 0.3333333333333333703, 0.3079598441704289313, 0.3333333333333333703, 0.3079598441704289313, 0.3333333333333333703, 0.3079598441704289313, 0.3333333333333333703, 0.3079598441704289313, 0.3333333333333333703, 0.3079598441704289313, 0.3333333333333333703, 0.3079598441704289313, 0.3333333333333333703, 0.3079598441704289313, 0.3333333333333333703, 0.3079598441704289313, 0.3333333333333333703, 0.3079598441704289313, 0.3333333333333333703, 0.3079598441704289313, 0.3333333333333333703, 0.3079598441704289313, 0.3333333333333333703, 0.3079598441704289313, 0.3333333333333333703, 0.3079598441704289313, 0.3333333333333333703, 0.3079598441704289313, 0.3333333333333333703, 0.3079598441704289313, 0.3333333333333333703, 0.3079598441704289313, 0.3333333333333333703, 0.3079598441704289313, 0.3333333333333333703, 0.3251605826665369681, 0.3222526856454325239),
 ( 0.3333333333333333703, 0.3079598441704289313, 0.3333333333333333703, 0.3079598441704289313, 0.3333333333333333703, 0.3079598441704289313, 0.3333333333333333703, 0.3079598441704289313, 0.3333333333333333703, 0.3079598441704289313, 0.3333333333333333703, 0.3079598441704289313, 0.3333333333333333703, 0.3079598441704289313, 0.3333333333333333703, 0.3079598441704289313, 0.3333333333333333703, 0.3079598441704289313, 0.3333333333333333703, 0.3079598441704289313, 0.3333333333333333703, 0.3079598441704289313, 0.3333333333333333703, 0.3079598441704289313, 0.3333333333333333703, 0.3079598441704289313, 0.3333333333333333703, 0.3079598441704289313, 0.3333333333333333703, 0.3079598441704289313, 0.3333333333333333703, 0.3079598441704289313, 0.3333333333333333703, 0.3079598441704289313, 0.3333333333333333703, 0.3079598441704289313, 0.3333333333333333703, 0.3079598441704289313, 0.3333333333333333703, 0.3079598441704289313, 0.3333333333333333703, 0.3079598441704289313, 0.3333333333333333703, 0.3079598441704289313, 0.3333333333333333703, 0.3079598441704289313, 0.3333333333333333703, 0.3079598441704289313, 0.3333333333333333703, 0.3079598441704289313, 0.3333333333333333703, 0.3079598441704289313, 0.3333333333333333703, 0.3079598441704289313, 0.3333333333333333703, 0.3079598441704289313, 0.3333333333333333703, 0.3079598441704289313, 0.3333333333333333703, 0.3079598441704289313, 0.3333333333333333703, 0.3079598441704289313, 0.3333333333333333703, 0.3079598441704289313, 0.3333333333333333703, 0.3079598441704289313, 0.3333333333333333703, 0.3079598441704289313, 0.3333333333333333703, 0.3079598441704289313, 0.3333333333333333703, 0.3079598441704289313, 0.3333333333333333703, 0.3079598441704289313, 0.3333333333333333703, 0.3079598441704289313, 0.3333333333333333703, 0.3079598441704289313, 0.3333333333333333703, 0.3079598441704289313, 0.3333333333333333703, 0.3079598441704289313, 0.3333333333333333703, 0.3079598441704289313, 0.3333333333333333703, 0.3079598441704289313, 0.3333333333333333703, 0.3079598441704289313, 0.3333333333333333703, 0.3079598441704289313, 0.3333333333333333703, 0.3079598441704289313, 0.3333333333333333703, 0.3251605826665369681, 0.3222526856454325239),
 ( 1.000000000000000000, 0.9238795325112867385, 1.000000000000000000, 0.9238795325112867385, 1.000000000000000000, 0.9238795325112867385, 1.000000000000000000, 0.9238795325112867385, 1.000000000000000000, 0.9238795325112867385, 1.000000000000000000, 0.9238795325112867385, 1.000000000000000000, 0.9238795325112867385, 1.000000000000000000, 0.9238795325112867385, 1.000000000000000000, 0.9238795325112867385, 1.000000000000000000, 0.9238795325112867385, 1.000000000000000000, 0.9238795325112867385, 1.000000000000000000, 0.9238795325112867385, 1.000000000000000000, 0.9238795325112867385, 1.000000000000000000, 0.9238795325112867385, 1.000000000000000000, 0.9238795325112867385, 1.000000000000000000, 0.9238795325112867385, 1.000000000000000000, 0.9238795325112867385, 1.000000000000000000, 0.9238795325112867385, 1.000000000000000000, 0.9238795325112867385, 1.000000000000000000, 0.9238795325112867385, 1.000000000000000000, 0.9238795325112867385, 1.000000000000000000, 0.9238795325112867385, 1.000000000000000000, 0.9238795325112867385, 1.000000000000000000, 0.9238795325112867385, 1.000000000000000000, 0.9238795325112867385, 1.000000000000000000, 0.9238795325112867385, 1.000000000000000000, 0.9238795325112867385, 1.000000000000000000, 0.9238795325112867385, 1.000000000000000000, 0.9238795325112867385, 1.000000000000000000, 0.9238795325112867385, 1.000000000000000000, 0.9238795325112867385, 1.000000000000000000, 0.9238795325112867385, 1.000000000000000000, 0.9238795325112867385, 1.000000000000000000, 0.9238795325112867385, 1.000000000000000000, 0.9238795325112867385, 1.000000000000000000, 0.9238795325112867385, 1.000000000000000000, 0.9238795325112867385, 1.000000000000000000, 0.9238795325112867385, 1.000000000000000000, 0.9238795325112867385, 1.000000000000000000, 0.9238795325112867385, 1.000000000000000000, 0.9238795325112867385, 1.000000000000000000, 0.9238795325112867385, 1.000000000000000000, 0.9238795325112867385, 1.000000000000000000, 0.9238795325112867385, 1.000000000000000000, 0.9238795325112867385, 1.000000000000000000, 0.9238795325112867385, 1.000000000000000000, 0.9754817479996107377, 0.9667580569362973497),
 ( 0.3333333333333333703, 0.3079598441704289313, 0.3333333333333333703, 0.3079598441704289313, 0.3333333333333333703, 0.3079598441704289313, 0.3333333333333333703, 0.3079598441704289313, 0.3333333333333333703, 0.3079598441704289313, 0.3333333333333333703, 0.3079598441704289313, 0.3333333333333333703, 0.3079598441704289313, 0.3333333333333333703, 0.3079598441704289313, 0.3333333333333333703, 0.3079598441704289313, 0.3333333333333333703, 0.3079598441704289313, 0.3333333333333333703, 0.3079598441704289313, 0.3333333333333333703, 0.3079598441704289313, 0.3333333333333333703, 0.3079598441704289313, 0.3333333333333333703, 0.3079598441704289313, 0.3333333333333333703, 0.3079598441704289313, 0.3333333333333333703, 0.3079598441704289313, 0.3333333333333333703, 0.3079598441704289313, 0.3333333333333333703, 0.3079598441704289313, 0.3333333333333333703, 0.3079598441704289313, 0.3333333333333333703, 0.3079598441704289313, 0.3333333333333333703, 0.3079598441704289313, 0.3333333333333333703, 0.3079598441704289313, 0.3333333333333333703, 0.3079598441704289313, 0.3333333333333333703, 0.3079598441704289313, 0.3333333333333333703, 0.3079598441704289313, 0.3333333333333333703, 0.3079598441704289313, 0.3333333333333333703, 0.3079598441704289313, 0.3333333333333333703, 0.3079598441704289313, 0.3333333333333333703, 0.3079598441704289313, 0.3333333333333333703, 0.3079598441704289313, 0.3333333333333333703, 0.3079598441704289313, 0.3333333333333333703, 0.3079598441704289313, 0.3333333333333333703, 0.3079598441704289313, 0.3333333333333333703, 0.3079598441704289313, 0.3333333333333333703, 0.3079598441704289313, 0.3333333333333333703, 0.3079598441704289313, 0.3333333333333333703, 0.3079598441704289313, 0.3333333333333333703, 0.3079598441704289313, 0.3333333333333333703, 0.3079598441704289313, 0.3333333333333333703, 0.3079598441704289313, 0.3333333333333333703, 0.3079598441704289313, 0.3333333333333333703, 0.3079598441704289313, 0.3333333333333333703, 0.3079598441704289313, 0.3333333333333333703, 0.3079598441704289313, 0.3333333333333333703, 0.3079598441704289313, 0.3333333333333333703, 0.3079598441704289313, 0.3333333333333333703, 0.3251605826665369681, 0.3222526856454325239),
 ( 0.3333333333333333703, 0.3079598441704289313, 0.3333333333333333703, 0.3079598441704289313, 0.3333333333333333703, 0.3079598441704289313, 0.3333333333333333703, 0.3079598441704289313, 0.3333333333333333703, 0.3079598441704289313, 0.3333333333333333703, 0.3079598441704289313, 0.3333333333333333703, 0.3079598441704289313, 0.3333333333333333703, 0.3079598441704289313, 0.3333333333333333703, 0.3079598441704289313, 0.3333333333333333703, 0.3079598441704289313, 0.3333333333333333703, 0.3079598441704289313, 0.3333333333333333703, 0.3079598441704289313, 0.3333333333333333703, 0.3079598441704289313, 0.3333333333333333703, 0.3079598441704289313, 0.3333333333333333703, 0.3079598441704289313, 0.3333333333333333703, 0.3079598441704289313, 0.3333333333333333703, 0.3079598441704289313, 0.3333333333333333703, 0.3079598441704289313, 0.3333333333333333703, 0.3079598441704289313, 0.3333333333333333703, 0.3079598441704289313, 0.3333333333333333703, 0.3079598441704289313, 0.3333333333333333703, 0.3079598441704289313, 0.3333333333333333703, 0.3079598441704289313, 0.3333333333333333703, 0.3079598441704289313, 0.3333333333333333703, 0.3079598441704289313, 0.3333333333333333703, 0.3079598441704289313, 0.3333333333333333703, 0.3079598441704289313, 0.3333333333333333703, 0.3079598441704289313, 0.3333333333333333703, 0.3079598441704289313, 0.3333333333333333703, 0.3079598441704289313, 0.3333333333333333703, 0.3079598441704289313, 0.3333333333333333703, 0.3079598441704289313, 0.3333333333333333703, 0.3079598441704289313, 0.3333333333333333703, 0.3079598441704289313, 0.3333333333333333703, 0.3079598441704289313, 0.3333333333333333703, 0.3079598441704289313, 0.3333333333333333703, 0.3079598441704289313, 0.3333333333333333703, 0.3079598441704289313, 0.3333333333333333703, 0.3079598441704289313, 0.3333333333333333703, 0.3079598441704289313, 0.3333333333333333703, 0.3079598441704289313, 0.3333333333333333703, 0.3079598441704289313, 0.3333333333333333703, 0.3079598441704289313, 0.3333333333333333703, 0.3079598441704289313, 0.3333333333333333703, 0.3079598441704289313, 0.3333333333333333703, 0.3079598441704289313, 0.3333333333333333703, 0.3251605826665369681, 0.3222526856454325239),
 ( 1.000000000000000000, 0.9238795325112867385, 1.000000000000000000, 0.9238795325112867385, 1.000000000000000000, 0.9238795325112867385, 1.000000000000000000, 0.9238795325112867385, 1.000000000000000000, 0.9238795325112867385, 1.000000000000000000, 0.9238795325112867385, 1.000000000000000000, 0.9238795325112867385, 1.000000000000000000, 0.9238795325112867385, 1.000000000000000000, 0.9238795325112867385, 1.000000000000000000, 0.9238795325112867385, 1.000000000000000000, 0.9238795325112867385, 1.000000000000000000, 0.9238795325112867385, 1.000000000000000000, 0.9238795325112867385, 1.000000000000000000, 0.9238795325112867385, 1.000000000000000000, 0.9238795325112867385, 1.000000000000000000, 0.9238795325112867385, 1.000000000000000000, 0.9238795325112867385, 1.000000000000000000, 0.9238795325112867385, 1.000000000000000000, 0.9238795325112867385, 1.000000000000000000, 0.9238795325112867385, 1.000000000000000000, 0.9238795325112867385, 1.000000000000000000, 0.9238795325112867385, 1.000000000000000000, 0.9238795325112867385, 1.000000000000000000, 0.9238795325112867385, 1.000000000000000000, 0.9238795325112867385, 1.000000000000000000, 0.9238795325112867385, 1.000000000000000000, 0.9238795325112867385, 1.000000000000000000, 0.9238795325112867385, 1.000000000000000000, 0.9238795325112867385, 1.000000000000000000, 0.9238795325112867385, 1.000000000000000000, 0.9238795325112867385, 1.000000000000000000, 0.9238795325112867385, 1.000000000000000000, 0.9238795325112867385, 1.000000000000000000, 0.9238795325112867385, 1.000000000000000000, 0.9238795325112867385, 1.000000000000000000, 0.9238795325112867385, 1.000000000000000000, 0.9238795325112867385, 1.000000000000000000, 0.9238795325112867385, 1.000000000000000000, 0.9238795325112867385, 1.000000000000000000, 0.9238795325112867385, 1.000000000000000000, 0.9238795325112867385, 1.000000000000000000, 0.9238795325112867385, 1.000000000000000000, 0.9238795325112867385, 1.000000000000000000, 0.9238795325112867385, 1.000000000000000000, 0.9238795325112867385, 1.000000000000000000, 0.9238795325112867385, 1.000000000000000000, 0.9754817479996107377, 0.9667580569362973497) ) ) 
 REPRESENTATION_ITEM ( '' )  SURFACE ( )  );
#14835=CARTESIAN_POINT ( 'NONE',  ( 2.596731678114175157, -9.937710376390764822, 2.583953520835782225 ) ) ;
#14838=CARTESIAN_POINT ( 'NONE',  ( 13.10624331898488037, 4.052787608736739600, 6.006964772046813117 ) ) ;
#14840=CARTESIAN_POINT ( 'NONE',  ( 12.62500016093973620, -20.24999187254239175, 4.532396751752561848 ) ) ;
#14842=CARTESIAN_POINT ( 'NONE',  ( 7.840308582316795949, -22.98484643305508612, 6.020995438708344416 ) ) ;
#14843=CARTESIAN_POINT ( 'NONE',  ( -12.85087781109329974, -9.593170539812428288, 6.465204579154565145 ) ) ;
#14844=CARTESIAN_POINT ( 'NONE',  ( -7.559058582316795949, -20.19639159124062999, 5.231925497173373074 ) ) ;
#14848=CARTESIAN_POINT ( 'NONE',  ( 11.21530858231679595, -23.02099543870833998, 3.136473910504556262 ) ) ;
#14850=CARTESIAN_POINT ( 'NONE',  ( -8.597191417683177406, -22.77556120703057729, 5.229004561291656472 ) ) ;
#14853=CARTESIAN_POINT ( 'NONE',  ( 13.87367531042247748, 4.933103176334663331, 5.324010972534209074 ) ) ;
#14860=CARTESIAN_POINT ( 'NONE',  ( 13.84667963294518778, 4.277765388965502957, 4.000000000000000888 ) ) ;
#14861=CARTESIAN_POINT ( 'NONE',  ( 13.75871503850933841, -0.8723905552644914962, 5.888179699623941943 ) ) ;
#14863=CARTESIAN_POINT ( 'NONE',  ( 1.787053415088318609, -8.367039355952382351, 2.373188808236395886 ) ) ;
#14866=CARTESIAN_POINT ( 'NONE',  ( -12.62966097655984754, -19.26462068372267566, 4.756751955311774083 ) ) ;
#14867=CARTESIAN_POINT ( 'NONE',  ( 8.590308582316794173, -21.32581373872472952, 1.729004561291657138 ) ) ;
#14869=CARTESIAN_POINT ( 'NONE',  ( 13.10821839766814279, 4.152529082241303904, 5.997503362667785609 ) ) ;
#14870=CARTESIAN_POINT ( 'NONE',  ( -2.659620708751979645, -10.38426118526329489, 2.698636689302993830 ) ) ;
#14871=CARTESIAN_POINT ( 'NONE',  ( 6.996558582316795949, -22.05068747287764452, 2.499999999999999112 ) ) ;
#14873=CARTESIAN_POINT ( 'NONE',  ( 11.50344141768317563, -22.05068747287765873, 5.250000000000000888 ) ) ;
#14874=CARTESIAN_POINT ( 'NONE',  ( -5.215308582316795949, -23.02099543870833998, 3.136473910504556262 ) ) ;
#14876=CARTESIAN_POINT ( 'NONE',  ( 13.11824772738305356, 3.909010232842670796, 6.755569162489314827 ) ) ;
#14877=CARTESIAN_POINT ( 'NONE',  ( 12.66835678905406049, -17.31048215276408797, 4.799178440007564994 ) ) ;
#14878=CARTESIAN_POINT ( 'NONE',  ( -12.62499999999990230, -20.15044198641778195, 3.551156945994470071 ) ) ;
#14885=DIRECTION ( 'NONE',  ( -0.1351665943404306014, -0.9596796555888911229, 0.2464649070825229160 ) ) ;
#14886=CARTESIAN_POINT ( 'NONE',  ( 1.337453470010121714, -9.864917468222230923, 2.372643865078341019 ) ) ;
#14889=CARTESIAN_POINT ( 'NONE',  ( 12.62499999999998224, -20.29300445137376485, 3.551156945995087799 ) ) ;
#14891=CARTESIAN_POINT ( 'NONE',  ( -5.590308582316794173, -21.32581373872472597, 1.729004561291657582 ) ) ;
#14892=CARTESIAN_POINT ( 'NONE',  ( -0.2815691515810352930, -9.114917468222230923, 2.372643865078523984 ) ) ;
#14895=CARTESIAN_POINT ( 'NONE',  ( -13.09560264576187905, 4.265433610975056133, 4.166666666666765551 ) ) ;
#14897=ADVANCED_FACE ( 'NONE', ( #2276 ), #19769, .T. ) ;
#14898=CARTESIAN_POINT ( 'NONE',  ( -7.378441417683176518, -23.74999999999999645, 3.449312527122335492 ) ) ;
#14901=CARTESIAN_POINT ( 'NONE',  ( 13.37818000216760694, -19.33940989053615311, 4.728953261990445966 ) ) ;
#14906=ORIENTED_EDGE ( 'NONE', *, *, #12473, .F. ) ;
#14907=CARTESIAN_POINT ( 'NONE',  ( -13.37503071710846925, -20.24844878602346299, 4.564052989354591361 ) ) ;
#14913=CARTESIAN_POINT ( 'NONE',  ( 3.211992482548209349, -9.366834950279640637, 2.629956289783360823 ) ) ;
#14915=CARTESIAN_POINT ( 'NONE',  ( 12.65986935584910000, -19.23909752961862907, 6.257782094979345899 ) ) ;
#14917=CARTESIAN_POINT ( 'NONE',  ( 9.159691417683179182, -22.67418626127524917, 1.729004561291651809 ) ) ;
#14919=CARTESIAN_POINT ( 'NONE',  ( -4.753441417683176518, -21.94931252712233061, 2.499999999999999112 ) ) ;
#14920=CARTESIAN_POINT ( 'NONE',  ( -6.715308582316796837, -24.52099543870834708, 2.515153566944913432 ) ) ;
#14922=CARTESIAN_POINT ( 'NONE',  ( 12.64931222250080545, -19.02223276370786209, 5.512399842915133519 ) ) ;
#14923=CARTESIAN_POINT ( 'NONE',  ( -13.15498530132288479, 5.764257716805535559, 4.916666666666649199 ) ) ;
#14929=CARTESIAN_POINT ( 'NONE',  ( 13.28039013372821131, -20.00084031961838704, 3.461764366045932295 ) ) ;
#14934=CARTESIAN_POINT ( 'NONE',  ( -1.720709671993384093, -9.114925383610804843, 1.622645897908254753 ) ) ;
#14941=CARTESIAN_POINT ( 'NONE',  ( 8.965308582316795949, -19.47900456129164937, 4.484846433055089676 ) ) ;
#14942=CARTESIAN_POINT ( 'NONE',  ( -12.70700162295422864, -16.85891804079483691, 6.308954579156044851 ) ) ;
#14943=CARTESIAN_POINT ( 'NONE',  ( -7.659691417683177406, -22.98484643305507191, 0.9790045612916508100 ) ) ;
#14946=CARTESIAN_POINT ( 'NONE',  ( 12.15280858231679950, -21.53509896474924901, 4.479004561291659137 ) ) ;
#14947=CARTESIAN_POINT ( 'NONE',  ( -3.974842109207561425, -21.82955800590261930, 5.256404853634145447 ) ) ;
#14950=CARTESIAN_POINT ( 'NONE',  ( 13.87470602645761986, 4.985154336109792972, 4.916666666666650087 ) ) ;
#14958=CARTESIAN_POINT ( 'NONE',  ( 13.85980676119184629, 4.232741440188380722, 5.965367510457697975 ) ) ;
#14960=CARTESIAN_POINT ( 'NONE',  ( 3.270401025279431995, -9.547343748290430199, 2.676314555138040063 ) ) ;
#14963=CARTESIAN_POINT ( 'NONE',  ( -12.62499999999998401, -19.49999999999998934, 2.439580858552613751 ) ) ;
#14964=CARTESIAN_POINT ( 'NONE',  ( 5.590308582316794173, -21.32581373872472952, 1.729004561291657138 ) ) ;
#14966=CARTESIAN_POINT ( 'NONE',  ( 12.66369984131459070, -18.29565801360988075, 5.528024842915327142 ) ) ;
#14968=CARTESIAN_POINT ( 'NONE',  ( 0.000000000000000000, -9.864917468222230923, 2.372643865078341019 ) ) ;
#14970=CARTESIAN_POINT ( 'NONE',  ( 11.49655858231679595, -22.05068747287764452, 2.499999999999999112 ) ) ;
#14972=CARTESIAN_POINT ( 'NONE',  ( 11.69094141768317563, -23.27327832286946219, 4.701595411283453707 ) ) ;
#14973=CARTESIAN_POINT ( 'NONE',  ( -8.027808582316792396, -23.72900456129165647, 4.275561207030568411 ) ) ;
#14975=CARTESIAN_POINT ( 'NONE',  ( 12.75496035233418013, -14.43700220713569138, 6.361037912489419632 ) ) ;
#14977=CARTESIAN_POINT ( 'NONE',  ( 13.09300823383486900, 4.134415808666423331, 5.226944302881396887 ) ) ;
#14988=CARTESIAN_POINT ( 'NONE',  ( 0.9854920305337621089, -9.114917468222230923, 2.372643865078341019 ) ) ;
#14991=CARTESIAN_POINT ( 'NONE',  ( 12.71341536712609965, -20.49194379261451715, 3.539064175304416082 ) ) ;
#14993=CARTESIAN_POINT ( 'NONE',  ( -6.902808582316793284, -22.77556120703056308, 1.770995438708339975 ) ) ;
#14994=CARTESIAN_POINT ( 'NONE',  ( -3.521144778809589315, -10.09312707791070096, 2.066482617302010105 ) ) ;
#14997=CARTESIAN_POINT ( 'NONE',  ( -13.37732542738919328, -19.38256591684242025, 4.710253041318374301 ) ) ;
#14998=CARTESIAN_POINT ( 'NONE',  ( -5.121558582316794173, -23.74999999999999645, 3.550687472877651629 ) ) ;
#14999=CARTESIAN_POINT ( 'NONE',  ( -11.50344141768317741, -22.05068747287766229, 4.499999999999999112 ) ) ;
#15002=CARTESIAN_POINT ( 'NONE',  ( 13.39359219590679295, -19.31109410670777038, 5.491647114909025795 ) ) ;
#15009=CARTESIAN_POINT ( 'NONE',  ( -13.37597619100657198, -20.20070235416671167, 4.815535977982682070 ) ) ;
#15016=CARTESIAN_POINT ( 'NONE',  ( -13.87500000000000000, 5.000000000000049738, 4.000000000000000888 ) ) ;
#15017=CARTESIAN_POINT ( 'NONE',  ( 3.594802210173583035, -11.77224174634763898, 3.247712807842289884 ) ) ;
#15018=CARTESIAN_POINT ( 'NONE',  ( -7.277808582316795061, -20.27099543870833642, 2.724438792969431589 ) ) ;
#15020=CARTESIAN_POINT ( 'NONE',  ( 13.90439735423465351, 5.734566389025032684, 3.333333333332063386 ) ) ;
#15021=PLANE ( 'NONE',  #16636 ) ;
#15022=CARTESIAN_POINT ( 'NONE',  ( 10.65969141768317741, -22.36352608949543352, 2.479004561291652031 ) ) ;
#15023=CARTESIAN_POINT ( 'NONE',  ( -12.62888984277510218, -20.05356293986039873, 5.111704976569332537 ) ) ;
#15024=CARTESIAN_POINT ( 'NONE',  ( -4.659691417683177406, -22.36352608949543352, 2.479004561291652031 ) ) ;
#15025=CARTESIAN_POINT ( 'NONE',  ( -8.496558582316795949, -22.05068747287764452, 0.9999999999999978906 ) ) ;
#15027=CARTESIAN_POINT ( 'NONE',  ( 13.12529397354238192, 5.014845663890295846, 4.791666666666685614 ) ) ;
#15028=CARTESIAN_POINT ( 'NONE',  ( -12.69247507894198712, -16.84250851341299082, 5.559274842915185033 ) ) ;
#15037=ORIENTED_EDGE ( 'NONE', *, *, #2402, .T. ) ;
#15039=CARTESIAN_POINT ( 'NONE',  ( 13.10372118337080849, 3.925419760224517329, 6.005889426248455010 ) ) ;
#15040=CARTESIAN_POINT ( 'NONE',  ( -1.754777266914451461, -9.116337928146160507, 1.623008667563337726 ) ) ;
#15043=CARTESIAN_POINT ( 'NONE',  ( 13.12463908936614132, 4.981774012991869505, 5.264611377988129171 ) ) ;
#15045=CARTESIAN_POINT ( 'NONE',  ( 6.902808582316795949, -23.08622137881038938, 1.020995438708339309 ) ) ;
#15046=CARTESIAN_POINT ( 'NONE',  ( -13.12529397354238192, 5.014845663890295846, 4.666666666666619889 ) ) ;
#15048=CARTESIAN_POINT ( 'NONE',  ( -7.847191417683175629, -20.91377862118959285, 1.020995438708345082 ) ) ;
#15054=CARTESIAN_POINT ( 'NONE',  ( -13.40621837757088564, -18.67347193267085714, 5.505367199623145247 ) ) ;
#15056=CARTESIAN_POINT ( 'NONE',  ( 9.340308582316795949, -22.36352608949544418, 4.520995438708343528 ) ) ;
#15060=CARTESIAN_POINT ( 'NONE',  ( 13.85528666703740619, 4.004476685417483139, 5.993048563355776182 ) ) ;
#15067=CARTESIAN_POINT ( 'NONE',  ( 13.39296152110871851, -19.34294318400601753, 5.489418334493660012 ) ) ;
#15070=CARTESIAN_POINT ( 'NONE',  ( 3.451187703687236041, -10.75258211228477734, 2.985843844067104680 ) ) ;
#15072=CARTESIAN_POINT ( 'NONE',  ( -12.63036675113625407, -19.22897906761645004, 4.757923088130392664 ) ) ;
#15074=CARTESIAN_POINT ( 'NONE',  ( 12.99655858231679417, -22.05068747287764452, 1.749999999999998446 ) ) ;
#15075=CARTESIAN_POINT ( 'NONE',  ( 13.11017182064853159, 4.251176942750957366, 5.979809059808775196 ) ) ;
#15076=CARTESIAN_POINT ( 'NONE',  ( -1.513434189748285696, -9.114917468222230923, 2.372643865078341019 ) ) ;
#15077=CARTESIAN_POINT ( 'NONE',  ( 8.871558582316795949, -20.99999999999999645, 3.449312527122348371 ) ) ;
#15079=CARTESIAN_POINT ( 'NONE',  ( 6.628441417683176518, -20.24999999999999289, 3.550687472877664952 ) ) ;
#15080=CARTESIAN_POINT ( 'NONE',  ( -11.68405858231679417, -20.79840458871652942, 2.226721677130544030 ) ) ;
#15082=CARTESIAN_POINT ( 'NONE',  ( 12.65679946139692902, -19.39412719945235253, 6.251687395662565372 ) ) ;
#15083=CARTESIAN_POINT ( 'NONE',  ( 12.62525331949183105, -19.48720736566255951, 4.581880915780448760 ) ) ;
#15096=CARTESIAN_POINT ( 'NONE',  ( 1.742625132518061504, -9.872369070458363538, 2.374557585393312298 ) ) ;
#15098=CARTESIAN_POINT ( 'NONE',  ( -13.87500000000000178, 5.000000000000047962, 2.000000000000000000 ) ) ;
#15100=CARTESIAN_POINT ( 'NONE',  ( 13.33061827858665893, -20.43393009137478344, 3.455122606006641561 ) ) ;
#15102=CARTESIAN_POINT ( 'NONE',  ( -5.402808582316794173, -22.77556120703056308, 1.770995438708339975 ) ) ;
#15103=CARTESIAN_POINT ( 'NONE',  ( -1.126276606324276619, -8.364917468222230923, 2.372643865078341019 ) ) ;
#15105=CARTESIAN_POINT ( 'NONE',  ( -13.09560264576187905, 4.265433610975056133, 4.916666666666649199 ) ) ;
#15107=CARTESIAN_POINT ( 'NONE',  ( -9.902808582316794173, -22.77556120703056308, 1.770995438708339975 ) ) ;
#15108=CARTESIAN_POINT ( 'NONE',  ( 7.652808582316796837, -20.91377862118960351, 5.979004561291660913 ) ) ;
#15109=CARTESIAN_POINT ( 'NONE',  ( -7.190941417683177406, -22.74294823697955081, 4.171265325393542334 ) ) ;
#15110=ORIENTED_EDGE ( 'NONE', *, *, #15196, .T. ) ;
#15111=CARTESIAN_POINT ( 'NONE',  ( 13.37741471237955260, -20.12805702483293757, 4.993653275319895890 ) ) ;
#15112=CARTESIAN_POINT ( 'NONE',  ( -2.693754455098655409, -10.14181605509423711, 1.874202551270839123 ) ) ;
#15119=CARTESIAN_POINT ( 'NONE',  ( -13.37499999999998579, -20.24999999999999289, 3.482947684955674639 ) ) ;
#15126=CARTESIAN_POINT ( 'NONE',  ( 1.787053415088318609, -8.367039355952382351, 2.373188808236395886 ) ) ;
#15127=CARTESIAN_POINT ( 'NONE',  ( -8.121558582316792396, -23.74999999999999645, 3.550687472877651629 ) ) ;
#15130=CARTESIAN_POINT ( 'NONE',  ( 13.90326467458556969, 5.677366066573198644, 5.457668599364335904 ) ) ;
#15132=CARTESIAN_POINT ( 'NONE',  ( 5.034691417683178294, -20.22900456129164581, 2.825813738724747726 ) ) ;
#15134=CARTESIAN_POINT ( 'NONE',  ( -4.565941417683176518, -22.67126532539353789, 2.757051763020445634 ) ) ;
#15135=CARTESIAN_POINT ( 'NONE',  ( -5.027808582316795949, -24.47900456129166358, 4.586221378810390270 ) ) ;
#15137=CARTESIAN_POINT ( 'NONE',  ( 12.64197948789552051, -18.64253586127677309, 4.770532606674187548 ) ) ;
#15138=CARTESIAN_POINT ( 'NONE',  ( -13.12529397354238192, 5.014845663890295846, 4.583333333333296622 ) ) ;
#15149=CARTESIAN_POINT ( 'NONE',  ( -2.722060606927515725, -8.660968749821154944, 1.698675748411476283 ) ) ;
#15154=CARTESIAN_POINT ( 'NONE',  ( 10.47219141768317741, -24.47900456129165292, 2.413778621189595963 ) ) ;
#15155=CARTESIAN_POINT ( 'NONE',  ( -13.12424783836753228, 4.962015837561366993, 5.328858059679200565 ) ) ;
#15156=CARTESIAN_POINT ( 'NONE',  ( -4.003441417683175629, -22.05068747287766229, 6.000000000000001776 ) ) ;
#15158=CARTESIAN_POINT ( 'NONE',  ( 12.90280858231679773, -22.77556120703056308, 1.770995438708339975 ) ) ;
#15160=CARTESIAN_POINT ( 'NONE',  ( -13.86436316834274329, 3.712840001305938831, 6.736817769197426031 ) ) ;
#15161=CARTESIAN_POINT ( 'NONE',  ( 13.27780858231679595, -20.27099543870833642, 2.724438792969431589 ) ) ;
#15166=CARTESIAN_POINT ( 'NONE',  ( 13.87470602645761986, 4.985154336109792972, 4.333333333333382775 ) ) ;
#15169=VERTEX_POINT ( 'NONE', #19130 ) ;
#15173=CARTESIAN_POINT ( 'NONE',  ( 13.87470602645761986, 4.985154336109792972, 4.833333333333344584 ) ) ;
#15175=CARTESIAN_POINT ( 'NONE',  ( 1.655860418491166941, -9.114909740826840689, 2.372641880528837621 ) ) ;
#15176=EDGE_CURVE ( 'NONE', #2288, #9910, #19015, .T. ) ;
#15178=CARTESIAN_POINT ( 'NONE',  ( -12.64197948789552051, -18.64253586127677309, 4.770532606674187548 ) ) ;
#15181=CARTESIAN_POINT ( 'NONE',  ( -13.87470602645761986, 4.985154336109792972, 4.166666666666765551 ) ) ;
#15183=CARTESIAN_POINT ( 'NONE',  ( 11.30905858231679417, -23.27327832286945153, 2.298404588716537411 ) ) ;
#15184=CARTESIAN_POINT ( 'NONE',  ( 9.534691417683177406, -20.97900456129164581, 3.136473910504570917 ) ) ;
#15185=CARTESIAN_POINT ( 'NONE',  ( -9.715308582316794173, -23.77099543870833998, 2.825813738724734847 ) ) ;
#15186=ORIENTED_EDGE ( 'NONE', *, *, #6414, .T. ) ;
#15187=CARTESIAN_POINT ( 'NONE',  ( 12.66863463945108137, -18.79645070772368953, 6.267287912489321045 ) ) ;
#15188=CARTESIAN_POINT ( 'NONE',  ( 12.62562661273123332, -19.46835605706984040, 4.628101975944573176 ) ) ;
#15196=EDGE_CURVE ( 'NONE', #13563, #18369, #19127, .T. ) ;
#15198=CARTESIAN_POINT ( 'NONE',  ( 1.513434189748285696, -9.114917468222230923, 2.372643865078341019 ) ) ;
#15203=CARTESIAN_POINT ( 'NONE',  ( -9.996558582316795949, -22.05068747287764452, 0.9999999999999978906 ) ) ;
#15204=CARTESIAN_POINT ( 'NONE',  ( -1.619022621591187150, -9.114917468222230923, 1.622643865078341463 ) ) ;
#15206=CARTESIAN_POINT ( 'NONE',  ( -13.09559422631463654, 4.265008428887424152, 5.017082219073495608 ) ) ;
#15207=CARTESIAN_POINT ( 'NONE',  ( -8.871558582316794173, -20.24999999999999289, 3.449312527122348371 ) ) ;
#15208=CARTESIAN_POINT ( 'NONE',  ( 7.559058582316795949, -20.19639159124062999, 5.231925497173373074 ) ) ;
#15209=CARTESIAN_POINT ( 'NONE',  ( -9.722191417683177406, -21.02099543870834353, 3.964901035250761208 ) ) ;
#15211=CARTESIAN_POINT ( 'NONE',  ( 13.39662663169496781, -19.15785509940297615, 5.494950532956567102 ) ) ;
#15218=CARTESIAN_POINT ( 'NONE',  ( -13.38921792038197900, -19.53199502070850357, 5.456033026503027017 ) ) ;
#15219=ORIENTED_EDGE ( 'NONE', *, *, #19539, .T. ) ;
#15223=CARTESIAN_POINT ( 'NONE',  ( 3.537356407578672535, -11.36437789272258669, 3.142965222332344766 ) ) ;
#15227=CARTESIAN_POINT ( 'NONE',  ( 13.90439735423812273, 5.734566389025032684, 2.999999999999999556 ) ) ;
#15230=CARTESIAN_POINT ( 'NONE',  ( 12.62844141768317741, -20.99999999999999645, 3.550687472877664952 ) ) ;
#15231=CARTESIAN_POINT ( 'NONE',  ( -12.62499999999998224, -20.24999999999991829, 4.333333333333343695 ) ) ;
#15232=CARTESIAN_POINT ( 'NONE',  ( -7.284691417683176518, -23.02099543870834353, 3.863526089495429972 ) ) ;
#15233=CARTESIAN_POINT ( 'NONE',  ( -7.940941417683175629, -20.19639159124061933, 1.768074502826635586 ) ) ;
#15236=CARTESIAN_POINT ( 'NONE',  ( 12.70672377255832686, -15.37294948583620346, 4.840845106674187548 ) ) ;
#15237=LINE ( 'NONE', #910, #3201 ) ;
#15247=CARTESIAN_POINT ( 'NONE',  ( -2.589709240944451096, -9.559844081062008669, 1.736909907557668165 ) ) ;
#15252=CARTESIAN_POINT ( 'NONE',  ( 5.121558582316795061, -24.50000000000000000, 3.550687472877651629 ) ) ;
#15253=CARTESIAN_POINT ( 'NONE',  ( -13.11145189917479392, 4.315820908324673688, 5.961432613039677086 ) ) ;
#15254=CARTESIAN_POINT ( 'NONE',  ( -6.534691417683177406, -19.47900456129164581, 2.515153566944927199 ) ) ;
#15256=CARTESIAN_POINT ( 'NONE',  ( 11.30905858231679417, -23.27327832286945153, 2.298404588716537411 ) ) ;
#15258=CARTESIAN_POINT ( 'NONE',  ( -13.89992416064626646, 5.508670112635706495, 5.888743936161951353 ) ) ;
#15259=CARTESIAN_POINT ( 'NONE',  ( 11.21530858231679417, -23.77099543870833998, 2.825813738724734847 ) ) ;
#15263=CARTESIAN_POINT ( 'NONE',  ( 13.58606361274418184, -9.591287556442823714, 5.700679699621803209 ) ) ;
#15271=CARTESIAN_POINT ( 'NONE',  ( 3.385922596301560894, -9.481287983549590237, 1.909350115156127403 ) ) ;
#15276=CARTESIAN_POINT ( 'NONE',  ( -13.09300823383486900, 4.134415808666423331, 5.226944302881396887 ) ) ;
#15277=CARTESIAN_POINT ( 'NONE',  ( 10.65280858231679240, -21.22443879296942626, 5.229004561291659137 ) ) ;
#15278=CARTESIAN_POINT ( 'NONE',  ( -13.86796007304617717, 3.894483688830428836, 6.740724019197413597 ) ) ;
#15281=CARTESIAN_POINT ( 'NONE',  ( 10.55905858231679595, -20.72672167713054137, 4.701595411283463477 ) ) ;
#15282=CARTESIAN_POINT ( 'NONE',  ( 12.25344141768317741, -21.94931252712233061, 2.499999999999999112 ) ) ;
#15283=CARTESIAN_POINT ( 'NONE',  ( -9.246558582316794173, -21.94931252712234482, 5.250000000000000888 ) ) ;
#15285=CARTESIAN_POINT ( 'NONE',  ( 12.62691554569741648, -19.40326494227377907, 4.703927990036796736 ) ) ;
#15292=CARTESIAN_POINT ( 'NONE',  ( -12.91308523408712183, -5.701695678577235249, 5.798858176249892082 ) ) ;
#15293=CARTESIAN_POINT ( 'NONE',  ( -3.047379876266447685, -13.13734219723468755, 3.405682891496055742 ) ) ;
#15294=CARTESIAN_POINT ( 'NONE',  ( -13.84983662433050178, 3.729249528687784920, 5.987138032956566214 ) ) ;
#15297=CARTESIAN_POINT ( 'NONE',  ( 1.407845757905374695, -9.114917468222230923, 2.372643865078341019 ) ) ;
#15302=CARTESIAN_POINT ( 'NONE',  ( -10.18405858231679595, -20.26807450282662160, 1.696391591240633101 ) ) ;
#15303=CARTESIAN_POINT ( 'NONE',  ( -3.462011766956747394, -14.92507028461178287, 3.114807177791267812 ) ) ;
#15305=CARTESIAN_POINT ( 'NONE',  ( -13.37500751150753864, -19.49962066887028556, 4.515663405036051792 ) ) ;
#15307=CARTESIAN_POINT ( 'NONE',  ( 11.87844141768317741, -24.50000000000000000, 3.449312527122335048 ) ) ;
#15308=CARTESIAN_POINT ( 'NONE',  ( -8.222191417683175629, -21.02099543870834353, 3.964901035250761208 ) ) ;
#15310=CARTESIAN_POINT ( 'NONE',  ( 13.44218742460511073, -16.85703505742523234, 5.544429699623282914 ) ) ;
#15318=CARTESIAN_POINT ( 'NONE',  ( -13.87367531042247748, 4.933103176334663331, 5.324010972534209074 ) ) ;
#15325=CARTESIAN_POINT ( 'NONE',  ( 3.034277558025862298, -9.029550313327863620, 2.543334857076493094 ) ) ;
#15327=CARTESIAN_POINT ( 'NONE',  ( 12.65017171054692113, -19.72882861737994631, 6.192581331858542981 ) ) ;
#15331=CARTESIAN_POINT ( 'NONE',  ( 13.12529397354238192, 5.014845663890295846, 4.916666666666650087 ) ) ;
#15332=CARTESIAN_POINT ( 'NONE',  ( 5.503441417683176518, -22.05068747287765873, 5.250000000000000888 ) ) ;
#15334=CARTESIAN_POINT ( 'NONE',  ( -13.27780858231679417, -21.02099543870833998, 3.035098964749253003 ) ) ;
#15335=CARTESIAN_POINT ( 'NONE',  ( -9.440941417683177406, -20.19639159124061933, 1.768074502826635586 ) ) ;
#15337=CARTESIAN_POINT ( 'NONE',  ( 12.62500000000002132, -19.50000000000273559, 4.083333333315724012 ) ) ;
#15338=CARTESIAN_POINT ( 'NONE',  ( -13.12119116326504908, 4.807653744879115010, 5.626470997801169105 ) ) ;
#15343=CARTESIAN_POINT ( 'NONE',  ( 1.903957340438703572, -10.27085516675799148, 2.476896775482616331 ) ) ;
#15352=CARTESIAN_POINT ( 'NONE',  ( -1.897597015127918230, -9.924601616748528699, 1.637971946730535588 ) ) ;
#15356=CARTESIAN_POINT ( 'NONE',  ( -13.50000000000000178, 5.000000000000047962, 4.000000000000000000 ) ) ;
#15358=CARTESIAN_POINT ( 'NONE',  ( 11.78469141768317741, -24.52099543870834708, 4.484846433055073689 ) ) ;
#15359=CARTESIAN_POINT ( 'NONE',  ( -13.12270769621861355, 4.884238659038159902, 5.513847264053151065 ) ) ;
#15360=CARTESIAN_POINT ( 'NONE',  ( -5.878441417683177406, -24.50000000000000000, 3.449312527122335048 ) ) ;
#15362=CARTESIAN_POINT ( 'NONE',  ( 11.12155858231679417, -23.74999999999999645, 3.550687472877651629 ) ) ;
#15364=CARTESIAN_POINT ( 'NONE',  ( -13.88045627189955233, 4.525541730927888473, 6.662882075361062029 ) ) ;
#15365=AXIS2_PLACEMENT_3D ( 'NONE', #1522, #19208, #14266 ) ;
#15366=CARTESIAN_POINT ( 'NONE',  ( 5.402808582316795949, -22.46490103525074034, 2.520995438708341307 ) ) ;
#15370=CARTESIAN_POINT ( 'NONE',  ( 13.42793873098995938, -18.32659408500397191, 6.262859435864284841 ) ) ;
#15374=DIRECTION ( 'NONE',  ( -0.1351665943404259662, -0.9596796555888893465, 0.2464649070825324084 ) ) ;
#15378=CARTESIAN_POINT ( 'NONE',  ( -12.15280858231679595, -21.22443879296942626, 5.229004561291659137 ) ) ;
#15379=CARTESIAN_POINT ( 'NONE',  ( 13.87066368810231154, 4.781016249162736820, 5.617237349937618696 ) ) ;
#15381=CARTESIAN_POINT ( 'NONE',  ( 3.451003380014874722, -9.682417022083358304, 1.961004070207825523 ) ) ;
#15385=CARTESIAN_POINT ( 'NONE',  ( -13.08739618700683849, 3.851007443844064237, 5.254256565007597857 ) ) ;
#15386=CARTESIAN_POINT ( 'NONE',  ( 10.55905858231679595, -20.72672167713054137, 4.701595411283463477 ) ) ;
#15387=CARTESIAN_POINT ( 'NONE',  ( -13.39782821820594627, -19.84717498059871943, 6.143582220458365661 ) ) ;
#15388=DIRECTION ( 'NONE',  ( 1.000000000000000000, 0.000000000000000000, 0.000000000000000000 ) ) ;
#15389=CARTESIAN_POINT ( 'NONE',  ( 12.90280858231679773, -22.77556120703056308, 1.770995438708339975 ) ) ;
#15390=CARTESIAN_POINT ( 'NONE',  ( 5.128441417683177406, -20.24999999999999289, 3.550687472877664952 ) ) ;
#15391=CARTESIAN_POINT ( 'NONE',  ( -8.590308582316794173, -21.32581373872472597, 1.729004561291657582 ) ) ;
#15393=CARTESIAN_POINT ( 'NONE',  ( 13.38210008768272630, -19.14144557202113006, 4.745270796715706396 ) ) ;
#15401=CARTESIAN_POINT ( 'NONE',  ( -12.66369984131459070, -18.29565801360988075, 5.528024842915327142 ) ) ;
#15402=CARTESIAN_POINT ( 'NONE',  ( -2.602174906157317835, -9.976397331638239052, 2.593889103792902606 ) ) ;
#15403=CARTESIAN_POINT ( 'NONE',  ( -13.47096266223369376, -15.40388555723029462, 5.575679699623145247 ) ) ;
#15410=CARTESIAN_POINT ( 'NONE',  ( 4.509702210102195075, -21.45583770899529696, 5.512481659358018149 ) ) ;
#15411=CARTESIAN_POINT ( 'NONE',  ( -9.246558582316795949, -21.94931252712234127, 6.000000000000001776 ) ) ;
#15412=CARTESIAN_POINT ( 'NONE',  ( -1.407845757905374695, -8.364917468222230923, 1.622643865078341907 ) ) ;
#15414=CARTESIAN_POINT ( 'NONE',  ( -13.37524505148396514, -20.23762490005974968, 4.659512268729234741 ) ) ;
#15416=CARTESIAN_POINT ( 'NONE',  ( 5.684058582316795949, -20.26807450282662160, 1.696391591240633101 ) ) ;
#15417=CARTESIAN_POINT ( 'NONE',  ( -7.753441417683177406, -21.94931252712233061, 2.499999999999999112 ) ) ;
#15419=CARTESIAN_POINT ( 'NONE',  ( 13.43259567872942917, -17.34141822415733714, 5.534013032956523581 ) ) ;
#15427=CARTESIAN_POINT ( 'NONE',  ( -13.87470602645761986, 4.985154336109792972, 4.666666666666619889 ) ) ;
#15435=CARTESIAN_POINT ( 'NONE',  ( 2.121089610268797276, -8.411987239090384705, 1.634732322550447758 ) ) ;
#15437=CARTESIAN_POINT ( 'NONE',  ( 13.10431844137356627, 3.955581289335645234, 6.006545679920360925 ) ) ;
#15441=CARTESIAN_POINT ( 'NONE',  ( 13.12529397353891270, 5.014845663890295846, 3.333333333333220239 ) ) ;
#15442=CARTESIAN_POINT ( 'NONE',  ( 8.409691417683177406, -21.63647391050456648, 4.520995438708348857 ) ) ;
#15444=CARTESIAN_POINT ( 'NONE',  ( -12.52780858231679773, -22.97900456129165647, 3.964901035250747885 ) ) ;
#15445=CARTESIAN_POINT ( 'NONE',  ( -7.847191417683175629, -20.91377862118959285, 1.020995438708345082 ) ) ;
#15447=CARTESIAN_POINT ( 'NONE',  ( 12.62499999999998224, -19.49999999999991473, 4.333333333333343695 ) ) ;
#15448=CARTESIAN_POINT ( 'NONE',  ( -12.64931222250080545, -19.02223276370786209, 5.512399842915133519 ) ) ;
#15452=CARTESIAN_POINT ( 'NONE',  ( 1.824488249492779879, -9.124319963227819130, 2.375058613629473570 ) ) ;
#15457=CARTESIAN_POINT ( 'NONE',  ( -1.126276606324276619, -9.114917468222230923, 1.622643865078341463 ) ) ;
#15461=CARTESIAN_POINT ( 'NONE',  ( 12.25344141768317741, -21.94931252712233061, 0.9999999999999978906 ) ) ;
#15462=CARTESIAN_POINT ( 'NONE',  ( -13.10624331898488037, 4.052787608736739600, 6.006964772046813117 ) ) ;
#15463=CARTESIAN_POINT ( 'NONE',  ( -12.15969141768317741, -22.67418626127524917, 1.729004561291651809 ) ) ;
#15469=CARTESIAN_POINT ( 'NONE',  ( -13.84997554952896515, 2.986265251207539606, 6.721192769197450012 ) ) ;
#15471=CARTESIAN_POINT ( 'NONE',  ( 4.687312169500634340, -21.70215802671379990, 4.455959925339818106 ) ) ;
#15475=CARTESIAN_POINT ( 'NONE',  ( 13.39995901559228031, -19.73956971259024229, 6.178279423016713956 ) ) ;
#15483=CARTESIAN_POINT ( 'NONE',  ( 3.549867680106858714, -10.29705900472337632, 2.118856410057032402 ) ) ;
#15485=CARTESIAN_POINT ( 'NONE',  ( -13.37499999999998401, -19.49999999999998934, 3.666666666666654084 ) ) ;
#15486=CARTESIAN_POINT ( 'NONE',  ( 13.27780858231679595, -20.27099543870833642, 2.724438792969431589 ) ) ;
#15487=CARTESIAN_POINT ( 'NONE',  ( -13.42793873098995938, -18.32659408500397191, 6.262859435864284841 ) ) ;
#15490=CARTESIAN_POINT ( 'NONE',  ( 12.15280858231679595, -21.22443879296942626, 5.229004561291659137 ) ) ;
#15491=CARTESIAN_POINT ( 'NONE',  ( 12.15969141768317918, -22.36352608949543352, 2.479004561291652031 ) ) ;
#15492=CARTESIAN_POINT ( 'NONE',  ( -7.465308582316795061, -20.22900456129164937, 4.174186261275266929 ) ) ;
#15495=CARTESIAN_POINT ( 'NONE',  ( 13.37499999999998401, -19.49999999999998934, 3.666666666666654084 ) ) ;
#15502=CARTESIAN_POINT ( 'NONE',  ( -13.10431844137356627, 3.955581289335645234, 6.006545679920360925 ) ) ;
#15504=CARTESIAN_POINT ( 'NONE',  ( -13.39722611581222189, -19.12758115148224647, 5.495601574623241170 ) ) ;
#15511=CARTESIAN_POINT ( 'NONE',  ( -8.121558582316795949, -24.50000000000000000, 3.550687472877651629 ) ) ;
#15512=CARTESIAN_POINT ( 'NONE',  ( -1.906542528716098417, -8.376716462152538512, 1.625674082428238298 ) ) ;
#15514=CARTESIAN_POINT ( 'NONE',  ( -13.84167967300649238, 4.067323486828401613, 5.231641758301140754 ) ) ;
#15516=CARTESIAN_POINT ( 'NONE',  ( 4.840308582316795061, -22.98484643305508612, 6.020995438708344416 ) ) ;
#15517=CARTESIAN_POINT ( 'NONE',  ( -4.753441417683176518, -21.94931252712233061, 2.499999999999999112 ) ) ;
#15519=CARTESIAN_POINT ( 'NONE',  ( 13.87470602645761986, 4.985154336109792972, 4.833333333333344584 ) ) ;
#15520=CARTESIAN_POINT ( 'NONE',  ( 12.63249216759192350, -19.87164553660301536, 5.297612231341934041 ) ) ;
#15525=CARTESIAN_POINT ( 'NONE',  ( -13.40022353639839103, -18.97621141187856608, 5.498856782956575984 ) ) ;
#15534=CARTESIAN_POINT ( 'NONE',  ( 3.528325504133930313, -10.14411005961392398, 2.079576065490765124 ) ) ;
#15543=CIRCLE ( 'NONE', #15882, 0.3750000000000003331 ) ;
#15544=CARTESIAN_POINT ( 'NONE',  ( 7.847191417683175629, -21.53509896474923835, 2.520995438708346192 ) ) ;
#15545=CARTESIAN_POINT ( 'NONE',  ( -13.11740841389447709, 4.616624901677048420, 5.813473370769506765 ) ) ;
#15546=CARTESIAN_POINT ( 'NONE',  ( -10.65280858231679595, -21.53509896474924901, 4.479004561291659137 ) ) ;
#15547=CARTESIAN_POINT ( 'NONE',  ( -11.03469141768317741, -19.47900456129164581, 2.515153566944927199 ) ) ;
#15549=CARTESIAN_POINT ( 'NONE',  ( 13.09560264576187905, 4.265433610975056133, 4.583333333333295734 ) ) ;
#15554=CARTESIAN_POINT ( 'NONE',  ( 1.407845757905374695, -9.864917468222230923, 2.372643865078341019 ) ) ;
#15559=CARTESIAN_POINT ( 'NONE',  ( -2.512468814886674284, -13.43512376012158782, 2.539544162874482591 ) ) ;
#15563=CARTESIAN_POINT ( 'NONE',  ( 5.784691417683178294, -24.52099543870834708, 4.484846433055073689 ) ) ;
#15565=CARTESIAN_POINT ( 'NONE',  ( -9.347191417683177406, -21.22443879296941915, 1.770995438708345748 ) ) ;
#15567=CARTESIAN_POINT ( 'NONE',  ( 8.402808582316794173, -22.77556120703056308, 1.770995438708339975 ) ) ;
#15569=CARTESIAN_POINT ( 'NONE',  ( -13.37671366598624800, -20.91345986769124465, 5.053911344471881506 ) ) ;
#15570=CARTESIAN_POINT ( 'NONE',  ( 6.340308582316796837, -22.36352608949544418, 4.520995438708343528 ) ) ;
#15574=CARTESIAN_POINT ( 'NONE',  ( 13.82120031190154208, 1.533115751011936867, 6.689942769197355865 ) ) ;
#15583=CARTESIAN_POINT ( 'NONE',  ( 1.720709671993384093, -9.114925383610804843, 1.622645897908254753 ) ) ;
#15585=CARTESIAN_POINT ( 'NONE',  ( -13.09560260347216953, 4.265431475339161338, 5.020858537328734883 ) ) ;
#15586=CARTESIAN_POINT ( 'NONE',  ( 7.746558582316794173, -21.94931252712234482, 5.250000000000000888 ) ) ;
#15587=CARTESIAN_POINT ( 'NONE',  ( -12.62543384439201510, -20.97809085820452424, 4.782403934559678937 ) ) ;
#15589=CARTESIAN_POINT ( 'NONE',  ( 13.27780858231679595, -20.27099543870833642, 2.724438792969431589 ) ) ;
#15590=CARTESIAN_POINT ( 'NONE',  ( 12.53469141768317741, -20.97900456129164581, 3.136473910504570917 ) ) ;
#15591=CARTESIAN_POINT ( 'NONE',  ( -11.40969141768317918, -21.32581373872474373, 5.270995438708348857 ) ) ;
#15593=CARTESIAN_POINT ( 'NONE',  ( 13.37499999999998224, -19.50000000000006040, 4.416666666666682062 ) ) ;
#15595=CARTESIAN_POINT ( 'NONE',  ( -1.819865260185086875, -9.122006307963404836, 1.624464420737683046 ) ) ;
#15600=CARTESIAN_POINT ( 'NONE',  ( -13.10012427866737639, 3.743776072700027324, 6.001983176248468332 ) ) ;
#15601=CARTESIAN_POINT ( 'NONE',  ( -3.173374397671306912, -9.279487642487616483, 2.607523756204581211 ) ) ;
#15602=CARTESIAN_POINT ( 'NONE',  ( -13.58606361274418184, -9.591287556442823714, 5.700679699621803209 ) ) ;
#15606=CARTESIAN_POINT ( 'NONE',  ( 13.12499999999999645, 5.000000000000047073, 3.999999999999996447 ) ) ;
#15610=CARTESIAN_POINT ( 'NONE',  ( -11.49655858231679595, -22.05068747287764452, 0.9999999999999978906 ) ) ;
#15611=CARTESIAN_POINT ( 'NONE',  ( -2.762374231067749708, -9.968169115173667549, 1.841775933429679268 ) ) ;
#15613=CARTESIAN_POINT ( 'NONE',  ( -13.37499999999998224, -20.24999999999991829, 4.333333333333343695 ) ) ;
#15615=CARTESIAN_POINT ( 'NONE',  ( 5.871558582316795949, -19.49999999999998934, 3.449312527122348371 ) ) ;
#15616=CARTESIAN_POINT ( 'NONE',  ( -4.097191417683177406, -22.46490103525075810, 4.479004561291653808 ) ) ;
#15618=CARTESIAN_POINT ( 'NONE',  ( 13.87470602645761986, 4.985154336109792972, 4.916666666666650087 ) ) ;
#15619=CARTESIAN_POINT ( 'NONE',  ( 12.62499999999998401, -20.24999999999998934, 2.439580858552613751 ) ) ;
#15624=CARTESIAN_POINT ( 'NONE',  ( -13.44218742460511073, -16.85703505742523234, 5.544429699623282914 ) ) ;
#15631=CARTESIAN_POINT ( 'NONE',  ( -13.12509927631103501, 5.009931486494128450, 3.999999999999983125 ) ) ;
#15633=CARTESIAN_POINT ( 'NONE',  ( 3.049989092406311109, -8.938202327316346896, 1.769874869409437279 ) ) ;
#15634=LINE ( 'NONE', #20057, #6865 ) ;
#15635=CARTESIAN_POINT ( 'NONE',  ( 13.12529397354238192, 5.014845663890295846, 3.000000000000000000 ) ) ;
#15639=AXIS2_PLACEMENT_3D ( 'NONE', #12829, #6154, #15861 ) ;
#15640=CARTESIAN_POINT ( 'NONE',  ( 6.347191417683176518, -21.53509896474923835, 2.520995438708346192 ) ) ;
#15641=CARTESIAN_POINT ( 'NONE',  ( -12.62499999999998401, -19.49999999999998934, 2.439580858552613751 ) ) ;
#15642=EDGE_CURVE ( 'NONE', #7438, #18614, #701, .T. ) ;
#15643=CARTESIAN_POINT ( 'NONE',  ( -8.215308582316795949, -23.02099543870833998, 3.136473910504556262 ) ) ;
#15644=CARTESIAN_POINT ( 'NONE',  ( -5.690941417683177406, -23.80360840875937001, 5.231925497173365081 ) ) ;
#15647=CARTESIAN_POINT ( 'NONE',  ( 13.37732542738919328, -19.38256591684242025, 4.710253041318374301 ) ) ;
#15653=CARTESIAN_POINT ( 'NONE',  ( 1.717920576997000737, -9.114924032904250240, 2.372645551019823884 ) ) ;
#15662=CARTESIAN_POINT ( 'NONE',  ( -2.742252025265078608, -15.06657917462210605, 2.958534504914692942 ) ) ;
#15665=CARTESIAN_POINT ( 'NONE',  ( 12.62844141768317741, -20.24999999999999289, 3.550687472877664952 ) ) ;
#15668=CARTESIAN_POINT ( 'NONE',  ( -7.190941417683176518, -23.27327832286946219, 4.701595411283453707 ) ) ;
#15670=CARTESIAN_POINT ( 'NONE',  ( 6.246558582316794173, -21.94931252712234482, 5.250000000000000888 ) ) ;
#15672=CARTESIAN_POINT ( 'NONE',  ( -12.66863463945108137, -18.79645070772368953, 6.267287912489321045 ) ) ;
#15675=CARTESIAN_POINT ( 'NONE',  ( 9.434058582316794173, -23.20159541128345992, 4.773278322869455970 ) ) ;
#15679=CARTESIAN_POINT ( 'NONE',  ( 13.43273460392801155, -18.08440250163749496, 6.268067769197452677 ) ) ;
#15686=CARTESIAN_POINT ( 'NONE',  ( -9.340308582316794173, -22.67418626127525982, 5.270995438708342640 ) ) ;
#15689=CARTESIAN_POINT ( 'NONE',  ( 1.513434189748285918, -8.364917468222230923, 1.622643865078341907 ) ) ;
#15692=CARTESIAN_POINT ( 'NONE',  ( -13.08799567112409790, 3.881281391764801025, 5.254907606674271037 ) ) ;
#15693=CARTESIAN_POINT ( 'NONE',  ( 7.090308582316794173, -21.32581373872472597, 1.729004561291657582 ) ) ;
#15694=CARTESIAN_POINT ( 'NONE',  ( -13.89075858682503650, 5.045808634669852744, 6.406973581600956535 ) ) ;
#15697=CARTESIAN_POINT ( 'NONE',  ( 9.246558582316794173, -21.94931252712234482, 5.250000000000000888 ) ) ;
#15698=CARTESIAN_POINT ( 'NONE',  ( 12.90280858231679595, -22.46490103525074034, 2.520995438708341307 ) ) ;
#15699=CARTESIAN_POINT ( 'NONE',  ( -12.44094141768317741, -20.72672167713052715, 2.298404588716546293 ) ) ;
#15701=CARTESIAN_POINT ( 'NONE',  ( 13.42766088059286922, -16.84062553004338625, 4.794749963382423985 ) ) ;
#15702=CARTESIAN_POINT ( 'NONE',  ( -2.786182376113650605, -10.12667130264514626, 1.882483419865550900 ) ) ;
#15708=CIRCLE ( 'NONE', #12036, 0.3750000000000003331 ) ;
#15709=CARTESIAN_POINT ( 'NONE',  ( -12.68288333306630378, -17.32689168014509207, 5.548858176248425700 ) ) ;
#15710=CARTESIAN_POINT ( 'NONE',  ( -1.126276606324276619, -8.364917468222230923, 2.372643865078341019 ) ) ;
#15711=CARTESIAN_POINT ( 'NONE',  ( -13.40382044110196347, -18.79456772435387890, 5.502763032956559108 ) ) ;
#15714=CARTESIAN_POINT ( 'NONE',  ( 11.02780858231679595, -23.72900456129165292, 4.275561207030568411 ) ) ;
#15716=CARTESIAN_POINT ( 'NONE',  ( 13.10026320386584153, 3.000791795219782454, 6.736037912489353019 ) ) ;
#15717=CARTESIAN_POINT ( 'NONE',  ( -6.527808582316795949, -24.47900456129166358, 4.586221378810390270 ) ) ;
#15718=CARTESIAN_POINT ( 'NONE',  ( -2.088806020750596737, -10.42712783963456857, 1.767030719737609168 ) ) ;
#15721=CARTESIAN_POINT ( 'NONE',  ( -13.37503071710846925, -20.24844878602346299, 4.564052989354591361 ) ) ;
#15725=CARTESIAN_POINT ( 'NONE',  ( 6.902808582316795949, -23.08622137881038938, 1.020995438708339309 ) ) ;
#15726=CARTESIAN_POINT ( 'NONE',  ( -6.159691417683175629, -22.36352608949543352, 2.479004561291652031 ) ) ;
#15729=CARTESIAN_POINT ( 'NONE',  ( 13.42074492158312715, -18.68988146005270679, 6.255046935864005064 ) ) ;
#15734=CARTESIAN_POINT ( 'NONE',  ( -13.84504075139246915, 3.487057945321567765, 5.981929699623240282 ) ) ;
#15738=CARTESIAN_POINT ( 'NONE',  ( 2.436080212393455735, -9.483920418190111334, 2.467411194204634839 ) ) ;
#15741=CARTESIAN_POINT ( 'NONE',  ( 1.619022621591187150, -9.114917468222230923, 1.622643865078341463 ) ) ;
#15746=CARTESIAN_POINT ( 'NONE',  ( -12.66615398568989370, -20.44683554016566163, 3.545542780064843136 ) ) ;
#15747=CARTESIAN_POINT ( 'NONE',  ( 6.722191417683176518, -21.02099543870834353, 3.964901035250761208 ) ) ;
#15748=CARTESIAN_POINT ( 'NONE',  ( -13.12529397354238192, 5.014845663890295846, 3.000000000000000000 ) ) ;
#15749=CARTESIAN_POINT ( 'NONE',  ( -11.96530858231679773, -20.97900456129165647, 3.863526089495444626 ) ) ;
#15751=CARTESIAN_POINT ( 'NONE',  ( -11.40969141768318096, -21.32581373872474373, 5.270995438708348857 ) ) ;
#15753=CARTESIAN_POINT ( 'NONE',  ( 13.37503747255156306, -19.49810763614315690, 4.531249681074674740 ) ) ;
#15759=CARTESIAN_POINT ( 'NONE',  ( 1.772926875221950249, -9.883376166076789815, 2.377384427436886494 ) ) ;
#15763=CARTESIAN_POINT ( 'NONE',  ( 7.940941417683176518, -20.72672167713052715, 2.298404588716546293 ) ) ;
#15765=CARTESIAN_POINT ( 'NONE',  ( -2.110348196723525138, -10.58007678474401914, 1.806311064303893099 ) ) ;
#15770=CARTESIAN_POINT ( 'NONE',  ( 6.347191417683176518, -20.91377862118959285, 1.020995438708345082 ) ) ;
#15772=CARTESIAN_POINT ( 'NONE',  ( -10.28469141768318096, -23.77099543870834353, 4.174186261275252718 ) ) ;
#15775=CARTESIAN_POINT ( 'NONE',  ( 13.09030858231679417, -21.01515356694490322, 0.9790045612916562501 ) ) ;
#15777=CARTESIAN_POINT ( 'NONE',  ( -12.62927505847832776, -20.78410954684871825, 5.373974324164845662 ) ) ;
#15780=CARTESIAN_POINT ( 'NONE',  ( 9.527808582316792396, -23.72900456129165647, 4.275561207030568411 ) ) ;
#15789=CARTESIAN_POINT ( 'NONE',  ( -6.340308582316793284, -22.67418626127525982, 5.270995438708342640 ) ) ;
#15791=CARTESIAN_POINT ( 'NONE',  ( 13.15332036705482466, 5.722234611034569873, 3.999999999999985345 ) ) ;
#15792=CARTESIAN_POINT ( 'NONE',  ( 0.2815691515810352930, -9.114917468222230923, 1.622643865078524206 ) ) ;
#15794=CARTESIAN_POINT ( 'NONE',  ( -13.38929389708972195, -18.77815819697223887, 4.753083296715700179 ) ) ;
#15795=CARTESIAN_POINT ( 'NONE',  ( 4.840308582316793284, -22.67418626127525982, 5.270995438708342640 ) ) ;
#15796=CARTESIAN_POINT ( 'NONE',  ( -13.90326467458556969, 5.677366066573198644, 5.457668599364335904 ) ) ;
#15800=CARTESIAN_POINT ( 'NONE',  ( 3.944195004867015353, -21.66042601004066981, 5.025996387692261536 ) ) ;
#15802=CARTESIAN_POINT ( 'NONE',  ( 4.378441417683176518, -22.99999999999999645, 3.449312527122335048 ) ) ;
#15803=CARTESIAN_POINT ( 'NONE',  ( -5.309058582316794173, -23.27327832286945153, 2.298404588716537411 ) ) ;
#15806=CARTESIAN_POINT ( 'NONE',  ( 13.37847682517167947, -19.32442032882675775, 4.733786629989340078 ) ) ;
#15807=CARTESIAN_POINT ( 'NONE',  ( -1.619022621591187150, -9.114917468222230923, 1.622643865078341463 ) ) ;
#15813=CARTESIAN_POINT ( 'NONE',  ( 0.000000000000000000, -8.364917468222230923, 2.372643865078341019 ) ) ;
#15817=CARTESIAN_POINT ( 'NONE',  ( 9.902808582316794173, -22.77556120703056308, 1.770995438708340197 ) ) ;
#15819=CARTESIAN_POINT ( 'NONE',  ( 13.10745701327265778, 3.364079170269163921, 6.743850412489304169 ) ) ;
#15820=CARTESIAN_POINT ( 'NONE',  ( -5.215308582316795949, -24.52099543870834708, 2.515153566944913432 ) ) ;
#15821=CARTESIAN_POINT ( 'NONE',  ( -1.700193846275138032, -9.865151716929458914, 2.372704024825938340 ) ) ;
#15824=CARTESIAN_POINT ( 'NONE',  ( -13.83051420738022763, 3.503467472703414742, 5.232249963382380464 ) ) ;
#15826=CARTESIAN_POINT ( 'NONE',  ( 7.565941417683177406, -23.73192549717336064, 1.696391591240623331 ) ) ;
#15827=CARTESIAN_POINT ( 'NONE',  ( -11.02780858231679595, -22.97900456129165647, 3.964901035250747885 ) ) ;
#15829=CARTESIAN_POINT ( 'NONE',  ( 13.44712222274167246, -17.35782775154002522, 6.283692769197384287 ) ) ;
#15830=CARTESIAN_POINT ( 'NONE',  ( 12.63943061533661982, -19.52125392549825733, 5.470334935344855154 ) ) ;
#15834=CARTESIAN_POINT ( 'NONE',  ( 4.315753587183822404, -21.47141115243053378, 5.558207674221720573 ) ) ;
#15837=ORIENTED_EDGE ( 'NONE', *, *, #12582, .T. ) ;
#15839=CARTESIAN_POINT ( 'NONE',  ( 2.875042468481914248, -11.91375063635796039, 3.091440134965714126 ) ) ;
#15841=CARTESIAN_POINT ( 'NONE',  ( 3.436477319925839602, -9.631595465688135960, 1.947952079262935676 ) ) ;
#15846=CARTESIAN_POINT ( 'NONE',  ( -12.80905858231679417, -23.27327832286945153, 2.298404588716537411 ) ) ;
#15847=PRODUCT_DEFINITION_SHAPE ( 'NONE', 'NONE',  #12257 ) ;
#15848=CARTESIAN_POINT ( 'NONE',  ( 9.065941417683177406, -22.67126532539353789, 2.757051763020445634 ) ) ;
#15849=CARTESIAN_POINT ( 'NONE',  ( -13.12529397354238192, 5.014845663890295846, 4.666666666666619889 ) ) ;
#15850=CARTESIAN_POINT ( 'NONE',  ( -12.99655858231679417, -22.05068747287764452, 1.749999999999998446 ) ) ;
#15851=CARTESIAN_POINT ( 'NONE',  ( -4.378441417683176518, -24.50000000000000000, 3.449312527122335048 ) ) ;
#15853=CARTESIAN_POINT ( 'NONE',  ( 13.09073190589589331, 4.019461247742575516, 5.257453802652931607 ) ) ;
#15861=DIRECTION ( 'NONE',  ( -0.9908228861781570584, 0.1309180808328758994, -0.03362237850931586169 ) ) ;
#15865=CARTESIAN_POINT ( 'NONE',  ( -1.619022621591187150, -9.114917468222230923, 2.372643865078341019 ) ) ;
#15867=CARTESIAN_POINT ( 'NONE',  ( -12.24655858231679240, -21.94931252712234482, 5.250000000000000888 ) ) ;
#15870=CARTESIAN_POINT ( 'NONE',  ( 6.253441417683175629, -21.94931252712233061, 0.9999999999999978906 ) ) ;
#15872=CARTESIAN_POINT ( 'NONE',  ( -8.315941417683177406, -20.79840458871654363, 4.773278322869464851 ) ) ;
#15875=CARTESIAN_POINT ( 'NONE',  ( 6.715308582316794173, -23.77099543870833998, 2.825813738724734847 ) ) ;
#15877=CARTESIAN_POINT ( 'NONE',  ( -12.96597876160390683, -3.780572539034193102, 6.590204579154564257 ) ) ;
#15878=CARTESIAN_POINT ( 'NONE',  ( 5.590308582316794173, -21.32581373872472597, 1.729004561291657582 ) ) ;
#15882=AXIS2_PLACEMENT_3D ( 'NONE', #12527, #9594, #12626 ) ;
#15886=CARTESIAN_POINT ( 'NONE',  ( -12.52780858231679773, -24.47900456129166358, 4.586221378810390270 ) ) ;
#15887=CARTESIAN_POINT ( 'NONE',  ( 12.62888984277510218, -20.05356293986039873, 5.111704976569332537 ) ) ;
#15890=CARTESIAN_POINT ( 'NONE',  ( 2.340131407102140848, -12.21153219924485889, 2.225301406344140531 ) ) ;
#15892=CARTESIAN_POINT ( 'NONE',  ( -13.84485691484488257, 4.227774199669918964, 5.063753864839139140 ) ) ;
#15893=CARTESIAN_POINT ( 'NONE',  ( 9.434058582316794173, -23.20159541128345992, 4.773278322869455970 ) ) ;
#15894=CARTESIAN_POINT ( 'NONE',  ( -13.90439735423812273, 5.734566389025032684, 4.791666666666684726 ) ) ;
#15896=CARTESIAN_POINT ( 'NONE',  ( -10.09030858231679595, -21.01515356694490322, 0.9790045612916562501 ) ) ;
#15899=CARTESIAN_POINT ( 'NONE',  ( 7.472191417683177406, -22.97900456129165292, 3.035098964749240125 ) ) ;
#15900=CARTESIAN_POINT ( 'NONE',  ( -10.09719141768317563, -22.77556120703057729, 5.229004561291656472 ) ) ;
#15902=CARTESIAN_POINT ( 'NONE',  ( 13.83973345681288158, 3.969039569021246550, 5.242263935944164288 ) ) ;
#15910=ADVANCED_FACE ( 'NONE', ( #12450 ), #12239, .T. ) ;
#15912=CARTESIAN_POINT ( 'NONE',  ( -3.594802210173583035, -11.77224174634763898, 3.247712807842289884 ) ) ;
#15915=CARTESIAN_POINT ( 'NONE',  ( -12.62888984277510218, -20.05356293986039873, 5.111704976569332537 ) ) ;
#15916=CARTESIAN_POINT ( 'NONE',  ( 12.90280858231679595, -22.77556120703056308, 1.770995438708340197 ) ) ;
#15918=CARTESIAN_POINT ( 'NONE',  ( 13.11824772738305356, 3.909010232842670796, 6.755569162489314827 ) ) ;
#15919=CARTESIAN_POINT ( 'NONE',  ( -1.882415164465650825, -10.11790622164856224, 2.437616430916333510 ) ) ;
#15922=CARTESIAN_POINT ( 'NONE',  ( -13.84264281492353987, 3.365962153638767607, 5.979325532956542233 ) ) ;
#15925=CARTESIAN_POINT ( 'NONE',  ( 8.222191417683175629, -19.52099543870834353, 4.586221378810406257 ) ) ;
#15926=CARTESIAN_POINT ( 'NONE',  ( -5.503441417683177406, -22.05068747287766229, 4.499999999999999112 ) ) ;
#15928=CARTESIAN_POINT ( 'NONE',  ( 13.48548920624593883, -15.42029508461213716, 6.325359435864005064 ) ) ;
#15929=CARTESIAN_POINT ( 'NONE',  ( 12.62599079447150885, -20.19996487918709249, 4.820256282269618886 ) ) ;
#15937=CARTESIAN_POINT ( 'NONE',  ( 2.583953725994688533, -9.847075946378776479, 2.560676788604062004 ) ) ;
#15939=CARTESIAN_POINT ( 'NONE',  ( 1.897597015127918230, -9.924601616748528699, 1.637971946730535588 ) ) ;
#15945=CARTESIAN_POINT ( 'NONE',  ( -2.534747216115884161, -9.671180236796224960, 2.515503256513427210 ) ) ;
#15946=CARTESIAN_POINT ( 'NONE',  ( 12.05905858231679595, -21.25705176302045274, 4.171265325393551215 ) ) ;
#15947=CARTESIAN_POINT ( 'NONE',  ( -13.08739618700683849, 3.851007443844064237, 5.254256565007597857 ) ) ;
#15948=CARTESIAN_POINT ( 'NONE',  ( -6.902808582316795949, -22.46490103525074034, 2.520995438708341307 ) ) ;
#15950=CARTESIAN_POINT ( 'NONE',  ( -5.315941417683176518, -20.26807450282663225, 5.303608408759377113 ) ) ;
#15951=ORIENTED_EDGE ( 'NONE', *, *, #12473, .T. ) ;
#15952=CARTESIAN_POINT ( 'NONE',  ( 13.08739618700683849, 3.851007443844064237, 5.254256565007597857 ) ) ;
#15963=CARTESIAN_POINT ( 'NONE',  ( 12.25344141768317741, -21.94931252712233061, 1.749999999999998446 ) ) ;
#15965=CARTESIAN_POINT ( 'NONE',  ( -2.645259258103298983, -10.28229522185712241, 2.672449792925449596 ) ) ;
#15967=CARTESIAN_POINT ( 'NONE',  ( -12.15280858231679595, -21.22443879296942626, 5.229004561291660025 ) ) ;
#15970=CARTESIAN_POINT ( 'NONE',  ( 6.534691417683177406, -19.47900456129164581, 2.515153566944927199 ) ) ;
#15972=CARTESIAN_POINT ( 'NONE',  ( -13.12529397354238192, 5.014845663890295846, 4.333333333333382775 ) ) ;
#15973=CARTESIAN_POINT ( 'NONE',  ( -6.722191417683177406, -20.27099543870833998, 4.275561207030583510 ) ) ;
#15975=CARTESIAN_POINT ( 'NONE',  ( 4.934058582316793284, -23.20159541128345992, 4.773278322869455970 ) ) ;
#15977=CARTESIAN_POINT ( 'NONE',  ( -12.81251082758882376, -11.53070320674076576, 6.423537912489145185 ) ) ;
#15979=EDGE_CURVE ( 'NONE', #14618, #2750, #14030, .T. ) ;
#15980=CARTESIAN_POINT ( 'NONE',  ( 7.934058582316792396, -23.20159541128345992, 4.773278322869455970 ) ) ;
#15993=CARTESIAN_POINT ( 'NONE',  ( -4.687312169500632564, -21.51559725698341197, 5.182386163300427562 ) ) ;
#15996=CARTESIAN_POINT ( 'NONE',  ( 1.126276606324276619, -9.864917468222230923, 1.622643865078341907 ) ) ;
#15998=CARTESIAN_POINT ( 'NONE',  ( -13.37499999999998401, -20.24999999999998934, 2.439580858552613751 ) ) ;
#16001=CARTESIAN_POINT ( 'NONE',  ( 6.996558582316793284, -22.05068747287764452, 1.749999999999998446 ) ) ;
#16002=CARTESIAN_POINT ( 'NONE',  ( -12.65816212372154403, -19.32531275206247301, 6.255900543948403225 ) ) ;
#16005=CARTESIAN_POINT ( 'NONE',  ( -6.902808582316795949, -23.08622137881038938, 1.020995438708339309 ) ) ;
#16006=CARTESIAN_POINT ( 'NONE',  ( 6.809058582316794173, -23.27327832286945153, 2.298404588716537411 ) ) ;
#16009=CARTESIAN_POINT ( 'NONE',  ( 5.597191417683177406, -22.46490103525075810, 4.479004561291653808 ) ) ;
#16010=CARTESIAN_POINT ( 'NONE',  ( -7.190941417683176518, -23.27327832286946219, 4.701595411283453707 ) ) ;
#16013=CARTESIAN_POINT ( 'NONE',  ( 13.84137125862932649, 4.051748560779529384, 5.236069268230914453 ) ) ;
#16025=CARTESIAN_POINT ( 'NONE',  ( -3.292205091070697698, -9.639507599131205140, 2.699984073191874057 ) ) ;
#16029=CARTESIAN_POINT ( 'NONE',  ( -12.66849571425264287, -18.05346643024382303, 5.533233176248494978 ) ) ;
#16032=CARTESIAN_POINT ( 'NONE',  ( 12.62499999998404121, -20.24999999996810729, 2.793053905886972998 ) ) ;
#16033=CARTESIAN_POINT ( 'NONE',  ( -1.513434189748285918, -9.864917468222230923, 1.622643865078341907 ) ) ;
#16036=CARTESIAN_POINT ( 'NONE',  ( -13.87470602645761986, 4.985154336109792972, 3.000000000000000000 ) ) ;
#16039=CARTESIAN_POINT ( 'NONE',  ( 4.565941417683176518, -23.73192549717336064, 1.696391591240623331 ) ) ;
#16040=CARTESIAN_POINT ( 'NONE',  ( -10.74655858231679595, -21.94931252712234127, 4.499999999999999112 ) ) ;
#16044=CARTESIAN_POINT ( 'NONE',  ( 12.62527129584495000, -20.98629955982801576, 4.726243163759704657 ) ) ;
#16045=CARTESIAN_POINT ( 'NONE',  ( 12.91308523408712183, -5.701695678577235249, 5.798858176249892082 ) ) ;
#16056=CARTESIAN_POINT ( 'NONE',  ( 1.548630333695928618, -9.864917468222230923, 1.622643865078341907 ) ) ;
#16063=CARTESIAN_POINT ( 'NONE',  ( -11.40280858231679417, -22.77556120703056308, 1.770995438708339975 ) ) ;
#16064=CARTESIAN_POINT ( 'NONE',  ( -1.407845757905374695, -9.114917468222230923, 2.372643865078341019 ) ) ;
#16065=CARTESIAN_POINT ( 'NONE',  ( 11.87155858231679595, -20.99999999999999645, 3.449312527122348371 ) ) ;
#16066=CARTESIAN_POINT ( 'NONE',  ( -13.01365964058540037, 0.1273118495903458325, 5.174178440007729307 ) ) ;
#16067=CARTESIAN_POINT ( 'NONE',  ( -6.434058582316796837, -22.67126532539354855, 4.242948236979545484 ) ) ;
#16069=CARTESIAN_POINT ( 'NONE',  ( -5.034691417683177406, -19.47900456129164581, 2.515153566944927199 ) ) ;
#16072=CARTESIAN_POINT ( 'NONE',  ( 13.84256985046264710, 4.112277448363203192, 5.213861325540929847 ) ) ;
#16082=CARTESIAN_POINT ( 'NONE',  ( 8.878441417683177406, -23.74999999999999645, 3.449312527122335492 ) ) ;
#16085=CARTESIAN_POINT ( 'NONE',  ( -0.5631383031621635116, -9.114917468222230923, 2.372643865078341019 ) ) ;
#16086=CARTESIAN_POINT ( 'NONE',  ( 3.047379876266447685, -13.13734219723468755, 3.405682891496055742 ) ) ;
#16089=CARTESIAN_POINT ( 'NONE',  ( 7.753441417683176518, -21.94931252712233061, 1.749999999999998446 ) ) ;
#16091=CARTESIAN_POINT ( 'NONE',  ( -10.94094141768317741, -21.25705176302044208, 2.828734674606458555 ) ) ;
#16094=CARTESIAN_POINT ( 'NONE',  ( 7.090308582316795061, -21.01515356694490322, 0.9790045612916562501 ) ) ;
#16095=CARTESIAN_POINT ( 'NONE',  ( 13.10192273101908000, 3.834597916462216816, 6.003936301248457674 ) ) ;
#16096=CARTESIAN_POINT ( 'NONE',  ( -12.65457057572495181, -19.50668592589112293, 6.238308001337955488 ) ) ;
#16098=CARTESIAN_POINT ( 'NONE',  ( 8.965308582316794173, -20.22900456129164937, 4.174186261275266929 ) ) ;
#16105=CARTESIAN_POINT ( 'NONE',  ( -11.77780858231679595, -19.52099543870833642, 2.413778621189609286 ) ) ;
#16109=CARTESIAN_POINT ( 'NONE',  ( 2.097836924194969033, -11.64739567274323129, 2.830419876579102212 ) ) ;
#16111=CARTESIAN_POINT ( 'NONE',  ( 13.15498530132288479, 5.764257716805535559, 4.166666666666765551 ) ) ;
#16113=CARTESIAN_POINT ( 'NONE',  ( -13.83890698502169059, 3.927302743594121903, 5.241364546715693074 ) ) ;
#16114=CARTESIAN_POINT ( 'NONE',  ( 10.18405858231679595, -20.26807450282662160, 1.696391591240633101 ) ) ;
#16116=CARTESIAN_POINT ( 'NONE',  ( -13.12175473207386922, 4.086113969730903683, 6.756475741440692850 ) ) ;
#16118=CARTESIAN_POINT ( 'NONE',  ( 5.027808582316793284, -23.72900456129165647, 4.275561207030568411 ) ) ;
#16120=CARTESIAN_POINT ( 'NONE',  ( 7.378441417683177406, -22.99999999999999645, 3.449312527122335048 ) ) ;
#16121=CARTESIAN_POINT ( 'NONE',  ( -7.472191417683176518, -23.72900456129164937, 2.724438792969417378 ) ) ;
#16124=CARTESIAN_POINT ( 'NONE',  ( 13.84501469867711698, 4.235742283194553259, 4.583333333333295734 ) ) ;
#16131=CARTESIAN_POINT ( 'NONE',  ( -13.12529397354238192, 5.014845663890295846, 4.583333333333296622 ) ) ;
#16132=B_SPLINE_CURVE_WITH_KNOTS ( 'NONE', 3,
 ( #4932, #16330, #5554, #16433, #16627, #9948, #10366, #10260, #19490, #16531, #13089, #2414, #6914, #638, #3880, #2304, #18003, #6719, #14761, #8696, #2207, #5240, #2107, #19898, #11519, #15067, #11826, #19584, #18216, #8492, #16742, #13499, #11926, #18319, #6819, #3983, #749, #3782, #11617, #7135, #3675, #10061, #8805, #334, #5455, #14861, #5143, #13188, #17902, #3569, #536, #2004, #8391, #13394, #439, #13284, #19683, #5347, #7027, #11724, #18119, #10160, #8589, #14958, #19798, #2511, #4192, #15379, #20209, #4294, #2932, #18427, #18530, #4091, #10788, #9112, #1163, #15173, #18631, #7335, #8904, #16844, #7543, #1265 ),
 .UNSPECIFIED., .F., .F.,
 ( 4, 2, 2, 2, 2, 2, 2, 2, 2, 2, 2, 2, 2, 2, 2, 2, 2, 2, 2, 2, 2, 2, 2, 2, 2, 2, 2, 2, 2, 2, 2, 2, 2, 2, 2, 2, 2, 2, 2, 2, 2, 4 ),
 ( 0.03313147696908364664, 0.03481082764294501225, 0.05122453910963482154, 0.05943139484297972619, 0.06353482270965217504, 0.06763825057632462390, 0.07081696859385247511, 0.07399568661138032633, 0.08035312264643604263, 0.09306799471654744749, 0.1057828667866588523, 0.1121403028217145825, 0.1153190208392423921, 0.1184977388567702294, 0.1214804596100246548, 0.1244631803632790801, 0.1304286218697878474, 0.1423595048828054654, 0.1662212709088406182, 0.2139448029609110069, 0.3093918670650517289, 0.5002859952733333948, 0.6911801234816148387, 0.7866271875857556717, 0.8343507196378259216, 0.8582124856638611021, 0.8701433686768788034, 0.8761088101833875985, 0.8790915309366421626, 0.8820742516898965047, 0.8853411830926054549, 0.8886081144953145161, 0.8951419773007325276, 0.9082097029115688835, 0.9212774285224050175, 0.9278112913278232510, 0.9310782227305322012, 0.9343451541332412624, 0.9384485819999136558, 0.9425520098665861601, 0.9507588655999309468, 0.9671725770666207422 ),
 .UNSPECIFIED. ) ;
#16133=CARTESIAN_POINT ( 'NONE',  ( -1.906542528716098417, -8.376716462152538512, 1.625674082428238298 ) ) ;
#16138=CARTESIAN_POINT ( 'NONE',  ( -12.63943061533661982, -19.52125392549825733, 5.470334935344855154 ) ) ;
#16139=CARTESIAN_POINT ( 'NONE',  ( 10.74655858231679417, -21.94931252712234482, 5.250000000000000888 ) ) ;
#16141=CARTESIAN_POINT ( 'NONE',  ( 12.62499999999998579, -20.24999999999999289, 3.666666666666653640 ) ) ;
#16142=CARTESIAN_POINT ( 'NONE',  ( -2.067263844777544435, -10.27417889452513933, 1.727750375171331676 ) ) ;
#16146=CARTESIAN_POINT ( 'NONE',  ( -13.37500000000002132, -21.00000000000274269, 4.083333333315724012 ) ) ;
#16148=CARTESIAN_POINT ( 'NONE',  ( 4.003441417683175629, -22.05068747287766229, 6.000000000000001776 ) ) ;
#16150=CARTESIAN_POINT ( 'NONE',  ( -5.871558582316795949, -20.99999999999999645, 3.449312527122348371 ) ) ;
#16152=CARTESIAN_POINT ( 'NONE',  ( 13.90439735423812273, 5.734566389025032684, 4.583333333333295734 ) ) ;
#16153=CARTESIAN_POINT ( 'NONE',  ( 12.72125031657057015, -15.38935901321805133, 5.590524842915047365 ) ) ;
#16157=ORIENTED_EDGE ( 'NONE', *, *, #8649, .T. ) ;
#16164=CARTESIAN_POINT ( 'NONE',  ( 2.155282726790247239, -12.05525952636828357, 2.935167462089139256 ) ) ;
#16165=CARTESIAN_POINT ( 'NONE',  ( 13.87500000000000178, 5.000000000000047962, 2.000000000000000000 ) ) ;
#16170=CARTESIAN_POINT ( 'NONE',  ( -12.52780858231679595, -23.72900456129165647, 4.275561207030568411 ) ) ;
#16171=CARTESIAN_POINT ( 'NONE',  ( -1.655860418491166941, -9.114909740826840689, 2.372641880528837621 ) ) ;
#16173=CARTESIAN_POINT ( 'NONE',  ( -13.09553549038190567, 4.262042264285192950, 5.042530537310905281 ) ) ;
#16174=CARTESIAN_POINT ( 'NONE',  ( -10.55905858231679595, -20.72672167713054137, 4.701595411283463477 ) ) ;
#16175=CARTESIAN_POINT ( 'NONE',  ( -4.565941417683176518, -23.20159541128344927, 2.226721677130534705 ) ) ;
#16177=CARTESIAN_POINT ( 'NONE',  ( 13.83973345681288158, 3.969039569021246550, 5.242263935944164288 ) ) ;
#16185=CARTESIAN_POINT ( 'NONE',  ( 9.909691417683179182, -21.32581373872474373, 5.270995438708348857 ) ) ;
#16189=CARTESIAN_POINT ( 'NONE',  ( -0.9854920305337622199, -9.864917468222230923, 2.372643865078341019 ) ) ;
#16191=CARTESIAN_POINT ( 'NONE',  ( -9.527808582316794173, -23.72900456129165292, 4.275561207030568411 ) ) ;
#16194=CARTESIAN_POINT ( 'NONE',  ( 7.097191417683177406, -22.77556120703057729, 5.229004561291655584 ) ) ;
#16196=CARTESIAN_POINT ( 'NONE',  ( -11.12844141768317741, -20.99999999999999645, 3.550687472877664952 ) ) ;
#16198=CARTESIAN_POINT ( 'NONE',  ( 10.37155858231679595, -19.49999999999998934, 3.449312527122348371 ) ) ;
#16199=CARTESIAN_POINT ( 'NONE',  ( 12.65051119073526564, -18.96168486786632457, 5.513701926248478102 ) ) ;
#16200=CARTESIAN_POINT ( 'NONE',  ( -13.15384296923648400, 5.706569946443514674, 5.461568745250741763 ) ) ;
#16207=CARTESIAN_POINT ( 'NONE',  ( 12.63268481240007546, -20.15932789777624023, 3.549899454067339200 ) ) ;
#16209=CARTESIAN_POINT ( 'NONE',  ( -11.96530858231679773, -19.47900456129164937, 4.484846433055089676 ) ) ;
#16210=CARTESIAN_POINT ( 'NONE',  ( 12.72125031657057015, -15.38935901321805133, 5.590524842915047365 ) ) ;
#16213=CARTESIAN_POINT ( 'NONE',  ( 12.64323021897839006, -19.32937394158751943, 5.504219675487169283 ) ) ;
#16215=CARTESIAN_POINT ( 'NONE',  ( -13.83411111208379474, 3.685111160228107252, 5.236156213382356484 ) ) ;
#16216=CARTESIAN_POINT ( 'NONE',  ( 8.027808582316795949, -24.47900456129166358, 4.586221378810390270 ) ) ;
#16217=CARTESIAN_POINT ( 'NONE',  ( -13.04271272860988340, 0.09449279482665236263, 6.673537912489449830 ) ) ;
#16218=CARTESIAN_POINT ( 'NONE',  ( -10.37844141768317741, -24.50000000000000000, 3.449312527122335048 ) ) ;
#16223=CARTESIAN_POINT ( 'NONE',  ( 7.371558582316795949, -20.99999999999999645, 3.449312527122348371 ) ) ;
#16224=CARTESIAN_POINT ( 'NONE',  ( -6.628441417683176518, -20.24999999999999289, 3.550687472877664952 ) ) ;
#16227=CARTESIAN_POINT ( 'NONE',  ( 13.84497512400090891, 4.233743762047977199, 5.032110966142367303 ) ) ;
#16229=DIRECTION ( 'NONE',  ( 0.000000000000000000, 0.000000000000000000, 1.000000000000000000 ) ) ;
#16234=CARTESIAN_POINT ( 'NONE',  ( -13.12503131243110843, 5.001581277770153378, 5.166347330538456184 ) ) ;
#16237=CARTESIAN_POINT ( 'NONE',  ( -12.62745083560477966, -20.12623280195927933, 5.001038150054709419 ) ) ;
#16238=CARTESIAN_POINT ( 'NONE',  ( 6.527808582316794173, -23.72900456129165292, 4.275561207030568411 ) ) ;
#16240=CARTESIAN_POINT ( 'NONE',  ( 12.63819864697926754, -19.58346832754827105, 5.450273968536036406 ) ) ;
#16241=CARTESIAN_POINT ( 'NONE',  ( -1.126276606324276619, -9.114917468222230923, 2.372643865078341019 ) ) ;
#16243=CARTESIAN_POINT ( 'NONE',  ( -13.86470821076586368, 4.480264643675554659, 5.874551681240599343 ) ) ;
#16245=CARTESIAN_POINT ( 'NONE',  ( 10.37844141768317741, -23.74999999999999645, 3.449312527122335492 ) ) ;
#16246=CARTESIAN_POINT ( 'NONE',  ( -10.55905858231679595, -21.25705176302045274, 4.171265325393551215 ) ) ;
#16248=CARTESIAN_POINT ( 'NONE',  ( 13.90258797164900884, 5.643192568275169130, 5.568788873356017355 ) ) ;
#16249=CARTESIAN_POINT ( 'NONE',  ( 13.10756170493883310, 4.119366099410778581, 6.001761809183453700 ) ) ;
#16250=CARTESIAN_POINT ( 'NONE',  ( -13.33402348762467327, -20.05346030977060678, 3.454433009287248613 ) ) ;
#16259=CARTESIAN_POINT ( 'NONE',  ( 1.863950040896528604, -9.995453039732266731, 2.406168007552154098 ) ) ;
#16264=FACE_OUTER_BOUND ( 'NONE', #8988, .T. ) ;
#16265=CARTESIAN_POINT ( 'NONE',  ( -3.342893013439646843, -9.383962644129466568, 1.884355023724047173 ) ) ;
#16267=CARTESIAN_POINT ( 'NONE',  ( -12.62499999999998224, -19.49999999999991473, 4.333333333333343695 ) ) ;
#16268=CARTESIAN_POINT ( 'NONE',  ( -13.09030858231679417, -21.32581373872472597, 1.729004561291657582 ) ) ;
#16269=CARTESIAN_POINT ( 'NONE',  ( -8.878441417683177406, -23.74999999999999645, 3.449312527122335492 ) ) ;
#16271=CARTESIAN_POINT ( 'NONE',  ( 13.84500676459759383, 4.235341612176667603, 5.016097456370799179 ) ) ;
#16272=CARTESIAN_POINT ( 'NONE',  ( -4.315753587183822404, -21.47141115243053378, 5.558207674221720573 ) ) ;
#16281=CARTESIAN_POINT ( 'NONE',  ( 6.534691417683176518, -20.22900456129164581, 2.825813738724748170 ) ) ;
#16283=CARTESIAN_POINT ( 'NONE',  ( -1.548630333695928618, -9.864917468222230923, 2.372643865078341019 ) ) ;
#16284=CARTESIAN_POINT ( 'NONE',  ( 2.579281110863027582, -9.822567596814183233, 2.554382554832406615 ) ) ;
#16285=CARTESIAN_POINT ( 'NONE',  ( -8.777808582316792396, -20.27099543870833642, 2.724438792969431589 ) ) ;
#16288=CARTESIAN_POINT ( 'NONE',  ( 10.75344141768317741, -21.94931252712233061, 1.749999999999998446 ) ) ;
#16290=CARTESIAN_POINT ( 'NONE',  ( -12.15969141768317918, -22.36352608949543352, 2.479004561291652031 ) ) ;
#16292=CARTESIAN_POINT ( 'NONE',  ( 10.27780858231679595, -19.52099543870833642, 2.413778621189609286 ) ) ;
#16293=CARTESIAN_POINT ( 'NONE',  ( 13.05696142222617695, 1.564051822406025583, 5.955108176248398166 ) ) ;
#16294=CARTESIAN_POINT ( 'NONE',  ( -12.63943061533661982, -19.52125392549825733, 5.470334935344855154 ) ) ;
#16301=( NAMED_UNIT ( * ) PLANE_ANGLE_UNIT ( ) SI_UNIT ( $, .RADIAN. ) );
#16302=ORIENTED_EDGE ( 'NONE', *, *, #5151, .F. ) ;
#16309=CARTESIAN_POINT ( 'NONE',  ( 12.62499999999998224, -20.25000000000006395, 4.416666666666681174 ) ) ;
#16310=CARTESIAN_POINT ( 'NONE',  ( 4.647268150594000780, -21.56957941601164563, 4.994152606344886891 ) ) ;
#16311=CARTESIAN_POINT ( 'NONE',  ( -13.37499999999998224, -20.25000000000006395, 4.416666666666681174 ) ) ;
#16312=CARTESIAN_POINT ( 'NONE',  ( 11.96530858231679773, -19.47900456129164937, 4.484846433055089676 ) ) ;
#16313=CARTESIAN_POINT ( 'NONE',  ( -13.12035191997235906, 4.015271958632619764, 6.757839745787993735 ) ) ;
#16314=CARTESIAN_POINT ( 'NONE',  ( -6.246558582316795949, -21.94931252712234127, 6.000000000000001776 ) ) ;
#16317=CARTESIAN_POINT ( 'NONE',  ( 10.46530858231679595, -20.97900456129165647, 3.863526089495444626 ) ) ;
#16318=CARTESIAN_POINT ( 'NONE',  ( -4.940941417683177406, -20.72672167713052715, 2.298404588716546293 ) ) ;
#16323=CARTESIAN_POINT ( 'NONE',  ( 13.37499999999998224, -20.24999999999998934, 4.166666666666636765 ) ) ;
#16330=CARTESIAN_POINT ( 'NONE',  ( 13.37499999999995204, -20.24999999999992184, 3.465895369911768054 ) ) ;
#16333=CARTESIAN_POINT ( 'NONE',  ( 2.076833265075072266, -8.407161531158021006, 2.383492984350220389 ) ) ;
#16336=CARTESIAN_POINT ( 'NONE',  ( 1.407845757905374695, -9.114917468222230923, 1.622643865078341463 ) ) ;
#16337=CARTESIAN_POINT ( 'NONE',  ( -13.09892531043291086, 3.683228176858501790, 6.000681092915118420 ) ) ;
#16338=CARTESIAN_POINT ( 'NONE',  ( 4.746558582316793284, -21.94931252712234482, 5.250000000000000888 ) ) ;
#16340=CARTESIAN_POINT ( 'NONE',  ( 13.12529418130016445, 5.014856155665242454, 4.958178834604180629 ) ) ;
#16341=CARTESIAN_POINT ( 'NONE',  ( -2.645259258103298983, -10.28229522185712241, 2.672449792925449596 ) ) ;
#16343=CARTESIAN_POINT ( 'NONE',  ( 11.31594141768317741, -20.79840458871654363, 4.773278322869464851 ) ) ;
#16344=CARTESIAN_POINT ( 'NONE',  ( -9.434058582316795949, -22.67126532539354855, 4.242948236979545484 ) ) ;
#16346=CARTESIAN_POINT ( 'NONE',  ( 13.82120031190154208, 1.533115751011936867, 6.689942769197355865 ) ) ;
#16347=CARTESIAN_POINT ( 'NONE',  ( 12.83635126708105823, -9.576761012430582198, 5.715524842913705328 ) ) ;
#16349=CARTESIAN_POINT ( 'NONE',  ( -13.37327929115833491, -20.24999999560066399, 3.449077790995343840 ) ) ;
#16357=CARTESIAN_POINT ( 'NONE',  ( 1.513434189748285918, -9.864917468222230923, 1.622643865078341907 ) ) ;
#16362=CARTESIAN_POINT ( 'NONE',  ( 13.24898903296832486, -20.53044634143503444, 3.466065607697936368 ) ) ;
#16364=CARTESIAN_POINT ( 'NONE',  ( -7.840308582316794173, -22.67418626127525982, 5.270995438708342640 ) ) ;
#16365=CARTESIAN_POINT ( 'NONE',  ( -1.548630333695928618, -8.364917468222230923, 2.372643865078341019 ) ) ;
#16367=CARTESIAN_POINT ( 'NONE',  ( -12.70672377255832686, -15.37294948583620346, 4.840845106674187548 ) ) ;
#16368=CARTESIAN_POINT ( 'NONE',  ( -7.184058582316794173, -20.79840458871652942, 2.226721677130544030 ) ) ;
#16370=CARTESIAN_POINT ( 'NONE',  ( -7.940941417683176518, -20.72672167713052715, 2.298404588716546293 ) ) ;
#16372=CARTESIAN_POINT ( 'NONE',  ( 13.40368151590352497, -18.05158344687463412, 4.768708296715732153 ) ) ;
#16378=CARTESIAN_POINT ( 'NONE',  ( -13.39296152110871851, -19.34294318400601753, 5.489418334493660012 ) ) ;
#16381=CARTESIAN_POINT ( 'NONE',  ( 6.440941417683176518, -20.72672167713052715, 2.298404588716546293 ) ) ;
#16386=CARTESIAN_POINT ( 'NONE',  ( -7.184058582316794173, -20.79840458871652942, 2.226721677130544030 ) ) ;
#16389=CARTESIAN_POINT ( 'NONE',  ( 8.034691417683175629, -20.22900456129164581, 2.825813738724747726 ) ) ;
#16391=CARTESIAN_POINT ( 'NONE',  ( -12.06594141768317741, -22.67126532539353789, 2.757051763020445634 ) ) ;
#16392=CARTESIAN_POINT ( 'NONE',  ( -8.027808582316795949, -24.47900456129166358, 4.586221378810390270 ) ) ;
#16395=CARTESIAN_POINT ( 'NONE',  ( 12.62562019941893432, -20.21867992933967173, 4.757612834768309540 ) ) ;
#16396=CARTESIAN_POINT ( 'NONE',  ( -13.13728495444130751, 4.870390199291127153, 6.548325014280736767 ) ) ;
#16406=CARTESIAN_POINT ( 'NONE',  ( 12.75111466187344966, -19.96946164605619245, 3.533920058977110479 ) ) ;
#16408=DIRECTION ( 'NONE',  ( -1.000000000000000000, 0.000000000000000000, 0.000000000000000000 ) ) ;
#16413=CARTESIAN_POINT ( 'NONE',  ( 12.74043380832193684, -14.42059267975384529, 5.611358176248560703 ) ) ;
#16415=CARTESIAN_POINT ( 'NONE',  ( 11.30905858231679595, -23.80360840875935935, 1.768074502826626260 ) ) ;
#16416=CARTESIAN_POINT ( 'NONE',  ( -12.62500016093973620, -20.24999187254239175, 4.532396751752561848 ) ) ;
#16417=CARTESIAN_POINT ( 'NONE',  ( -10.75344141768317741, -21.94931252712233061, 0.9999999999999978906 ) ) ;
#16420=CARTESIAN_POINT ( 'NONE',  ( 12.05905858231679595, -21.25705176302045274, 4.171265325393551215 ) ) ;
#16421=CARTESIAN_POINT ( 'NONE',  ( -4.097191417683176518, -22.77556120703057729, 5.229004561291656472 ) ) ;
#16424=CARTESIAN_POINT ( 'NONE',  ( 13.86106797245302147, 4.296432608878145487, 5.947261916831099171 ) ) ;
#16433=CARTESIAN_POINT ( 'NONE',  ( 13.37499999999998579, -20.24999999999999289, 3.666666666666653640 ) ) ;
#16435=CARTESIAN_POINT ( 'NONE',  ( 3.882031223148668886, -13.81156101447257889, 3.771450735391772557 ) ) ;
#16439=CARTESIAN_POINT ( 'NONE',  ( -12.62599452815238443, -19.44977632830967806, 4.656396506304353977 ) ) ;
#16440=CARTESIAN_POINT ( 'NONE',  ( 8.684058582316794173, -20.79840458871652942, 2.226721677130544030 ) ) ;
#16442=CARTESIAN_POINT ( 'NONE',  ( 12.64931222250080545, -19.02223276370786209, 5.512399842915133519 ) ) ;
#16444=B_SPLINE_CURVE_WITH_KNOTS ( 'NONE', 3,
 ( #16655, #13313, #19714, #16555, #8615, #11851 ),
 .UNSPECIFIED., .F., .F.,
 ( 4, 2, 4 ),
 ( 0.000000000000000000, 0.2500000000000000000, 0.5000000000000000000 ),
 .UNSPECIFIED. ) ;
#16445=CARTESIAN_POINT ( 'NONE',  ( -2.594671182134835163, -9.923034775318452461, 2.580184533305832861 ) ) ;
#16446=CARTESIAN_POINT ( 'NONE',  ( 12.24655858231679595, -21.94931252712234127, 4.499999999999999112 ) ) ;
#16447=CARTESIAN_POINT ( 'NONE',  ( 8.222191417683175629, -20.27099543870833998, 4.275561207030583510 ) ) ;
#16448=CARTESIAN_POINT ( 'NONE',  ( -10.09030858231679595, -21.63647391050454871, 2.479004561291657804 ) ) ;
#16450=CARTESIAN_POINT ( 'NONE',  ( 13.07148796623841847, 1.547642295024179493, 6.704787912489258872 ) ) ;
#16451=CARTESIAN_POINT ( 'NONE',  ( 12.62499999998404299, -19.49999999996810729, 2.793053905886972998 ) ) ;
#16452=CARTESIAN_POINT ( 'NONE',  ( -12.90166454282617536, -19.87494034644570107, 3.513414777791785681 ) ) ;
#16455=EDGE_LOOP ( 'NONE', ( #300, #19064, #10123, #18735, #14906, #16302 ) ) ;
#16461=CARTESIAN_POINT ( 'NONE',  ( 1.710927537542899612, -9.866086492083725901, 2.372944093759576933 ) ) ;
#16466=CARTESIAN_POINT ( 'NONE',  ( -1.904508877737772998, -9.138371295333994837, 2.378667276417936627 ) ) ;
#16467=CARTESIAN_POINT ( 'NONE',  ( -6.059058582316793284, -20.72672167713054137, 4.701595411283463477 ) ) ;
#16468=CARTESIAN_POINT ( 'NONE',  ( -3.257364212367626966, -9.501732542047829355, 2.664600686199549706 ) ) ;
#16470=CARTESIAN_POINT ( 'NONE',  ( -13.37847682517167947, -19.32442032882675775, 4.733786629989340078 ) ) ;
#16471=CARTESIAN_POINT ( 'NONE',  ( -10.18405858231679417, -20.79840458871652942, 2.226721677130544030 ) ) ;
#16473=CARTESIAN_POINT ( 'NONE',  ( -5.503441417683176518, -22.05068747287765873, 5.250000000000000888 ) ) ;
#16475=CARTESIAN_POINT ( 'NONE',  ( 13.84501474873290938, 4.235744811019327649, 4.974109985360144037 ) ) ;
#16484=CARTESIAN_POINT ( 'NONE',  ( 4.190941417683176518, -23.27327832286946219, 4.701595411283453707 ) ) ;
#16487=CARTESIAN_POINT ( 'NONE',  ( 2.875042468481914248, -11.91375063635796039, 3.091440134965714126 ) ) ;
#16488=CARTESIAN_POINT ( 'NONE',  ( -4.934058582316793284, -23.20159541128345992, 4.773278322869455970 ) ) ;
#16489=CARTESIAN_POINT ( 'NONE',  ( 13.90411326029870409, 5.720219645086723759, 5.230514352905474063 ) ) ;
#16491=CARTESIAN_POINT ( 'NONE',  ( 7.378441417683176518, -23.74999999999999645, 3.449312527122335492 ) ) ;
#16493=CARTESIAN_POINT ( 'NONE',  ( -6.534691417683177406, -20.97900456129164581, 3.136473910504570917 ) ) ;
#16494=CARTESIAN_POINT ( 'NONE',  ( -8.871558582316795949, -19.49999999999998934, 3.449312527122348371 ) ) ;
#16496=CARTESIAN_POINT ( 'NONE',  ( 12.83635126708105823, -9.576761012430582198, 5.715524842913705328 ) ) ;
#16497=CARTESIAN_POINT ( 'NONE',  ( -12.64195242771744709, -19.39390240027112000, 5.496549442168085164 ) ) ;
#16507=CARTESIAN_POINT ( 'NONE',  ( 13.10756170493883310, 4.119366099410778581, 6.001761809183453700 ) ) ;
#16509=CARTESIAN_POINT ( 'NONE',  ( -1.852280067228949445, -9.126254559850970338, 1.625555456689752321 ) ) ;
#16513=CARTESIAN_POINT ( 'NONE',  ( 12.62888984277510218, -20.05356293986039873, 5.111704976569332537 ) ) ;
#16515=CARTESIAN_POINT ( 'NONE',  ( 11.87155858231679595, -19.49999999999998934, 3.449312527122348371 ) ) ;
#16516=CARTESIAN_POINT ( 'NONE',  ( -12.62562019941893432, -20.21867992933967173, 4.757612834768309540 ) ) ;
#16517=CARTESIAN_POINT ( 'NONE',  ( -4.753441417683176518, -21.94931252712233061, 0.9999999999999978906 ) ) ;
#16520=CARTESIAN_POINT ( 'NONE',  ( 10.27780858231679595, -21.02099543870833998, 3.035098964749253003 ) ) ;
#16524=CARTESIAN_POINT ( 'NONE',  ( 13.37499999999998401, -20.99999999999998934, 2.439580858552613751 ) ) ;
#16527=EDGE_CURVE ( 'NONE', #1939, #8463, #5730, .T. ) ;
#16531=CARTESIAN_POINT ( 'NONE',  ( 13.37499999999998224, -20.25000000000006395, 4.416666666666681174 ) ) ;
#16533=CARTESIAN_POINT ( 'NONE',  ( 1.548630333695928618, -8.364917468222230923, 2.372643865078341019 ) ) ;
#16536=CARTESIAN_POINT ( 'NONE',  ( -12.89855869007488209, -5.685286151195387383, 5.049178440009032265 ) ) ;
#16537=CARTESIAN_POINT ( 'NONE',  ( 7.746558582316794173, -21.94931252712234482, 5.250000000000000888 ) ) ;
#16539=CARTESIAN_POINT ( 'NONE',  ( 13.10557919622060652, 4.019249409169220577, 6.007898877577752650 ) ) ;
#16541=CARTESIAN_POINT ( 'NONE',  ( 9.809058582316795949, -22.74294823697954016, 2.828734674606448785 ) ) ;
#16542=CARTESIAN_POINT ( 'NONE',  ( 7.940941417683176518, -20.72672167713052715, 2.298404588716546293 ) ) ;
#16543=CARTESIAN_POINT ( 'NONE',  ( -10.46530858231679417, -20.22900456129164937, 4.174186261275266929 ) ) ;
#16545=CARTESIAN_POINT ( 'NONE',  ( 12.65986935584910000, -19.23909752961862907, 6.257782094979345899 ) ) ;
#16546=CARTESIAN_POINT ( 'NONE',  ( 12.63298722613685676, -19.09664508008815531, 4.760766981674283471 ) ) ;
#16555=CARTESIAN_POINT ( 'NONE',  ( -3.984239023773644028, -21.55980365857980630, 5.395836504137947465 ) ) ;
#16556=CARTESIAN_POINT ( 'NONE',  ( 2.109407804498405703, -9.207748739546751438, 2.396484790045401603 ) ) ;
#16559=CARTESIAN_POINT ( 'NONE',  ( 13.18792642815267335, -20.57543385444909845, 3.474652748137723179 ) ) ;
#16561=CARTESIAN_POINT ( 'NONE',  ( -7.934058582316792396, -23.20159541128345992, 4.773278322869455970 ) ) ;
#16562=CARTESIAN_POINT ( 'NONE',  ( -3.365018999794965548, -10.14078633184679923, 2.828722465802024910 ) ) ;
#16564=CARTESIAN_POINT ( 'NONE',  ( -13.37499999999998401, -19.49999999999998934, 3.146526952850934755 ) ) ;
#16565=CARTESIAN_POINT ( 'NONE',  ( -6.902808582316793284, -22.77556120703056308, 1.770995438708339975 ) ) ;
#16566=CARTESIAN_POINT ( 'NONE',  ( -6.628441417683176518, -20.24999999999999289, 3.550687472877664952 ) ) ;
#16568=CARTESIAN_POINT ( 'NONE',  ( 13.41341218697771609, -18.31018455762212227, 5.513179699623425023 ) ) ;
#16574=CARTESIAN_POINT ( 'NONE',  ( -13.37327929115833491, -20.24999999560066399, 3.449077790995343840 ) ) ;
#16576=CARTESIAN_POINT ( 'NONE',  ( 7.565941417683176518, -23.20159541128344927, 2.226721677130534705 ) ) ;
#16579=CARTESIAN_POINT ( 'NONE',  ( 1.513434189748285696, -9.114917468222230923, 2.372643865078341019 ) ) ;
#16580=CARTESIAN_POINT ( 'NONE',  ( -5.027808582316793284, -23.72900456129165292, 4.275561207030568411 ) ) ;
#16582=CARTESIAN_POINT ( 'NONE',  ( 12.62527129584495000, -20.98629955982801576, 4.726243163759704657 ) ) ;
#16584=CARTESIAN_POINT ( 'NONE',  ( 12.34719141768317741, -21.53509896474923835, 2.520995438708346192 ) ) ;
#16585=CARTESIAN_POINT ( 'NONE',  ( -12.64511805349267526, -19.23403829861753422, 5.507852591554869726 ) ) ;
#16586=CARTESIAN_POINT ( 'NONE',  ( -7.940941417683175629, -21.25705176302044208, 2.828734674606458555 ) ) ;
#16587=CARTESIAN_POINT ( 'NONE',  ( -7.746558582316795949, -21.94931252712234127, 6.000000000000001776 ) ) ;
#16589=CARTESIAN_POINT ( 'NONE',  ( 12.62500797102436678, -19.49959746326937093, 4.516621614626514791 ) ) ;
#16590=CARTESIAN_POINT ( 'NONE',  ( -12.79798428357658047, -11.51429367935891790, 5.673858176248284479 ) ) ;
#16596=CARTESIAN_POINT ( 'NONE',  ( 12.81218474072258040, -19.92450197877212048, 3.525331579139530547 ) ) ;
#16599=CARTESIAN_POINT ( 'NONE',  ( 12.65051119073526564, -18.96168486786632457, 5.513701926248478102 ) ) ;
#16600=CARTESIAN_POINT ( 'NONE',  ( -2.762374231067749708, -9.968169115173667549, 1.841775933429679268 ) ) ;
#16605=CARTESIAN_POINT ( 'NONE',  ( 5.684058582316795949, -20.26807450282662160, 1.696391591240633101 ) ) ;
#16606=CARTESIAN_POINT ( 'NONE',  ( -13.09892531043291086, 3.683228176858501790, 6.000681092915118420 ) ) ;
#16607=CARTESIAN_POINT ( 'NONE',  ( -6.628441417683177406, -19.49999999999998934, 3.550687472877664952 ) ) ;
#16612=CARTESIAN_POINT ( 'NONE',  ( -13.75871503850933841, -0.8723905552644914962, 5.888179699623941943 ) ) ;
#16613=CARTESIAN_POINT ( 'NONE',  ( 8.590308582316797725, -21.63647391050454871, 2.479004561291657804 ) ) ;
#16616=ORIENTED_EDGE ( 'NONE', *, *, #7561, .T. ) ;
#16618=CARTESIAN_POINT ( 'NONE',  ( 13.41820805991576826, -18.06799297425606454, 5.518388032956592859 ) ) ;
#16627=CARTESIAN_POINT ( 'NONE',  ( 13.37500000000002132, -20.24999999999450040, 3.833333333368183382 ) ) ;
#16629=CARTESIAN_POINT ( 'NONE',  ( 2.171407406650392780, -8.432416083433171394, 2.389978857884845986 ) ) ;
#16631=CARTESIAN_POINT ( 'NONE',  ( -12.62499999999998401, -19.49999999999998934, 3.146526952850934755 ) ) ;
#16632=CARTESIAN_POINT ( 'NONE',  ( 7.934058582316792396, -23.20159541128345992, 4.773278322869455970 ) ) ;
#16634=CARTESIAN_POINT ( 'NONE',  ( 13.00900269284621302, -0.8578640112522492034, 5.903024842915844062 ) ) ;
#16636=AXIS2_PLACEMENT_3D ( 'NONE', #6979, #18070, #4047 ) ;
#16638=CARTESIAN_POINT ( 'NONE',  ( 7.371558582316795949, -20.99999999999999645, 3.449312527122348371 ) ) ;
#16639=CARTESIAN_POINT ( 'NONE',  ( 11.59719141768317563, -22.77556120703057729, 5.229004561291655584 ) ) ;
#16640=CARTESIAN_POINT ( 'NONE',  ( -9.340308582316794173, -22.67418626127525982, 5.270995438708342640 ) ) ;
#16642=CARTESIAN_POINT ( 'NONE',  ( 13.10745701327265778, 3.364079170269163921, 6.743850412489304169 ) ) ;
#16644=CARTESIAN_POINT ( 'NONE',  ( 12.64917329730235096, -18.27924848622803466, 4.778345106674467324 ) ) ;
#16655=CARTESIAN_POINT ( 'NONE',  ( -4.315753587183822404, -21.47141115243053378, 5.558207674221720573 ) ) ;
#16656=CARTESIAN_POINT ( 'NONE',  ( 2.594671182134835163, -9.923034775318452461, 2.580184533305832861 ) ) ;
#16661=CARTESIAN_POINT ( 'NONE',  ( -1.717920576997000737, -9.114924032904250240, 2.372645551019823884 ) ) ;
#16662=CARTESIAN_POINT ( 'NONE',  ( -6.152808582316793284, -21.22443879296942626, 5.229004561291659137 ) ) ;
#16663=CARTESIAN_POINT ( 'NONE',  ( -1.643076795806035717, -8.364903549957356077, 2.372640290589878909 ) ) ;
#16667=CARTESIAN_POINT ( 'NONE',  ( -13.41806913471718588, -17.32500869677464550, 4.784333296715663764 ) ) ;
#16668=CARTESIAN_POINT ( 'NONE',  ( -6.152808582316793284, -21.22443879296942626, 5.229004561291659137 ) ) ;
#16669=CARTESIAN_POINT ( 'NONE',  ( 12.71530858231679417, -24.52099543870834708, 2.515153566944913432 ) ) ;
#16670=CARTESIAN_POINT ( 'NONE',  ( -10.94094141768317741, -21.25705176302044208, 2.828734674606458555 ) ) ;
#16673=CARTESIAN_POINT ( 'NONE',  ( 13.38450946332969771, -19.76977210184853462, 5.359796180098093998 ) ) ;
#16679=CARTESIAN_POINT ( 'NONE',  ( -13.37500000000002132, -20.24999999999450040, 3.833333333368183382 ) ) ;
#16682=CARTESIAN_POINT ( 'NONE',  ( 4.097191417683176518, -22.77556120703057729, 5.229004561291656472 ) ) ;
#16686=CARTESIAN_POINT ( 'NONE',  ( 2.171407406650392780, -8.432416083433171394, 2.389978857884845986 ) ) ;
#16687=CARTESIAN_POINT ( 'NONE',  ( -6.340308582316794173, -22.67418626127525982, 5.270995438708342640 ) ) ;
#16690=CARTESIAN_POINT ( 'NONE',  ( 12.65816212372154403, -19.32531275206247301, 6.255900543948403225 ) ) ;
#16693=CARTESIAN_POINT ( 'NONE',  ( 4.565941417683176518, -23.20159541128344927, 2.226721677130534705 ) ) ;
#16694=FACE_OUTER_BOUND ( 'NONE', #5231, .T. ) ;
#16695=CARTESIAN_POINT ( 'NONE',  ( -8.315941417683177406, -21.32873467460645145, 4.242948236979555254 ) ) ;
#16696=CARTESIAN_POINT ( 'NONE',  ( -12.53469141768317741, -19.47900456129164581, 2.515153566944927199 ) ) ;
#16698=CARTESIAN_POINT ( 'NONE',  ( 12.62499999999998224, -19.49999999999998934, 4.291666666666699825 ) ) ;
#16699=CARTESIAN_POINT ( 'NONE',  ( -13.10756170493883310, 4.119366099410778581, 6.001761809183453700 ) ) ;
#16712=CARTESIAN_POINT ( 'NONE',  ( -3.347120161770001268, -14.10934257735911146, 2.905312006771028077 ) ) ;
#16716=CARTESIAN_POINT ( 'NONE',  ( -7.559058582316794173, -20.72672167713054137, 4.701595411283463477 ) ) ;
#16719=CARTESIAN_POINT ( 'NONE',  ( 9.440941417683177406, -20.19639159124061933, 1.768074502826635586 ) ) ;
#16720=CARTESIAN_POINT ( 'NONE',  ( -12.69247507894198712, -16.84250851341299082, 5.559274842915185033 ) ) ;
#16722=CARTESIAN_POINT ( 'NONE',  ( -4.378441417683176518, -24.50000000000000000, 3.449312527122335048 ) ) ;
#16726=CARTESIAN_POINT ( 'NONE',  ( 10.65280858231679240, -21.22443879296942626, 5.229004561291659137 ) ) ;
#16728=CARTESIAN_POINT ( 'NONE',  ( -13.88684657106908205, 4.848251838987907014, 6.535242036940271504 ) ) ;
#16730=CARTESIAN_POINT ( 'NONE',  ( 13.37155858231679417, -20.24999999999999289, 3.449312527122348371 ) ) ;
#16734=CARTESIAN_POINT ( 'NONE',  ( 13.85163507668220539, 3.820071372449974412, 5.989091157956555556 ) ) ;
#16737=EDGE_CURVE ( 'NONE', #8228, #7887, #20335, .T. ) ;
#16742=CARTESIAN_POINT ( 'NONE',  ( 13.39722611581222189, -19.12758115148224647, 5.495601574623241170 ) ) ;
#16745=CARTESIAN_POINT ( 'NONE',  ( 1.728780693989796724, -8.364929292255887106, 2.372646901726390478 ) ) ;
#16747=CARTESIAN_POINT ( 'NONE',  ( -12.63298722613685676, -19.09664508008815531, 4.760766981674283471 ) ) ;
#16749=CARTESIAN_POINT ( 'NONE',  ( 11.59030858231679417, -21.32581373872472597, 1.729004561291657582 ) ) ;
#16750=CARTESIAN_POINT ( 'NONE',  ( -13.37500000000002132, -21.00000000000274269, 4.083333333315724012 ) ) ;
#16752=CARTESIAN_POINT ( 'NONE',  ( 6.152808582316795949, -21.53509896474924901, 4.479004561291659137 ) ) ;
#16754=CARTESIAN_POINT ( 'NONE',  ( 11.59719141768317741, -22.46490103525075810, 4.479004561291653808 ) ) ;
#16755=CARTESIAN_POINT ( 'NONE',  ( -10.09030858231679595, -21.32581373872472597, 1.729004561291657582 ) ) ;
#16757=CARTESIAN_POINT ( 'NONE',  ( 12.65457057572495181, -19.50668592589112293, 6.238308001337955488 ) ) ;
#16758=CARTESIAN_POINT ( 'NONE',  ( 13.08559773465513487, 3.760185600081874746, 5.252303440007609403 ) ) ;
#16769=CARTESIAN_POINT ( 'NONE',  ( 1.548630333695928618, -9.864917468222230923, 2.372643865078341019 ) ) ;
#16773=CARTESIAN_POINT ( 'NONE',  ( -2.203959450683124377, -9.262433282444222371, 2.410528873095051594 ) ) ;
#16774=CARTESIAN_POINT ( 'NONE',  ( -9.715308582316794173, -23.77099543870833998, 2.825813738724734847 ) ) ;
#16775=CARTESIAN_POINT ( 'NONE',  ( -2.747777887823422471, -9.906471667804277459, 1.825930796414880763 ) ) ;
#16777=CARTESIAN_POINT ( 'NONE',  ( -13.09560264576187905, 4.265433610975056133, 4.666666666666618113 ) ) ;
#16779=CARTESIAN_POINT ( 'NONE',  ( -9.434058582316794173, -23.20159541128345992, 4.773278322869455970 ) ) ;
#16780=CARTESIAN_POINT ( 'NONE',  ( 9.340308582316795949, -22.98484643305508612, 6.020995438708344416 ) ) ;
#16781=CARTESIAN_POINT ( 'NONE',  ( -11.22219141768317741, -21.02099543870834353, 3.964901035250761208 ) ) ;
#16783=CARTESIAN_POINT ( 'NONE',  ( 13.85723511636018301, 4.102873376188801657, 5.986996695041598926 ) ) ;
#16796=CARTESIAN_POINT ( 'NONE',  ( 0.9854920305337622199, -8.364917468222230923, 2.372643865078341019 ) ) ;
#16799=CARTESIAN_POINT ( 'NONE',  ( 13.86833701876684088, 3.913519447696059750, 6.741146579470268740 ) ) ;
#16801=CARTESIAN_POINT ( 'NONE',  ( 11.22219141768317741, -21.02099543870834353, 3.964901035250761208 ) ) ;
#16804=CARTESIAN_POINT ( 'NONE',  ( -6.909691417683176518, -21.63647391050456648, 4.520995438708348857 ) ) ;
#16805=CARTESIAN_POINT ( 'NONE',  ( -9.347191417683177406, -20.91377862118959285, 1.020995438708345082 ) ) ;
#16807=CARTESIAN_POINT ( 'NONE',  ( 12.62691554569741648, -19.40326494227377907, 4.703927990036796736 ) ) ;
#16808=CARTESIAN_POINT ( 'NONE',  ( -13.10557919622060652, 4.019249409169220577, 6.007898877577752650 ) ) ;
#16817=EDGE_CURVE ( 'NONE', #10698, #8256, #15634, .T. ) ;
#16822=CARTESIAN_POINT ( 'NONE',  ( -2.787023586469211001, -10.13267000451481614, 1.884023048047904103 ) ) ;
#16825=DIRECTION ( 'NONE',  ( -0.000000000000000000, -0.000000000000000000, -1.000000000000000000 ) ) ;
#16826=CARTESIAN_POINT ( 'NONE',  ( 10.84719141768317741, -20.91377862118959285, 1.020995438708345082 ) ) ;
#16827=CARTESIAN_POINT ( 'NONE',  ( -13.08094078691552831, 2.775009739235173356, 5.981149842915306714 ) ) ;
#16828=CARTESIAN_POINT ( 'NONE',  ( -5.690941417683177406, -23.80360840875937001, 5.231925497173365081 ) ) ;
#16830=FACE_OUTER_BOUND ( 'NONE', #12519, .T. ) ;
#16832=CARTESIAN_POINT ( 'NONE',  ( -13.89075858682503650, 5.045808634669852744, 6.406973581600956535 ) ) ;
#16833=CARTESIAN_POINT ( 'NONE',  ( 10.27780858231679417, -20.27099543870833642, 2.724438792969431589 ) ) ;
#16837=CARTESIAN_POINT ( 'NONE',  ( 13.70116456325478893, -3.778689555664588973, 5.825679699621801433 ) ) ;
#16844=CARTESIAN_POINT ( 'NONE',  ( 13.87470602645761986, 4.985154336109792972, 4.333333333333379223 ) ) ;
#16845=( BOUNDED_CURVE ( )  B_SPLINE_CURVE ( 2, ( #17064, #4417, #15699, #1480, #14222, #7554, #1275, #20534, #10900, #20630, #6187, #2744, #14327, #15591, #12357, #9528, #6283, #18751, #12657, #18953, #4608, #9124, #10801, #2845, #17371, #7954, #17478, #15900, #7655, #14751, #120, #11205, #12968, #8271, #3663, #17578, #1994, #3252, #17892, #6505, #14543, #17686, #6400, #14850, #11299, #3357, #19575, #4824, #8073, #3459, #8481, #1891, #13077, #9624, #14641, #16121, #19479, #429, #16010, #8175, #11407, #12867, #1687, #323, #16224, #6601, #9939, #4921, #19372, #19269, #17793, #14438, #6708, #5132, #11511, #5027, #5229, #215, #9736, #12767, #3559, #9837, #16318, #8379, #1788, #6808, #13176, #11607, #17992, #10047, #19170, #16421, #2098, #14947, #12129 ),
 .UNSPECIFIED., .F., .F. ) 
 B_SPLINE_CURVE_WITH_KNOTS ( ( 3, 2, 2, 2, 2, 2, 2, 2, 2, 2, 2, 2, 2, 2, 2, 2, 2, 2, 2, 2, 2, 2, 2, 2, 2, 2, 2, 2, 2, 2, 2, 2, 2, 2, 2, 2, 2, 2, 2, 2, 2, 2, 2, 2, 2, 2, 2, 3 ),
 ( 0.000000000000000000, 0.02083333333333333218, 0.04166666666666666435, 0.06250000000000000000, 0.08333333333333332871, 0.1041666666666666713, 0.1250000000000000000, 0.1458333333333333426, 0.1666666666666666574, 0.1875000000000000000, 0.2083333333333333426, 0.2291666666666666574, 0.2500000000000000000, 0.2708333333333333148, 0.2916666666666666852, 0.3124999999999999445, 0.3333333333333333148, 0.3541666666666666852, 0.3750000000000000000, 0.3958333333333333148, 0.4166666666666666852, 0.4375000000000000555, 0.4583333333333333148, 0.4791666666666666852, 0.5000000000000000000, 0.5208333333333333703, 0.5416666666666666297, 0.5625000000000000000, 0.5833333333333333703, 0.6041666666666666297, 0.6249999999999998890, 0.6458333333333333703, 0.6666666666666666297, 0.6875000000000000000, 0.7083333333333333703, 0.7291666666666666297, 0.7500000000000000000, 0.7708333333333333703, 0.7916666666666666297, 0.8125000000000000000, 0.8333333333333333703, 0.8541666666666666297, 0.8750000000000001110, 0.8958333333333333703, 0.9166666666666666297, 0.9375000000000000000, 0.9583333333333333703, 0.9650437087885355147 ),
 .UNSPECIFIED. ) 
 CURVE ( )  GEOMETRIC_REPRESENTATION_ITEM ( )  RATIONAL_B_SPLINE_CURVE ( ( 1.000000000000000000, 0.9238795325112867385, 1.000000000000000000, 0.9238795325112867385, 1.000000000000000000, 0.9238795325112867385, 1.000000000000000000, 0.9238795325112867385, 1.000000000000000000, 0.9238795325112867385, 1.000000000000000000, 0.9238795325112867385, 1.000000000000000000, 0.9238795325112867385, 1.000000000000000000, 0.9238795325112867385, 1.000000000000000000, 0.9238795325112867385, 1.000000000000000000, 0.9238795325112867385, 1.000000000000000000, 0.9238795325112867385, 1.000000000000000000, 0.9238795325112867385, 1.000000000000000000, 0.9238795325112867385, 1.000000000000000000, 0.9238795325112867385, 1.000000000000000000, 0.9238795325112867385, 1.000000000000000000, 0.9238795325112867385, 1.000000000000000000, 0.9238795325112867385, 1.000000000000000000, 0.9238795325112867385, 1.000000000000000000, 0.9238795325112867385, 1.000000000000000000, 0.9238795325112867385, 1.000000000000000000, 0.9238795325112867385, 1.000000000000000000, 0.9238795325112867385, 1.000000000000000000, 0.9238795325112867385, 1.000000000000000000, 0.9238795325112867385, 1.000000000000000000, 0.9238795325112867385, 1.000000000000000000, 0.9238795325112867385, 1.000000000000000000, 0.9238795325112867385, 1.000000000000000000, 0.9238795325112867385, 1.000000000000000000, 0.9238795325112867385, 1.000000000000000000, 0.9238795325112867385, 1.000000000000000000, 0.9238795325112867385, 1.000000000000000000, 0.9238795325112867385, 1.000000000000000000, 0.9238795325112867385, 1.000000000000000000, 0.9238795325112867385, 1.000000000000000000, 0.9238795325112867385, 1.000000000000000000, 0.9238795325112867385, 1.000000000000000000, 0.9238795325112867385, 1.000000000000000000, 0.9238795325112867385, 1.000000000000000000, 0.9238795325112867385, 1.000000000000000000, 0.9238795325112867385, 1.000000000000000000, 0.9238795325112867385, 1.000000000000000000, 0.9238795325112867385, 1.000000000000000000, 0.9238795325112867385, 1.000000000000000000, 0.9238795325112867385, 1.000000000000000000, 0.9238795325112867385, 1.000000000000000000, 0.9238795325112867385, 1.000000000000000000, 0.9754817479996107377, 0.9667580569362973497 ) ) 
 REPRESENTATION_ITEM ( '' )  );
#16847=CARTESIAN_POINT ( 'NONE',  ( 1.960495238260606010, -8.383787449798761671, 1.627490053312942164 ) ) ;
#16849=CARTESIAN_POINT ( 'NONE',  ( -12.66835678905406049, -17.31048215276408797, 4.799178440007564994 ) ) ;
#16850=CARTESIAN_POINT ( 'NONE',  ( 10.74655858231679417, -21.94931252712234482, 5.250000000000000888 ) ) ;
#16851=CARTESIAN_POINT ( 'NONE',  ( -13.77324158252158171, -0.8888000826463379189, 6.637859435864801760 ) ) ;
#16854=CARTESIAN_POINT ( 'NONE',  ( 10.74655858231679417, -21.94931252712234482, 5.250000000000000888 ) ) ;
#16855=CARTESIAN_POINT ( 'NONE',  ( 5.784691417683179182, -23.77099543870834353, 4.174186261275252718 ) ) ;
#16856=CARTESIAN_POINT ( 'NONE',  ( -9.527808582316792396, -23.72900456129165647, 4.275561207030568411 ) ) ;
#16858=CARTESIAN_POINT ( 'NONE',  ( 12.66503773474750894, -18.97809439524806052, 6.263381662489337920 ) ) ;
#16859=CARTESIAN_POINT ( 'NONE',  ( 13.08739618700683849, 3.851007443844064237, 5.254256565007597857 ) ) ;
#16864=CARTESIAN_POINT ( 'NONE',  ( -12.64691428603184242, -19.14332855539073464, 5.509795676248469221 ) ) ;
#16866=CARTESIAN_POINT ( 'NONE',  ( -13.39662663169496781, -19.15785509940297615, 5.494950532956567102 ) ) ;
#16868=CARTESIAN_POINT ( 'NONE',  ( 2.731427961995660958, -10.89409100229510052, 2.829571171190552015 ) ) ;
#16873=CARTESIAN_POINT ( 'NONE',  ( -9.527808582316795949, -24.47900456129166358, 4.586221378810390270 ) ) ;
#16874=CARTESIAN_POINT ( 'NONE',  ( -1.960495238260606010, -8.383787449798761671, 1.627490053312942164 ) ) ;
#16876=CARTESIAN_POINT ( 'NONE',  ( -13.81612658856640863, 2.776892722604777930, 5.216624963382545666 ) ) ;
#16879=CARTESIAN_POINT ( 'NONE',  ( 4.934058582316795061, -23.73192549717337130, 5.303608408759367343 ) ) ;
#16880=CARTESIAN_POINT ( 'NONE',  ( -9.534691417683177406, -20.97900456129164581, 3.136473910504570917 ) ) ;
#16882=CARTESIAN_POINT ( 'NONE',  ( 13.37499999999998224, -20.24999999999991829, 4.333333333333343695 ) ) ;
#16889=CARTESIAN_POINT ( 'NONE',  ( -13.58606361274418184, -9.591287556442823714, 5.700679699621803209 ) ) ;
#16895=CARTESIAN_POINT ( 'NONE',  ( 1.513434189748285918, -8.364917468222230923, 2.372643865078341019 ) ) ;
#16897=CARTESIAN_POINT ( 'NONE',  ( 13.89075858682503650, 5.045808634669852744, 6.406973581600956535 ) ) ;
#16901=CARTESIAN_POINT ( 'NONE',  ( 10.37844141768317741, -22.99999999999999645, 3.449312527122335048 ) ) ;
#16902=CARTESIAN_POINT ( 'NONE',  ( -12.63819864697926754, -19.58346832754827105, 5.450273968536036406 ) ) ;
#16903=CARTESIAN_POINT ( 'NONE',  ( -6.440941417683175629, -21.25705176302044208, 2.828734674606458555 ) ) ;
#16905=CARTESIAN_POINT ( 'NONE',  ( -9.722191417683177406, -19.52099543870834353, 4.586221378810406257 ) ) ;
#16907=CARTESIAN_POINT ( 'NONE',  ( 12.63298722613685676, -19.09664508008815531, 4.760766981674283471 ) ) ;
#16908=CARTESIAN_POINT ( 'NONE',  ( -12.65051119073526564, -18.96168486786632457, 5.513701926248478102 ) ) ;
#16913=CARTESIAN_POINT ( 'NONE',  ( 1.872293763630120678, -10.04602735435188698, 2.419156501869924369 ) ) ;
#16919=CARTESIAN_POINT ( 'NONE',  ( -1.733187991654075777, -9.867296153774269385, 1.623254759047128237 ) ) ;
#16923=CARTESIAN_POINT ( 'NONE',  ( 11.97219141768317918, -24.47900456129165292, 2.413778621189595963 ) ) ;
#16924=CARTESIAN_POINT ( 'NONE',  ( -12.63249216759192350, -19.87164553660301536, 5.297612231341934041 ) ) ;
#16925=CARTESIAN_POINT ( 'NONE',  ( -8.878441417683177406, -24.50000000000000000, 3.449312527122335048 ) ) ;
#16929=CARTESIAN_POINT ( 'NONE',  ( 11.77780858231679417, -20.27099543870833642, 2.724438792969431589 ) ) ;
#16931=CARTESIAN_POINT ( 'NONE',  ( -13.87372783958217681, 4.185755898898970706, 6.732634959205082481 ) ) ;
#16932=CARTESIAN_POINT ( 'NONE',  ( 6.246558582316795949, -21.94931252712234127, 4.499999999999999112 ) ) ;
#16935=ORIENTED_EDGE ( 'NONE', *, *, #20543, .F. ) ;
#16936=CARTESIAN_POINT ( 'NONE',  ( 13.40787921250184311, -19.33959976865745389, 6.241060671539915283 ) ) ;
#16941=CARTESIAN_POINT ( 'NONE',  ( -12.43405858231679417, -23.20159541128345992, 4.773278322869455970 ) ) ;
#16944=CARTESIAN_POINT ( 'NONE',  ( 2.762374231067749708, -9.968169115173667549, 1.841775933429679268 ) ) ;
#16946=CARTESIAN_POINT ( 'NONE',  ( -13.37500003877585186, -19.49999804181952712, 4.520055687292853008 ) ) ;
#16947=CARTESIAN_POINT ( 'NONE',  ( 11.77780858231679417, -20.27099543870833642, 2.724438792969431589 ) ) ;
#16948=CARTESIAN_POINT ( 'NONE',  ( -13.40995420747273670, -19.23481252262645924, 6.243328185864100988 ) ) ;
#16952=CARTESIAN_POINT ( 'NONE',  ( 6.246558582316795949, -21.94931252712234127, 4.499999999999999112 ) ) ;
#16953=CARTESIAN_POINT ( 'NONE',  ( 5.222191417683178294, -20.27099543870833998, 4.275561207030583510 ) ) ;
#16954=CARTESIAN_POINT ( 'NONE',  ( -12.80905858231679417, -23.27327832286945153, 2.298404588716537411 ) ) ;
#16955=ORIENTED_EDGE ( 'NONE', *, *, #492, .F. ) ;
#16956=CARTESIAN_POINT ( 'NONE',  ( 13.09560264576187905, 4.265433610975056133, 4.333333333333380999 ) ) ;
#16961=( BOUNDED_SURFACE ( )  B_SPLINE_SURFACE ( 3, 3, ( 
 ( #6022, #10936, #17415, #15839, #12395, #14259, #2882, #6326, #9564, #12498, #2987, #5145, #9259, #15937, #4757, #18894, #4553, #9364, #1617, #15738, #14164, #12699, #19102, #751, #5242, #7233, #539, #19900, #6916, #15175, #11928, #13190, #19586, #5664, #12035, #18429, #19801, #18322, #11619, #5350 ),
 ( #14765, #16435, #441, #6821, #13397, #15070, #19999, #2308, #18007, #5557, #8807, #10369, #3677, #19687, #10164, #14960, #5457, #9950, #10064, #13287, #2111, #3986, #3882, #16629, #16333, #11828, #8494, #14863, #16745, #8698, #11728, #16533, #18121, #2416, #2008, #3784, #7137, #2209, #8591, #641 ),
 ( #7029, #18219, #8395, #10262, #13501, #851, #13597, #17253, #15483, #4093, #2934, #6178, #18739, #7643, #18633, #15381, #17160, #15271, #4296, #9313, #4507, #18532, #1165, #5871, #1372, #16847, #8906, #12240, #10478, #6082, #10891, #7753, #15689, #20108, #14118, #20211, #20421, #13701, #20525, #14013 ),
 ( #10681, #2514, #5971, #17055, #951, #12546, #13807, #7339, #5770, #10577, #12142, #4195, #7545, #9211, #16944, #2836, #2618, #12451, #9010, #1066, #7445, #2734, #9114, #13908, #20308, #12345, #4407, #10791, #15583, #18845, #1267, #8061, #18943, #17567, #4706, #6272, #3346, #108, #15792, #20719 ),
 ( #14425, #14531, #14212, #15890, #12645, #6494, #6388, #1778, #1568, #19051, #19359, #4598, #12755, #12855, #19257, #8165, #11192, #10990, #206, #17360, #4909, #9724, #19159, #7944, #11288, #7850, #4813, #12956, #6590, #11097, #9613, #3241, #5015, #1470, #20621, #15996, #3045, #9422, #17468, #3145 ),
 ( #9516, #14314, #1674, #17672, #16109, #7609, #10861, #10754, #17125, #15343, #18811, #2805, #16913, #9385, #5937, #13776, #12417, #20180, #13978, #18914, #1136, #12308, #15759, #7415, #4572, #6148, #10645, #12208, #1442, #12517, #9179, #7820, #17018, #15554, #7716, #18599, #14182, #7514, #10957, #13877 ),
 ( #19018, #20493, #1340, #20278, #4672, #2696, #3008, #14086, #4370, #5840, #17325, #20382, #6047, #20590, #6242, #18705, #12614, #2586, #4478, #8970, #17225, #1026, #4262, #9083, #1234, #15452, #2903, #9279, #15653, #11315, #6614, #17487, #13262, #14232, #20640, #7002, #13369, #19772, #133, #19659 ) ),
 .UNSPECIFIED., .T., .F., .T. ) 
 B_SPLINE_SURFACE_WITH_KNOTS ( ( 4, 3, 4 ),
 ( 4, 2, 2, 2, 2, 2, 2, 2, 2, 2, 2, 2, 2, 2, 2, 2, 2, 2, 2, 4 ),
 ( 0.000000000000000000, 0.5000000000000000000, 1.000000000000000000 ),
 ( 0.000000000000000000, 0.3100443560520446118, 0.4650665340780669177, 0.5425776230910780429, 0.5813331675975836887, 0.6007109398508364562, 0.6200887121040892236, 0.6309950902025724950, 0.6419014683010558775, 0.6637142244980225314, 0.7073397368919559502, 0.7509652492858893691, 0.7727780054828560230, 0.7836843835813394055, 0.7945907616798226769, 0.8074288390748337596, 0.8202669164698448423, 0.8459430712598670077, 0.8972953808399113385, 1.000000000000000000 ),
 .UNSPECIFIED. ) 
 GEOMETRIC_REPRESENTATION_ITEM ( )  RATIONAL_B_SPLINE_SURFACE ( (
 ( 1.000000000000000000, 1.000000000000000000, 1.000000000000000000, 1.000000000000000000, 1.000000000000000000, 1.000000000000000000, 1.000000000000000000, 1.000000000000000000, 1.000000000000000000, 1.000000000000000000, 1.000000000000000000, 1.000000000000000000, 1.000000000000000000, 1.000000000000000000, 1.000000000000000000, 1.000000000000000000, 1.000000000000000000, 1.000000000000000000, 1.000000000000000000, 1.000000000000000000, 1.000000000000000000, 1.000000000000000000, 1.000000000000000000, 1.000000000000000000, 1.000000000000000000, 1.000000000000000000, 1.000000000000000000, 1.000000000000000000, 1.000000000000000000, 1.000000000000000000, 1.000000000000000000, 1.000000000000000000, 1.000000000000000000, 1.000000000000000000, 1.000000000000000000, 1.000000000000000000, 1.000000000000000000, 1.000000000000000000, 1.000000000000000000, 1.000000000000000000),
 ( 0.3333333333333333703, 0.3333333333333333703, 0.3333333333333333703, 0.3333333333333333703, 0.3333333333333333703, 0.3333333333333333703, 0.3333333333333333703, 0.3333333333333333703, 0.3333333333333333703, 0.3333333333333333703, 0.3333333333333333703, 0.3333333333333333703, 0.3333333333333333703, 0.3333333333333333703, 0.3333333333333333703, 0.3333333333333333703, 0.3333333333333333703, 0.3333333333333333703, 0.3333333333333333703, 0.3333333333333333703, 0.3333333333333333703, 0.3333333333333333703, 0.3333333333333333703, 0.3333333333333333703, 0.3333333333333333703, 0.3333333333333333703, 0.3333333333333333703, 0.3333333333333333703, 0.3333333333333333703, 0.3333333333333333703, 0.3333333333333333703, 0.3333333333333333703, 0.3333333333333333703, 0.3333333333333333703, 0.3333333333333333703, 0.3333333333333333703, 0.3333333333333333703, 0.3333333333333333703, 0.3333333333333333703, 0.3333333333333333703),
 ( 0.3333333333333333703, 0.3333333333333333703, 0.3333333333333333703, 0.3333333333333333703, 0.3333333333333333703, 0.3333333333333333703, 0.3333333333333333703, 0.3333333333333333703, 0.3333333333333333703, 0.3333333333333333703, 0.3333333333333333703, 0.3333333333333333703, 0.3333333333333333703, 0.3333333333333333703, 0.3333333333333333703, 0.3333333333333333703, 0.3333333333333333703, 0.3333333333333333703, 0.3333333333333333703, 0.3333333333333333703, 0.3333333333333333703, 0.3333333333333333703, 0.3333333333333333703, 0.3333333333333333703, 0.3333333333333333703, 0.3333333333333333703, 0.3333333333333333703, 0.3333333333333333703, 0.3333333333333333703, 0.3333333333333333703, 0.3333333333333333703, 0.3333333333333333703, 0.3333333333333333703, 0.3333333333333333703, 0.3333333333333333703, 0.3333333333333333703, 0.3333333333333333703, 0.3333333333333333703, 0.3333333333333333703, 0.3333333333333333703),
 ( 1.000000000000000000, 1.000000000000000000, 1.000000000000000000, 1.000000000000000000, 1.000000000000000000, 1.000000000000000000, 1.000000000000000000, 1.000000000000000000, 1.000000000000000000, 1.000000000000000000, 1.000000000000000000, 1.000000000000000000, 1.000000000000000000, 1.000000000000000000, 1.000000000000000000, 1.000000000000000000, 1.000000000000000000, 1.000000000000000000, 1.000000000000000000, 1.000000000000000000, 1.000000000000000000, 1.000000000000000000, 1.000000000000000000, 1.000000000000000000, 1.000000000000000000, 1.000000000000000000, 1.000000000000000000, 1.000000000000000000, 1.000000000000000000, 1.000000000000000000, 1.000000000000000000, 1.000000000000000000, 1.000000000000000000, 1.000000000000000000, 1.000000000000000000, 1.000000000000000000, 1.000000000000000000, 1.000000000000000000, 1.000000000000000000, 1.000000000000000000),
 ( 0.3333333333333333703, 0.3333333333333333703, 0.3333333333333333703, 0.3333333333333333703, 0.3333333333333333703, 0.3333333333333333703, 0.3333333333333333703, 0.3333333333333333703, 0.3333333333333333703, 0.3333333333333333703, 0.3333333333333333703, 0.3333333333333333703, 0.3333333333333333703, 0.3333333333333333703, 0.3333333333333333703, 0.3333333333333333703, 0.3333333333333333703, 0.3333333333333333703, 0.3333333333333333703, 0.3333333333333333703, 0.3333333333333333703, 0.3333333333333333703, 0.3333333333333333703, 0.3333333333333333703, 0.3333333333333333703, 0.3333333333333333703, 0.3333333333333333703, 0.3333333333333333703, 0.3333333333333333703, 0.3333333333333333703, 0.3333333333333333703, 0.3333333333333333703, 0.3333333333333333703, 0.3333333333333333703, 0.3333333333333333703, 0.3333333333333333703, 0.3333333333333333703, 0.3333333333333333703, 0.3333333333333333703, 0.3333333333333333703),
 ( 0.3333333333333333703, 0.3333333333333333703, 0.3333333333333333703, 0.3333333333333333703, 0.3333333333333333703, 0.3333333333333333703, 0.3333333333333333703, 0.3333333333333333703, 0.3333333333333333703, 0.3333333333333333703, 0.3333333333333333703, 0.3333333333333333703, 0.3333333333333333703, 0.3333333333333333703, 0.3333333333333333703, 0.3333333333333333703, 0.3333333333333333703, 0.3333333333333333703, 0.3333333333333333703, 0.3333333333333333703, 0.3333333333333333703, 0.3333333333333333703, 0.3333333333333333703, 0.3333333333333333703, 0.3333333333333333703, 0.3333333333333333703, 0.3333333333333333703, 0.3333333333333333703, 0.3333333333333333703, 0.3333333333333333703, 0.3333333333333333703, 0.3333333333333333703, 0.3333333333333333703, 0.3333333333333333703, 0.3333333333333333703, 0.3333333333333333703, 0.3333333333333333703, 0.3333333333333333703, 0.3333333333333333703, 0.3333333333333333703),
 ( 1.000000000000000000, 1.000000000000000000, 1.000000000000000000, 1.000000000000000000, 1.000000000000000000, 1.000000000000000000, 1.000000000000000000, 1.000000000000000000, 1.000000000000000000, 1.000000000000000000, 1.000000000000000000, 1.000000000000000000, 1.000000000000000000, 1.000000000000000000, 1.000000000000000000, 1.000000000000000000, 1.000000000000000000, 1.000000000000000000, 1.000000000000000000, 1.000000000000000000, 1.000000000000000000, 1.000000000000000000, 1.000000000000000000, 1.000000000000000000, 1.000000000000000000, 1.000000000000000000, 1.000000000000000000, 1.000000000000000000, 1.000000000000000000, 1.000000000000000000, 1.000000000000000000, 1.000000000000000000, 1.000000000000000000, 1.000000000000000000, 1.000000000000000000, 1.000000000000000000, 1.000000000000000000, 1.000000000000000000, 1.000000000000000000, 1.000000000000000000) ) ) 
 REPRESENTATION_ITEM ( '' )  SURFACE ( )  );
#16965=CARTESIAN_POINT ( 'NONE',  ( -12.64571531779736979, -19.20387645123237164, 5.508493592915143289 ) ) ;
#16966=CARTESIAN_POINT ( 'NONE',  ( -2.623717082130370137, -10.12934627674766830, 2.633169448359191644 ) ) ;
#16967=CARTESIAN_POINT ( 'NONE',  ( -13.38921792038197900, -19.53199502070850357, 5.456033026503027017 ) ) ;
#16969=CARTESIAN_POINT ( 'NONE',  ( 0.000000000000000000, -9.114917468222230923, 1.997643865078340797 ) ) ;
#16975=CARTESIAN_POINT ( 'NONE',  ( -12.24655858231679595, -21.94931252712234127, 6.000000000000001776 ) ) ;
#16976=CARTESIAN_POINT ( 'NONE',  ( -1.731569788986178304, -8.364930642962441709, 1.622647248614820015 ) ) ;
#16978=CARTESIAN_POINT ( 'NONE',  ( -13.84256985046264710, 4.112277448363203192, 5.213861325540929847 ) ) ;
#16980=CARTESIAN_POINT ( 'NONE',  ( 9.628441417683177406, -19.49999999999998934, 3.550687472877664952 ) ) ;
#16981=CARTESIAN_POINT ( 'NONE',  ( -12.62844141768317741, -20.99999999999999645, 3.550687472877664952 ) ) ;
#16983=CARTESIAN_POINT ( 'NONE',  ( 13.83065313257865370, 2.760483195222930952, 5.966304699623404595 ) ) ;
#16991=CARTESIAN_POINT ( 'NONE',  ( -13.47096266223369376, -15.40388555723029462, 5.575679699623145247 ) ) ;
#16993=CARTESIAN_POINT ( 'NONE',  ( 1.407845757905374695, -9.114917468222230923, 2.372643865078341019 ) ) ;
#17001=CARTESIAN_POINT ( 'NONE',  ( 0.5631383031621635116, -9.114917468222230923, 2.372643865078341019 ) ) ;
#17007=CARTESIAN_POINT ( 'NONE',  ( 5.128441417683177406, -20.24999999999999289, 3.550687472877664952 ) ) ;
#17008=CARTESIAN_POINT ( 'NONE',  ( -12.62500016093973620, -20.24999187254239175, 4.532396751752561848 ) ) ;
#17009=CARTESIAN_POINT ( 'NONE',  ( -12.62155858231679417, -22.99999999999999645, 3.550687472877652073 ) ) ;
#17010=CARTESIAN_POINT ( 'NONE',  ( -8.128441417683177406, -19.49999999999998934, 3.550687472877664952 ) ) ;
#17012=CARTESIAN_POINT ( 'NONE',  ( 13.12529397354238192, 5.014845663890295846, 4.166666666666765551 ) ) ;
#17013=CARTESIAN_POINT ( 'NONE',  ( -13.12529397353891270, 5.014845663890295846, 3.333333333333220239 ) ) ;
#17018=CARTESIAN_POINT ( 'NONE',  ( 1.513434189748285918, -9.864917468222230923, 2.372643865078341019 ) ) ;
#17025=CARTESIAN_POINT ( 'NONE',  ( -1.776440835594205847, -9.874406767442327038, 1.625080906685880233 ) ) ;
#17031=CARTESIAN_POINT ( 'NONE',  ( 12.15969141768317918, -22.98484643305507191, 0.9790045612916508100 ) ) ;
#17032=CARTESIAN_POINT ( 'NONE',  ( -13.00900269284621302, -0.8578640112522492034, 5.903024842915844062 ) ) ;
#17033=CARTESIAN_POINT ( 'NONE',  ( -9.065941417683177406, -23.20159541128344927, 2.226721677130534705 ) ) ;
#17038=CARTESIAN_POINT ( 'NONE',  ( -13.37499999999998224, -20.99999999999998934, 4.166666666666637653 ) ) ;
#17040=CARTESIAN_POINT ( 'NONE',  ( 9.902808582316794173, -22.77556120703056308, 1.770995438708339975 ) ) ;
#17044=CARTESIAN_POINT ( 'NONE',  ( 13.84517967659089521, 2.744073667841084418, 6.715984435864265301 ) ) ;
#17046=( LENGTH_UNIT ( ) NAMED_UNIT ( * ) SI_UNIT ( .MILLI., .METRE. ) );
#17050=CARTESIAN_POINT ( 'NONE',  ( -8.309058582316792396, -23.27327832286945153, 2.298404588716537411 ) ) ;
#17055=CARTESIAN_POINT ( 'NONE',  ( 3.059891148793807414, -12.07002330923453570, 2.381574079220715401 ) ) ;
#17058=CARTESIAN_POINT ( 'NONE',  ( -13.09073190589589331, 4.019461247742575516, 5.257453802652931607 ) ) ;
#17059=CARTESIAN_POINT ( 'NONE',  ( 12.71530858231679240, -23.77099543870833998, 2.825813738724734847 ) ) ;
#17060=CARTESIAN_POINT ( 'NONE',  ( -13.37499999999998224, -21.00000000000006395, 4.416666666666682062 ) ) ;
#17062=CARTESIAN_POINT ( 'NONE',  ( 9.809058582316794173, -23.27327832286945153, 2.298404588716537411 ) ) ;
#17063=CARTESIAN_POINT ( 'NONE',  ( 4.378441417683176518, -23.74999999999999645, 3.449312527122335492 ) ) ;
#17064=CARTESIAN_POINT ( 'NONE',  ( -12.62672070884157804, -20.24999999999991473, 3.550922209436377042 ) ) ;
#17066=CARTESIAN_POINT ( 'NONE',  ( 13.37893135632597819, -19.30146650553847465, 4.738802066438188909 ) ) ;
#17074=CARTESIAN_POINT ( 'NONE',  ( -12.65410809543883985, -18.78004118034163739, 5.517608176248461227 ) ) ;
#17078=CARTESIAN_POINT ( 'NONE',  ( -13.70116456325478893, -3.778689555664588973, 5.825679699621801433 ) ) ;
#17085=CARTESIAN_POINT ( 'NONE',  ( -8.215308582316795949, -24.52099543870834708, 2.515153566944913432 ) ) ;
#17086=CARTESIAN_POINT ( 'NONE',  ( -1.337453470010121714, -9.114917468222230923, 1.622643865078341463 ) ) ;
#17088=CARTESIAN_POINT ( 'NONE',  ( -13.38921792038197900, -19.53199502070850357, 5.456033026503027017 ) ) ;
#17091=CARTESIAN_POINT ( 'NONE',  ( 4.746558582316795061, -21.94931252712234127, 6.000000000000001776 ) ) ;
#17092=CARTESIAN_POINT ( 'NONE',  ( -10.75344141768317741, -21.94931252712233061, 2.499999999999999112 ) ) ;
#17094=CARTESIAN_POINT ( 'NONE',  ( 13.40322194933353828, -19.57479155865495457, 6.214283636730510096 ) ) ;
#17095=CARTESIAN_POINT ( 'NONE',  ( 12.62562019941893432, -20.21867992933967173, 4.757612834768309540 ) ) ;
#17102=CARTESIAN_POINT ( 'NONE',  ( 0.2815691515810352930, -9.114917468222230923, 2.372643865078523984 ) ) ;
#17107=CARTESIAN_POINT ( 'NONE',  ( 3.521144778809589315, -10.09312707791070096, 2.066482617302010105 ) ) ;
#17109=CARTESIAN_POINT ( 'NONE',  ( 13.11740841389447709, 4.616624901677048420, 5.813473370769506765 ) ) ;
#17112=CARTESIAN_POINT ( 'NONE',  ( 13.12529397354238192, 5.014845663890295846, 4.666666666666619889 ) ) ;
#17113=CARTESIAN_POINT ( 'NONE',  ( 7.753441417683177406, -21.94931252712233061, 2.499999999999999112 ) ) ;
#17114=CARTESIAN_POINT ( 'NONE',  ( -12.66849571425264287, -18.05346643024382303, 5.533233176248494978 ) ) ;
#17115=CARTESIAN_POINT ( 'NONE',  ( -11.40280858231679595, -22.46490103525074034, 2.520995438708341307 ) ) ;
#17118=CARTESIAN_POINT ( 'NONE',  ( -11.50344141768317741, -22.05068747287766229, 6.000000000000001776 ) ) ;
#17120=CARTESIAN_POINT ( 'NONE',  ( 13.09300823383486900, 4.134415808666423331, 5.226944302881396887 ) ) ;
#17121=SURFACE_SIDE_STYLE ('',( #9579 ) ) ;
#17122=VERTEX_POINT ( 'NONE', #16165 ) ;
#17125=CARTESIAN_POINT ( 'NONE',  ( 1.925499516411631973, -10.42380411186744382, 2.516177120048874283 ) ) ;
#17130=CARTESIAN_POINT ( 'NONE',  ( -2.097836924194969033, -11.64739567274323129, 2.830419876579102212 ) ) ;
#17135=CARTESIAN_POINT ( 'NONE',  ( 4.753441417683176518, -21.94931252712233061, 0.9999999999999978906 ) ) ;
#17137=CARTESIAN_POINT ( 'NONE',  ( -7.284691417683176518, -23.77099543870834353, 4.174186261275252718 ) ) ;
#17140=CARTESIAN_POINT ( 'NONE',  ( 5.777808582316794173, -20.27099543870833642, 2.724438792969431589 ) ) ;
#17142=CARTESIAN_POINT ( 'NONE',  ( -13.38795836133016870, -20.34560275282643005, 5.879540349057044146 ) ) ;
#17143=ORIENTED_EDGE ( 'NONE', *, *, #11822, .T. ) ;
#17146=CARTESIAN_POINT ( 'NONE',  ( 5.121558582316795061, -22.99999999999999645, 3.550687472877652073 ) ) ;
#17150=CARTESIAN_POINT ( 'NONE',  ( 13.41475008041063433, -18.99262093926051520, 6.248536519197435801 ) ) ;
#17156=CARTESIAN_POINT ( 'NONE',  ( -12.24655858231679240, -21.94931252712234482, 5.250000000000000888 ) ) ;
#17160=CARTESIAN_POINT ( 'NONE',  ( 3.436477319925839602, -9.631595465688135960, 1.947952079262935676 ) ) ;
#17162=CARTESIAN_POINT ( 'NONE',  ( -13.09173631808601002, 4.070184063342107805, 5.250510817581989009 ) ) ;
#17164=CARTESIAN_POINT ( 'NONE',  ( -13.37499999999998224, -20.99999999999998934, 4.291666666666699825 ) ) ;
#17166=CARTESIAN_POINT ( 'NONE',  ( 5.402808582316795949, -22.46490103525074034, 2.520995438708341307 ) ) ;
#17169=CARTESIAN_POINT ( 'NONE',  ( 9.440941417683177406, -21.25705176302044208, 2.828734674606458555 ) ) ;
#17170=CARTESIAN_POINT ( 'NONE',  ( -5.496558582316794173, -22.05068747287764452, 1.749999999999998446 ) ) ;
#17172=CARTESIAN_POINT ( 'NONE',  ( 13.09553549038190567, 4.262042264285192950, 5.042530537310905281 ) ) ;
#17173=CARTESIAN_POINT ( 'NONE',  ( -1.852280067228949445, -9.126254559850970338, 1.625555456689752321 ) ) ;
#17177=CARTESIAN_POINT ( 'NONE',  ( -12.62499999999998224, -20.24999999999998934, 4.291666666666698937 ) ) ;
#17179=CARTESIAN_POINT ( 'NONE',  ( -13.37883250981221472, -20.05645825448334563, 5.102688967256983510 ) ) ;
#17185=CARTESIAN_POINT ( 'NONE',  ( -12.80905858231679417, -23.80360840875935935, 1.768074502826626260 ) ) ;
#17186=CARTESIAN_POINT ( 'NONE',  ( -2.506848361495492394, -9.459347215042898327, 1.711100304737409150 ) ) ;
#17188=CARTESIAN_POINT ( 'NONE',  ( -13.39170256340046095, -19.40652054827866380, 5.481861153867630065 ) ) ;
#17191=CARTESIAN_POINT ( 'NONE',  ( 10.28469141768317741, -24.52099543870834708, 4.484846433055073689 ) ) ;
#17192=CARTESIAN_POINT ( 'NONE',  ( -6.347191417683176518, -21.53509896474923835, 2.520995438708346192 ) ) ;
#17195=CARTESIAN_POINT ( 'NONE',  ( 13.37499999998404299, -20.99999999996810729, 2.793053905886972998 ) ) ;
#17201=CARTESIAN_POINT ( 'NONE',  ( -13.85528666703740619, 4.004476685417483139, 5.993048563355776182 ) ) ;
#17205=FACE_OUTER_BOUND ( 'NONE', #1077, .T. ) ;
#17207=CARTESIAN_POINT ( 'NONE',  ( 1.731569788986178304, -8.364930642962441709, 1.622647248614820015 ) ) ;
#17209=CARTESIAN_POINT ( 'NONE',  ( 13.12424783836753228, 4.962015837561366993, 5.328858059679200565 ) ) ;
#17214=CARTESIAN_POINT ( 'NONE',  ( 8.597191417683177406, -22.46490103525075810, 4.479004561291653808 ) ) ;
#17215=CARTESIAN_POINT ( 'NONE',  ( -13.10012427866737639, 3.743776072700027324, 6.001983176248468332 ) ) ;
#17216=CARTESIAN_POINT ( 'NONE',  ( -11.12155858231679595, -22.99999999999999645, 3.550687472877652073 ) ) ;
#17217=CARTESIAN_POINT ( 'NONE',  ( -12.15969141768317741, -22.67418626127524917, 1.729004561291651809 ) ) ;
#17220=CARTESIAN_POINT ( 'NONE',  ( 13.37559048950600626, -19.47018027994350220, 4.620717101209816491 ) ) ;
#17225=CARTESIAN_POINT ( 'NONE',  ( 2.367358971471363649, -9.400572650371021410, 2.446005822389718087 ) ) ;
#17226=APPLICATION_CONTEXT ( 'automotive_design' ) ;
#17231=CARTESIAN_POINT ( 'NONE',  ( -1.939860967060266672, -10.52577007527361808, 2.542364016426418516 ) ) ;
#17235=CARTESIAN_POINT ( 'NONE',  ( 7.659691417683177406, -22.98484643305507191, 0.9790045612916508100 ) ) ;
#17237=CARTESIAN_POINT ( 'NONE',  ( -9.534691417683177406, -20.22900456129164581, 2.825813738724747726 ) ) ;
#17239=CARTESIAN_POINT ( 'NONE',  ( 4.717959273841178636, -21.72818306014730183, 5.243595146365860771 ) ) ;
#17241=CARTESIAN_POINT ( 'NONE',  ( -12.65986935584910000, -19.23909752961862907, 6.257782094979345899 ) ) ;
#17242=CARTESIAN_POINT ( 'NONE',  ( 8.684058582316794173, -20.79840458871652942, 2.226721677130544030 ) ) ;
#17245=CARTESIAN_POINT ( 'NONE',  ( 13.84997554952896515, 2.986265251207539606, 6.721192769197450012 ) ) ;
#17250=CARTESIAN_POINT ( 'NONE',  ( -11.87155858231679417, -20.24999999999999289, 3.449312527122348371 ) ) ;
#17253=CARTESIAN_POINT ( 'NONE',  ( 3.564229130755586006, -10.39902496812945465, 2.145043306434553987 ) ) ;
#17257=CARTESIAN_POINT ( 'NONE',  ( -13.37499999999998401, -19.49999999999998934, 2.439580858552613751 ) ) ;
#17258=CARTESIAN_POINT ( 'NONE',  ( 7.652808582316795061, -21.22443879296942626, 5.229004561291659137 ) ) ;
#17259=CARTESIAN_POINT ( 'NONE',  ( -13.90439771357353038, 5.734584535470497180, 4.942866369314573127 ) ) ;
#17260=CARTESIAN_POINT ( 'NONE',  ( 4.315753587183824180, -21.65797192216094302, 4.831781436261117335 ) ) ;
#17261=CARTESIAN_POINT ( 'NONE',  ( 8.777808582316792396, -20.27099543870833642, 2.724438792969431589 ) ) ;
#17262=CARTESIAN_POINT ( 'NONE',  ( 6.159691417683175629, -22.36352608949543352, 2.479004561291652031 ) ) ;
#17263=CARTESIAN_POINT ( 'NONE',  ( -5.027808582316793284, -23.72900456129165647, 4.275561207030568411 ) ) ;
#17265=CARTESIAN_POINT ( 'NONE',  ( 13.37680511754115287, -19.40884156416817774, 4.692171866446762429 ) ) ;
#17271=CARTESIAN_POINT ( 'NONE',  ( -12.62499999999999289, -20.24999999999899103, 3.700614806296627979 ) ) ;
#17272=CARTESIAN_POINT ( 'NONE',  ( -3.343476823822036259, -9.987837386737346890, 2.789442121235767402 ) ) ;
#17273=CARTESIAN_POINT ( 'NONE',  ( -13.77789853026076550, 0.09637577819625635367, 5.909013032956687006 ) ) ;
#17279=CARTESIAN_POINT ( 'NONE',  ( 12.62499999999998224, -20.24999999999991829, 4.333333333333343695 ) ) ;
#17280=CARTESIAN_POINT ( 'NONE',  ( -10.74655858231679595, -21.94931252712234127, 6.000000000000001776 ) ) ;
#17281=CARTESIAN_POINT ( 'NONE',  ( -2.057814715640970515, -10.20705538578787852, 1.710511717200805304 ) ) ;
#17285=CARTESIAN_POINT ( 'NONE',  ( -13.84501469867711698, 4.235742283194553259, 4.166666666666765551 ) ) ;
#17288=CARTESIAN_POINT ( 'NONE',  ( 6.059058582316795949, -20.19639159124062999, 5.231925497173373074 ) ) ;
#17289=CARTESIAN_POINT ( 'NONE',  ( -12.99655858231679595, -22.05068747287764452, 2.499999999999999112 ) ) ;
#17291=CARTESIAN_POINT ( 'NONE',  ( 13.87470602645761986, 4.985154336109792972, 3.666666666666500873 ) ) ;
#17299=CARTESIAN_POINT ( 'NONE',  ( 1.824488249492779879, -9.124319963227819130, 2.375058613629473570 ) ) ;
#17306=CARTESIAN_POINT ( 'NONE',  ( 0.000000000000000000, -8.364917468222230923, 1.622643865078341241 ) ) ;
#17308=CARTESIAN_POINT ( 'NONE',  ( 13.12529397354238192, 5.014845663890295846, 4.166666666666765551 ) ) ;
#17312=CARTESIAN_POINT ( 'NONE',  ( 5.503441417683177406, -22.05068747287766229, 4.499999999999999112 ) ) ;
#17313=CARTESIAN_POINT ( 'NONE',  ( -12.74043380832193684, -14.42059267975384529, 5.611358176248560703 ) ) ;
#17314=CARTESIAN_POINT ( 'NONE',  ( -7.465308582316796837, -20.97900456129165647, 3.863526089495444626 ) ) ;
#17315=CARTESIAN_POINT ( 'NONE',  ( -10.75344141768317741, -21.94931252712233061, 1.749999999999998446 ) ) ;
#17318=CARTESIAN_POINT ( 'NONE',  ( 12.99447614883396973, -0.8414544838704021146, 5.153345106674984244 ) ) ;
#17325=CARTESIAN_POINT ( 'NONE',  ( 2.616536356806028696, -10.07836329504444706, 2.620076000170431296 ) ) ;
#17329=CARTESIAN_POINT ( 'NONE',  ( 11.40969141768317918, -21.32581373872474373, 5.270995438708348857 ) ) ;
#17334=CARTESIAN_POINT ( 'NONE',  ( -0.2815691515810352374, -9.864917468222230923, 1.622643865078524428 ) ) ;
#17339=CARTESIAN_POINT ( 'NONE',  ( 8.128441417683177406, -19.49999999999998934, 3.550687472877664952 ) ) ;
#17341=CARTESIAN_POINT ( 'NONE',  ( -7.565941417683176518, -23.20159541128344927, 2.226721677130534705 ) ) ;
#17343=CARTESIAN_POINT ( 'NONE',  ( 5.965308582316793284, -20.22900456129164937, 4.174186261275266929 ) ) ;
#17345=CARTESIAN_POINT ( 'NONE',  ( -13.90439735423812273, 5.734566389025032684, 4.666666666666618113 ) ) ;
#17349=CARTESIAN_POINT ( 'NONE',  ( 9.340308582316794173, -22.67418626127525982, 5.270995438708342640 ) ) ;
#17357=CARTESIAN_POINT ( 'NONE',  ( -8.871558582316794173, -20.24999999999999289, 3.449312527122348371 ) ) ;
#17359=CARTESIAN_POINT ( 'NONE',  ( 13.87500000000000000, 5.000000000000049738, 4.000000000000001776 ) ) ;
#17360=CARTESIAN_POINT ( 'NONE',  ( 1.991511895312070957, -10.01421418592441448, 1.660986244685804136 ) ) ;
#17363=CARTESIAN_POINT ( 'NONE',  ( -13.08559773465513487, 3.760185600081874746, 5.252303440007609403 ) ) ;
#17364=CARTESIAN_POINT ( 'NONE',  ( 5.215308582316793284, -23.77099543870833998, 2.825813738724734847 ) ) ;
#17365=CARTESIAN_POINT ( 'NONE',  ( -12.65679946139692902, -19.39412719945235253, 6.251687395662565372 ) ) ;
#17370=CARTESIAN_POINT ( 'NONE',  ( 5.034691417683177406, -20.97900456129164581, 3.136473910504570917 ) ) ;
#17371=CARTESIAN_POINT ( 'NONE',  ( -10.37844141768317741, -23.74999999999999645, 3.449312527122335492 ) ) ;
#17373=CARTESIAN_POINT ( 'NONE',  ( 13.37559048950600626, -19.47018027994350220, 4.620717101209816491 ) ) ;
#17375=CARTESIAN_POINT ( 'NONE',  ( -2.762374231067749708, -9.968169115173667549, 1.841775933429679268 ) ) ;
#17378=PRODUCT_DEFINITION_FORMATION_WITH_SPECIFIED_SOURCE ( 'ANY', '', #1665, .NOT_KNOWN. ) ;
#17383=CARTESIAN_POINT ( 'NONE',  ( -13.11514659413808737, 4.502403003978772134, 5.887634658581065494 ) ) ;
#17384=CARTESIAN_POINT ( 'NONE',  ( -2.910499702382182807, -8.879427762644468203, 2.504780387061739333 ) ) ;
#17388=CARTESIAN_POINT ( 'NONE',  ( 10.18405858231679417, -20.79840458871652942, 2.226721677130544030 ) ) ;
#17390=CARTESIAN_POINT ( 'NONE',  ( 12.62500000000001954, -20.25000000000274269, 4.083333333315724012 ) ) ;
#17391=CARTESIAN_POINT ( 'NONE',  ( -5.121558582316795061, -24.50000000000000000, 3.550687472877651629 ) ) ;
#17392=CARTESIAN_POINT ( 'NONE',  ( -1.619022621591186928, -9.864917468222230923, 1.622643865078341907 ) ) ;
#17394=CARTESIAN_POINT ( 'NONE',  ( -13.84051394328565365, 4.008454135954084840, 5.243107695145536873 ) ) ;
#17397=VECTOR ( 'NONE', #8219, 1000.000000000000114 ) ;
#17398=CARTESIAN_POINT ( 'NONE',  ( 6.440941417683175629, -20.19639159124061933, 1.768074502826635586 ) ) ;
#17399=CARTESIAN_POINT ( 'NONE',  ( -12.15280858231679950, -21.53509896474924901, 4.479004561291659137 ) ) ;
#17402=CARTESIAN_POINT ( 'NONE',  ( 13.40653076352726103, -19.40769644187082932, 6.236886054669082746 ) ) ;
#17404=CARTESIAN_POINT ( 'NONE',  ( 12.62503117662529739, -20.24842558042254836, 4.565011198945062354 ) ) ;
#17415=CARTESIAN_POINT ( 'NONE',  ( 3.047379876266447685, -13.13734219723468755, 3.405682891496055742 ) ) ;
#17419=CARTESIAN_POINT ( 'NONE',  ( 2.589709240944451096, -9.559844081062008669, 1.736909907557668165 ) ) ;
#17424=CARTESIAN_POINT ( 'NONE',  ( -1.717920576997000737, -9.114924032904250240, 2.372645551019823884 ) ) ;
#17425=CARTESIAN_POINT ( 'NONE',  ( 5.972191417683178294, -22.97900456129165292, 3.035098964749240125 ) ) ;
#17426=CARTESIAN_POINT ( 'NONE',  ( -12.66369984131459070, -18.29565801360988075, 5.528024842915327142 ) ) ;
#17427=CARTESIAN_POINT ( 'NONE',  ( -10.27780858231679595, -21.02099543870833998, 3.035098964749253003 ) ) ;
#17428=CARTESIAN_POINT ( 'NONE',  ( -5.784691417683178294, -24.52099543870834708, 4.484846433055073689 ) ) ;
#17430=CARTESIAN_POINT ( 'NONE',  ( 13.09560264576187905, 4.265433610975056133, 4.333333333333380999 ) ) ;
#17435=EDGE_CURVE ( 'NONE', #17639, #15169, #564, .T. ) ;
#17436=EDGE_LOOP ( 'NONE', ( #8630, #4183, #5842, #18874, #18559, #3919 ) ) ;
#17441=CARTESIAN_POINT ( 'NONE',  ( -1.824218240560544047, -9.921717538097572842, 2.387231257717697286 ) ) ;
#17443=CARTESIAN_POINT ( 'NONE',  ( -8.965308582316794173, -20.22900456129164937, 4.174186261275266929 ) ) ;
#17446=CARTESIAN_POINT ( 'NONE',  ( 4.284691417683177406, -24.52099543870834708, 4.484846433055073689 ) ) ;
#17448=CARTESIAN_POINT ( 'NONE',  ( -9.159691417683179182, -22.67418626127524917, 1.729004561291651809 ) ) ;
#17450=CARTESIAN_POINT ( 'NONE',  ( 8.496558582316794173, -22.05068747287764452, 1.749999999999998446 ) ) ;
#17452=CARTESIAN_POINT ( 'NONE',  ( -12.75496035233418013, -14.43700220713569138, 6.361037912489419632 ) ) ;
#17454=CARTESIAN_POINT ( 'NONE',  ( 9.059058582316794173, -20.72672167713054137, 4.701595411283463477 ) ) ;
#17465=CARTESIAN_POINT ( 'NONE',  ( -6.902808582316793284, -22.77556120703056308, 1.770995438708339975 ) ) ;
#17468=CARTESIAN_POINT ( 'NONE',  ( 0.2815691515810352374, -9.864917468222230923, 1.622643865078524428 ) ) ;
#17470=CARTESIAN_POINT ( 'NONE',  ( -13.84501469867711698, 4.235742283194553259, 4.166666666666765551 ) ) ;
#17471=CARTESIAN_POINT ( 'NONE',  ( 6.902808582316793284, -22.77556120703056308, 1.770995438708339975 ) ) ;
#17472=CARTESIAN_POINT ( 'NONE',  ( -12.66503773474750894, -18.97809439524806052, 6.263381662489337920 ) ) ;
#17474=CARTESIAN_POINT ( 'NONE',  ( -13.87499999999999467, 5.734882735235988349, 3.999999999999984901 ) ) ;
#17475=CARTESIAN_POINT ( 'NONE',  ( -10.55905858231679595, -20.19639159124062999, 5.231925497173373074 ) ) ;
#17476=CARTESIAN_POINT ( 'NONE',  ( 6.246558582316794173, -21.94931252712234482, 5.250000000000000888 ) ) ;
#17477=CARTESIAN_POINT ( 'NONE',  ( 7.097191417683176518, -22.46490103525075810, 4.479004561291653808 ) ) ;
#17478=CARTESIAN_POINT ( 'NONE',  ( -10.19094141768317563, -23.27327832286946219, 4.701595411283453707 ) ) ;
#17480=CARTESIAN_POINT ( 'NONE',  ( 13.84051394328565365, 4.008454135954084840, 5.243107695145536873 ) ) ;
#17485=CARTESIAN_POINT ( 'NONE',  ( -13.12529397354238192, 5.014845663890295846, 4.666666666666619889 ) ) ;
#17486=CARTESIAN_POINT ( 'NONE',  ( -1.337453470010121714, -9.114917468222230923, 2.372643865078341019 ) ) ;
#17487=CARTESIAN_POINT ( 'NONE',  ( 1.548630333695928396, -9.114917468222230923, 2.372643865078341019 ) ) ;
#17490=CARTESIAN_POINT ( 'NONE',  ( -12.68288333306630378, -17.32689168014509207, 5.548858176248425700 ) ) ;
#17491=CARTESIAN_POINT ( 'NONE',  ( 10.93405858231679417, -23.20159541128345992, 4.773278322869455970 ) ) ;
#17493=CARTESIAN_POINT ( 'NONE',  ( 12.67822638532683577, -18.31206754099172684, 6.277704579156187847 ) ) ;
#17494=CARTESIAN_POINT ( 'NONE',  ( -1.126276606324276619, -9.864917468222230923, 1.622643865078341907 ) ) ;
#17496=CARTESIAN_POINT ( 'NONE',  ( -13.87470602645415063, 4.985154336109792972, 3.333333333332063830 ) ) ;
#17498=CARTESIAN_POINT ( 'NONE',  ( 6.253441417683175629, -21.94931252712233061, 0.9999999999999978906 ) ) ;
#17499=CARTESIAN_POINT ( 'NONE',  ( -6.440941417683175629, -21.25705176302044208, 2.828734674606458555 ) ) ;
#17501=CARTESIAN_POINT ( 'NONE',  ( 13.37499999999998401, -20.99999999999999645, 3.666666666666654084 ) ) ;
#17502=CARTESIAN_POINT ( 'NONE',  ( 12.62499999999998224, -20.24999999999998934, 4.291666666666698937 ) ) ;
#17510=( BOUNDED_SURFACE ( )  B_SPLINE_SURFACE ( 3, 2, ( 
 ( #12543, #9311, #9005, #18840, #13905, #20305, #4191, #12447, #2615, #12342, #16941, #7750, #17156, #15378, #4504, #9417, #17250, #10987, #2728, #947, #7334, #14115, #20417, #5967, #10787, #13697, #7442, #5868, #20104, #10888, #2833, #6174, #18736, #9111, #18630, #4402, #1264, #18940, #2931, #5767, #12138, #7640, #6078, #15686, #4595, #1369, #18529, #10677, #17357, #13803, #3040, #20208, #12237, #4293, #17050, #19462, #11093, #20618, #3546, #12642, #6491, #17778, #16716, #3445, #14528, #203, #6385, #5012, #9513, #17465, #307, #12751, #8057, #19155, #4810, #15789, #1467, #11189, #17564, #8259, #14208, #3141, #12852, #17878, #11284, #1775, #6269, #3342, #3237, #8162, #9824, #9609, #19254, #6587, #15993 ),
 ( #11497, #19048, #11393, #1564, #14421, #7941, #17668, #14624, #1671, #15886, #105, #4906, #12952, #19355, #14311, #16209, #9721, #16105, #1876, #6692, #5118, #13062, #7846, #4702, #2166, #8070, #14434, #10014, #116, #6502, #17475, #5513, #1684, #12862, #10219, #15896, #19167, #14822, #19860, #13246, #3741, #7950, #5303, #19266, #10122, #5413, #4918, #497, #16494, #11295, #2264, #19644, #15025, #13457, #9, #6984, #3247, #16392, #9621, #11677, #16587, #17683, #4821, #3632, #2071, #8455, #6877, #18075, #1576, #16005, #8550, #14920, #19753, #12762, #598, #13353, #11785, #18177, #3839, #3153, #9524, #8653, #11200, #706, #7092, #17575, #14324, #6397, #18491, #15135, #2687, #13556, #2575, #810, #18696 ),
 ( #5616, #16696, #4153, #13768, #9172, #2374, #7507, #8764, #9074, #11991, #20066, #12102, #17118, #12300, #18389, #8960, #13656, #15547, #3939, #1016, #10535, #10327, #19957, #4363, #1227, #10746, #7193, #2798, #7292, #13870, #4052, #16905, #4254, #10436, #15335, #16805, #13969, #7406, #12200, #18277, #20171, #7603, #5731, #2473, #907, #5831, #18590, #10633, #17010, #8865, #15233, #15445, #1129, #20270, #5928, #20375, #11885, #19008, #17524, #6235, #14490, #8124, #9376, #20485, #17628, #14384, #14076, #3205, #12605, #4664, #9271, #9576, #7709, #17428, #15644, #12817, #1530, #6140, #15950, #6037, #1631, #16069, #7813, #12409, #18804, #19217, #4770, #20583, #15851, #4470, #12510, #10949, #10854, #8013, #7910 ),
 ( #3001, #14175, #6344, #3301, #67, #17217, #2895, #12714, #14273, #9481, #4870, #19117, #1332, #15751, #11249, #18907, #20681, #4564, #11155, #11055, #17315, #9683, #1433, #3106, #6454, #1741, #11558, #2146, #5083, #8527, #19621, #5279, #11461, #6761, #19427, #11655, #17843, #3508, #13130, #9889, #16269, #167, #8629, #1938, #8321, #13327, #19317, #1839, #17939, #2242, #16370, #6854, #11354, #8433, #14696, #13224, #14898, #377, #3607, #18049, #19527, #5388, #2048, #18154, #16566, #3408, #10097, #6653, #5180, #13024, #14802, #479, #11762, #3719, #6551, #12914, #16473, #575, #9989, #19727, #6955, #4973, #3818, #10197, #9790, #17743, #16175, #8224, #14588, #262, #18666, #10299, #19837, #2769, #11862 ),
 ( #16981, #13741, #20144, #5594, #885, #13534, #5804, #11964, #18362, #7270, #4025, #10409, #14999, #681, #19936, #16781, #7480, #13432, #16670, #12075, #17092, #10509, #989, #5489, #2550, #2449, #7378, #2658, #8842, #18466, #12175, #15209, #20244, #16880, #12274, #10719, #18256, #4228, #786, #13631, #7171, #8937, #13841, #20039, #2347, #5703, #4128, #15308, #18563, #10608, #3918, #9048, #15417, #1101, #5902, #8740, #4335, #7067, #15109, #20654, #9347, #17603, #11227, #12486, #2869, #41, #17499, #17192, #6311, #15726, #1407, #12384, #12686, #10827, #20559, #18777, #15926, #4636, #9246, #19088, #9148, #4743, #19193, #10924, #15517, #1202, #1603, #7886, #2971, #18981, #7578, #15616, #14049, #13941, #11130 ),
 ( #20343, #11029, #4444, #6007, #17289, #4846, #14152, #6210, #1299, #3179, #7680, #20458, #7789, #17399, #6427, #6115, #9553, #18878, #7982, #4539, #12580, #3081, #14355, #12791, #9455, #15827, #1504, #14245, #16040, #13102, #16246, #1716, #11327, #10074, #550, #16448, #19295, #8503, #19399, #19599, #12891, #9862, #16344, #8101, #8296, #14465, #5361, #1915, #3581, #9654, #19505, #2019, #8409, #17714, #11629, #5156, #14670, #3385, #18019, #6930, #6737, #17819, #6831, #14776, #350, #8200, #11535, #453, #4948, #11435, #144, #9764, #3690, #13297, #19698, #6530, #2122, #17914, #9962, #3486, #16150, #13200, #1814, #6628, #5252, #5058, #14566, #14874, #11739, #239, #12997, #3276, #7245, #18334, #961 ),
 ( #2426, #7039, #13607, #5675, #4103, #3997, #16954, #11938, #3893, #18131, #8915, #5880, #10486, #5781, #1076, #9020, #10382, #7455, #15080, #7350, #19913, #13712, #762, #12046, #2219, #18441, #13511, #19813, #5567, #18230, #2523, #16543, #10272, #20011, #10586, #16755, #5467, #7147, #8817, #15185, #862, #16856, #8602, #16640, #15283, #20118, #12150, #13408, #18541, #4204, #2633, #15391, #13817, #3796, #20219, #10173, #11839, #14973, #651, #2320, #8708, #18855, #4516, #15492, #3057, #13917, #2942, #1176, #19060, #7764, #20319, #9431, #12, #7860, #1579, #14025, #12250, #18642, #4718, #11002, #6093, #1383, #4308, #5982, #17170, #10693, #15803, #14129, #11107, #17263, #20434, #9221, #12461, #12555, #3156 ) ),
 .UNSPECIFIED., .T., .F., .F. ) 
 B_SPLINE_SURFACE_WITH_KNOTS ( ( 4, 3, 4 ),
 ( 3, 2, 2, 2, 2, 2, 2, 2, 2, 2, 2, 2, 2, 2, 2, 2, 2, 2, 2, 2, 2, 2, 2, 2, 2, 2, 2, 2, 2, 2, 2, 2, 2, 2, 2, 2, 2, 2, 2, 2, 2, 2, 2, 2, 2, 2, 2, 3 ),
 ( 0.000000000000000000, 0.5000000000000000000, 1.000000000000000000 ),
 ( 0.000000000000000000, 0.02083333333333333218, 0.04166666666666666435, 0.06250000000000000000, 0.08333333333333332871, 0.1041666666666666713, 0.1250000000000000000, 0.1458333333333333426, 0.1666666666666666574, 0.1875000000000000000, 0.2083333333333333426, 0.2291666666666666574, 0.2500000000000000000, 0.2708333333333333148, 0.2916666666666666852, 0.3125000000000000000, 0.3333333333333333148, 0.3541666666666666852, 0.3750000000000000000, 0.3958333333333333148, 0.4166666666666666852, 0.4375000000000000000, 0.4583333333333333148, 0.4791666666666666852, 0.5000000000000000000, 0.5208333333333333703, 0.5416666666666666297, 0.5625000000000000000, 0.5833333333333333703, 0.6041666666666666297, 0.6250000000000000000, 0.6458333333333333703, 0.6666666666666666297, 0.6875000000000000000, 0.7083333333333333703, 0.7291666666666666297, 0.7500000000000000000, 0.7708333333333333703, 0.7916666666666666297, 0.8125000000000000000, 0.8333333333333333703, 0.8541666666666666297, 0.8750000000000000000, 0.8958333333333333703, 0.9166666666666666297, 0.9375000000000000000, 0.9583333333333333703, 0.9650437087885355147 ),
 .UNSPECIFIED. ) 
 GEOMETRIC_REPRESENTATION_ITEM ( )  RATIONAL_B_SPLINE_SURFACE ( (
 ( 1.000000000000000000, 0.9238795325112867385, 1.000000000000000000, 0.9238795325112867385, 1.000000000000000000, 0.9238795325112867385, 1.000000000000000000, 0.9238795325112867385, 1.000000000000000000, 0.9238795325112867385, 1.000000000000000000, 0.9238795325112867385, 1.000000000000000000, 0.9238795325112867385, 1.000000000000000000, 0.9238795325112867385, 1.000000000000000000, 0.9238795325112867385, 1.000000000000000000, 0.9238795325112867385, 1.000000000000000000, 0.9238795325112867385, 1.000000000000000000, 0.9238795325112867385, 1.000000000000000000, 0.9238795325112867385, 1.000000000000000000, 0.9238795325112867385, 1.000000000000000000, 0.9238795325112867385, 1.000000000000000000, 0.9238795325112867385, 1.000000000000000000, 0.9238795325112867385, 1.000000000000000000, 0.9238795325112867385, 1.000000000000000000, 0.9238795325112867385, 1.000000000000000000, 0.9238795325112867385, 1.000000000000000000, 0.9238795325112867385, 1.000000000000000000, 0.9238795325112867385, 1.000000000000000000, 0.9238795325112867385, 1.000000000000000000, 0.9238795325112867385, 1.000000000000000000, 0.9238795325112867385, 1.000000000000000000, 0.9238795325112867385, 1.000000000000000000, 0.9238795325112867385, 1.000000000000000000, 0.9238795325112867385, 1.000000000000000000, 0.9238795325112867385, 1.000000000000000000, 0.9238795325112867385, 1.000000000000000000, 0.9238795325112867385, 1.000000000000000000, 0.9238795325112867385, 1.000000000000000000, 0.9238795325112867385, 1.000000000000000000, 0.9238795325112867385, 1.000000000000000000, 0.9238795325112867385, 1.000000000000000000, 0.9238795325112867385, 1.000000000000000000, 0.9238795325112867385, 1.000000000000000000, 0.9238795325112867385, 1.000000000000000000, 0.9238795325112867385, 1.000000000000000000, 0.9238795325112867385, 1.000000000000000000, 0.9238795325112867385, 1.000000000000000000, 0.9238795325112867385, 1.000000000000000000, 0.9238795325112867385, 1.000000000000000000, 0.9238795325112867385, 1.000000000000000000, 0.9238795325112867385, 1.000000000000000000, 0.9238795325112867385, 1.000000000000000000, 0.9754817479996107377, 0.9667580569362973497),
 ( 0.3333333333333333703, 0.3079598441704289313, 0.3333333333333333703, 0.3079598441704289313, 0.3333333333333333703, 0.3079598441704289313, 0.3333333333333333703, 0.3079598441704289313, 0.3333333333333333703, 0.3079598441704289313, 0.3333333333333333703, 0.3079598441704289313, 0.3333333333333333703, 0.3079598441704289313, 0.3333333333333333703, 0.3079598441704289313, 0.3333333333333333703, 0.3079598441704289313, 0.3333333333333333703, 0.3079598441704289313, 0.3333333333333333703, 0.3079598441704289313, 0.3333333333333333703, 0.3079598441704289313, 0.3333333333333333703, 0.3079598441704289313, 0.3333333333333333703, 0.3079598441704289313, 0.3333333333333333703, 0.3079598441704289313, 0.3333333333333333703, 0.3079598441704289313, 0.3333333333333333703, 0.3079598441704289313, 0.3333333333333333703, 0.3079598441704289313, 0.3333333333333333703, 0.3079598441704289313, 0.3333333333333333703, 0.3079598441704289313, 0.3333333333333333703, 0.3079598441704289313, 0.3333333333333333703, 0.3079598441704289313, 0.3333333333333333703, 0.3079598441704289313, 0.3333333333333333703, 0.3079598441704289313, 0.3333333333333333703, 0.3079598441704289313, 0.3333333333333333703, 0.3079598441704289313, 0.3333333333333333703, 0.3079598441704289313, 0.3333333333333333703, 0.3079598441704289313, 0.3333333333333333703, 0.3079598441704289313, 0.3333333333333333703, 0.3079598441704289313, 0.3333333333333333703, 0.3079598441704289313, 0.3333333333333333703, 0.3079598441704289313, 0.3333333333333333703, 0.3079598441704289313, 0.3333333333333333703, 0.3079598441704289313, 0.3333333333333333703, 0.3079598441704289313, 0.3333333333333333703, 0.3079598441704289313, 0.3333333333333333703, 0.3079598441704289313, 0.3333333333333333703, 0.3079598441704289313, 0.3333333333333333703, 0.3079598441704289313, 0.3333333333333333703, 0.3079598441704289313, 0.3333333333333333703, 0.3079598441704289313, 0.3333333333333333703, 0.3079598441704289313, 0.3333333333333333703, 0.3079598441704289313, 0.3333333333333333703, 0.3079598441704289313, 0.3333333333333333703, 0.3079598441704289313, 0.3333333333333333703, 0.3079598441704289313, 0.3333333333333333703, 0.3251605826665369681, 0.3222526856454325239),
 ( 0.3333333333333333703, 0.3079598441704289313, 0.3333333333333333703, 0.3079598441704289313, 0.3333333333333333703, 0.3079598441704289313, 0.3333333333333333703, 0.3079598441704289313, 0.3333333333333333703, 0.3079598441704289313, 0.3333333333333333703, 0.3079598441704289313, 0.3333333333333333703, 0.3079598441704289313, 0.3333333333333333703, 0.3079598441704289313, 0.3333333333333333703, 0.3079598441704289313, 0.3333333333333333703, 0.3079598441704289313, 0.3333333333333333703, 0.3079598441704289313, 0.3333333333333333703, 0.3079598441704289313, 0.3333333333333333703, 0.3079598441704289313, 0.3333333333333333703, 0.3079598441704289313, 0.3333333333333333703, 0.3079598441704289313, 0.3333333333333333703, 0.3079598441704289313, 0.3333333333333333703, 0.3079598441704289313, 0.3333333333333333703, 0.3079598441704289313, 0.3333333333333333703, 0.3079598441704289313, 0.3333333333333333703, 0.3079598441704289313, 0.3333333333333333703, 0.3079598441704289313, 0.3333333333333333703, 0.3079598441704289313, 0.3333333333333333703, 0.3079598441704289313, 0.3333333333333333703, 0.3079598441704289313, 0.3333333333333333703, 0.3079598441704289313, 0.3333333333333333703, 0.3079598441704289313, 0.3333333333333333703, 0.3079598441704289313, 0.3333333333333333703, 0.3079598441704289313, 0.3333333333333333703, 0.3079598441704289313, 0.3333333333333333703, 0.3079598441704289313, 0.3333333333333333703, 0.3079598441704289313, 0.3333333333333333703, 0.3079598441704289313, 0.3333333333333333703, 0.3079598441704289313, 0.3333333333333333703, 0.3079598441704289313, 0.3333333333333333703, 0.3079598441704289313, 0.3333333333333333703, 0.3079598441704289313, 0.3333333333333333703, 0.3079598441704289313, 0.3333333333333333703, 0.3079598441704289313, 0.3333333333333333703, 0.3079598441704289313, 0.3333333333333333703, 0.3079598441704289313, 0.3333333333333333703, 0.3079598441704289313, 0.3333333333333333703, 0.3079598441704289313, 0.3333333333333333703, 0.3079598441704289313, 0.3333333333333333703, 0.3079598441704289313, 0.3333333333333333703, 0.3079598441704289313, 0.3333333333333333703, 0.3079598441704289313, 0.3333333333333333703, 0.3251605826665369681, 0.3222526856454325239),
 ( 1.000000000000000000, 0.9238795325112867385, 1.000000000000000000, 0.9238795325112867385, 1.000000000000000000, 0.9238795325112867385, 1.000000000000000000, 0.9238795325112867385, 1.000000000000000000, 0.9238795325112867385, 1.000000000000000000, 0.9238795325112867385, 1.000000000000000000, 0.9238795325112867385, 1.000000000000000000, 0.9238795325112867385, 1.000000000000000000, 0.9238795325112867385, 1.000000000000000000, 0.9238795325112867385, 1.000000000000000000, 0.9238795325112867385, 1.000000000000000000, 0.9238795325112867385, 1.000000000000000000, 0.9238795325112867385, 1.000000000000000000, 0.9238795325112867385, 1.000000000000000000, 0.9238795325112867385, 1.000000000000000000, 0.9238795325112867385, 1.000000000000000000, 0.9238795325112867385, 1.000000000000000000, 0.9238795325112867385, 1.000000000000000000, 0.9238795325112867385, 1.000000000000000000, 0.9238795325112867385, 1.000000000000000000, 0.9238795325112867385, 1.000000000000000000, 0.9238795325112867385, 1.000000000000000000, 0.9238795325112867385, 1.000000000000000000, 0.9238795325112867385, 1.000000000000000000, 0.9238795325112867385, 1.000000000000000000, 0.9238795325112867385, 1.000000000000000000, 0.9238795325112867385, 1.000000000000000000, 0.9238795325112867385, 1.000000000000000000, 0.9238795325112867385, 1.000000000000000000, 0.9238795325112867385, 1.000000000000000000, 0.9238795325112867385, 1.000000000000000000, 0.9238795325112867385, 1.000000000000000000, 0.9238795325112867385, 1.000000000000000000, 0.9238795325112867385, 1.000000000000000000, 0.9238795325112867385, 1.000000000000000000, 0.9238795325112867385, 1.000000000000000000, 0.9238795325112867385, 1.000000000000000000, 0.9238795325112867385, 1.000000000000000000, 0.9238795325112867385, 1.000000000000000000, 0.9238795325112867385, 1.000000000000000000, 0.9238795325112867385, 1.000000000000000000, 0.9238795325112867385, 1.000000000000000000, 0.9238795325112867385, 1.000000000000000000, 0.9238795325112867385, 1.000000000000000000, 0.9238795325112867385, 1.000000000000000000, 0.9238795325112867385, 1.000000000000000000, 0.9754817479996107377, 0.9667580569362973497),
 ( 0.3333333333333333703, 0.3079598441704289313, 0.3333333333333333703, 0.3079598441704289313, 0.3333333333333333703, 0.3079598441704289313, 0.3333333333333333703, 0.3079598441704289313, 0.3333333333333333703, 0.3079598441704289313, 0.3333333333333333703, 0.3079598441704289313, 0.3333333333333333703, 0.3079598441704289313, 0.3333333333333333703, 0.3079598441704289313, 0.3333333333333333703, 0.3079598441704289313, 0.3333333333333333703, 0.3079598441704289313, 0.3333333333333333703, 0.3079598441704289313, 0.3333333333333333703, 0.3079598441704289313, 0.3333333333333333703, 0.3079598441704289313, 0.3333333333333333703, 0.3079598441704289313, 0.3333333333333333703, 0.3079598441704289313, 0.3333333333333333703, 0.3079598441704289313, 0.3333333333333333703, 0.3079598441704289313, 0.3333333333333333703, 0.3079598441704289313, 0.3333333333333333703, 0.3079598441704289313, 0.3333333333333333703, 0.3079598441704289313, 0.3333333333333333703, 0.3079598441704289313, 0.3333333333333333703, 0.3079598441704289313, 0.3333333333333333703, 0.3079598441704289313, 0.3333333333333333703, 0.3079598441704289313, 0.3333333333333333703, 0.3079598441704289313, 0.3333333333333333703, 0.3079598441704289313, 0.3333333333333333703, 0.3079598441704289313, 0.3333333333333333703, 0.3079598441704289313, 0.3333333333333333703, 0.3079598441704289313, 0.3333333333333333703, 0.3079598441704289313, 0.3333333333333333703, 0.3079598441704289313, 0.3333333333333333703, 0.3079598441704289313, 0.3333333333333333703, 0.3079598441704289313, 0.3333333333333333703, 0.3079598441704289313, 0.3333333333333333703, 0.3079598441704289313, 0.3333333333333333703, 0.3079598441704289313, 0.3333333333333333703, 0.3079598441704289313, 0.3333333333333333703, 0.3079598441704289313, 0.3333333333333333703, 0.3079598441704289313, 0.3333333333333333703, 0.3079598441704289313, 0.3333333333333333703, 0.3079598441704289313, 0.3333333333333333703, 0.3079598441704289313, 0.3333333333333333703, 0.3079598441704289313, 0.3333333333333333703, 0.3079598441704289313, 0.3333333333333333703, 0.3079598441704289313, 0.3333333333333333703, 0.3079598441704289313, 0.3333333333333333703, 0.3251605826665369681, 0.3222526856454325239),
 ( 0.3333333333333333703, 0.3079598441704289313, 0.3333333333333333703, 0.3079598441704289313, 0.3333333333333333703, 0.3079598441704289313, 0.3333333333333333703, 0.3079598441704289313, 0.3333333333333333703, 0.3079598441704289313, 0.3333333333333333703, 0.3079598441704289313, 0.3333333333333333703, 0.3079598441704289313, 0.3333333333333333703, 0.3079598441704289313, 0.3333333333333333703, 0.3079598441704289313, 0.3333333333333333703, 0.3079598441704289313, 0.3333333333333333703, 0.3079598441704289313, 0.3333333333333333703, 0.3079598441704289313, 0.3333333333333333703, 0.3079598441704289313, 0.3333333333333333703, 0.3079598441704289313, 0.3333333333333333703, 0.3079598441704289313, 0.3333333333333333703, 0.3079598441704289313, 0.3333333333333333703, 0.3079598441704289313, 0.3333333333333333703, 0.3079598441704289313, 0.3333333333333333703, 0.3079598441704289313, 0.3333333333333333703, 0.3079598441704289313, 0.3333333333333333703, 0.3079598441704289313, 0.3333333333333333703, 0.3079598441704289313, 0.3333333333333333703, 0.3079598441704289313, 0.3333333333333333703, 0.3079598441704289313, 0.3333333333333333703, 0.3079598441704289313, 0.3333333333333333703, 0.3079598441704289313, 0.3333333333333333703, 0.3079598441704289313, 0.3333333333333333703, 0.3079598441704289313, 0.3333333333333333703, 0.3079598441704289313, 0.3333333333333333703, 0.3079598441704289313, 0.3333333333333333703, 0.3079598441704289313, 0.3333333333333333703, 0.3079598441704289313, 0.3333333333333333703, 0.3079598441704289313, 0.3333333333333333703, 0.3079598441704289313, 0.3333333333333333703, 0.3079598441704289313, 0.3333333333333333703, 0.3079598441704289313, 0.3333333333333333703, 0.3079598441704289313, 0.3333333333333333703, 0.3079598441704289313, 0.3333333333333333703, 0.3079598441704289313, 0.3333333333333333703, 0.3079598441704289313, 0.3333333333333333703, 0.3079598441704289313, 0.3333333333333333703, 0.3079598441704289313, 0.3333333333333333703, 0.3079598441704289313, 0.3333333333333333703, 0.3079598441704289313, 0.3333333333333333703, 0.3079598441704289313, 0.3333333333333333703, 0.3079598441704289313, 0.3333333333333333703, 0.3251605826665369681, 0.3222526856454325239),
 ( 1.000000000000000000, 0.9238795325112867385, 1.000000000000000000, 0.9238795325112867385, 1.000000000000000000, 0.9238795325112867385, 1.000000000000000000, 0.9238795325112867385, 1.000000000000000000, 0.9238795325112867385, 1.000000000000000000, 0.9238795325112867385, 1.000000000000000000, 0.9238795325112867385, 1.000000000000000000, 0.9238795325112867385, 1.000000000000000000, 0.9238795325112867385, 1.000000000000000000, 0.9238795325112867385, 1.000000000000000000, 0.9238795325112867385, 1.000000000000000000, 0.9238795325112867385, 1.000000000000000000, 0.9238795325112867385, 1.000000000000000000, 0.9238795325112867385, 1.000000000000000000, 0.9238795325112867385, 1.000000000000000000, 0.9238795325112867385, 1.000000000000000000, 0.9238795325112867385, 1.000000000000000000, 0.9238795325112867385, 1.000000000000000000, 0.9238795325112867385, 1.000000000000000000, 0.9238795325112867385, 1.000000000000000000, 0.9238795325112867385, 1.000000000000000000, 0.9238795325112867385, 1.000000000000000000, 0.9238795325112867385, 1.000000000000000000, 0.9238795325112867385, 1.000000000000000000, 0.9238795325112867385, 1.000000000000000000, 0.9238795325112867385, 1.000000000000000000, 0.9238795325112867385, 1.000000000000000000, 0.9238795325112867385, 1.000000000000000000, 0.9238795325112867385, 1.000000000000000000, 0.9238795325112867385, 1.000000000000000000, 0.9238795325112867385, 1.000000000000000000, 0.9238795325112867385, 1.000000000000000000, 0.9238795325112867385, 1.000000000000000000, 0.9238795325112867385, 1.000000000000000000, 0.9238795325112867385, 1.000000000000000000, 0.9238795325112867385, 1.000000000000000000, 0.9238795325112867385, 1.000000000000000000, 0.9238795325112867385, 1.000000000000000000, 0.9238795325112867385, 1.000000000000000000, 0.9238795325112867385, 1.000000000000000000, 0.9238795325112867385, 1.000000000000000000, 0.9238795325112867385, 1.000000000000000000, 0.9238795325112867385, 1.000000000000000000, 0.9238795325112867385, 1.000000000000000000, 0.9238795325112867385, 1.000000000000000000, 0.9238795325112867385, 1.000000000000000000, 0.9754817479996107377, 0.9667580569362973497) ) ) 
 REPRESENTATION_ITEM ( '' )  SURFACE ( )  );
#17512=CARTESIAN_POINT ( 'NONE',  ( 0.5631383031621635116, -9.864917468222230923, 1.622643865078341907 ) ) ;
#17518=CARTESIAN_POINT ( 'NONE',  ( -12.34030858231679240, -22.67418626127525982, 5.270995438708342640 ) ) ;
#17521=CARTESIAN_POINT ( 'NONE',  ( 4.097191417683177406, -22.46490103525075810, 4.479004561291653808 ) ) ;
#17522=CARTESIAN_POINT ( 'NONE',  ( -13.12529397354238192, 5.014845663890295846, 4.833333333333344584 ) ) ;
#17523=CARTESIAN_POINT ( 'NONE',  ( -11.77780858231679417, -20.27099543870833642, 2.724438792969431589 ) ) ;
#17524=CARTESIAN_POINT ( 'NONE',  ( -7.190941417683177406, -23.80360840875937001, 5.231925497173365081 ) ) ;
#17525=ORIENTED_EDGE ( 'NONE', *, *, #17435, .T. ) ;
#17527=CARTESIAN_POINT ( 'NONE',  ( 13.37499999999998224, -19.50000000000006040, 4.416666666666682062 ) ) ;
#17528=FILL_AREA_STYLE ('',( #11158 ) ) ;
#17540=CARTESIAN_POINT ( 'NONE',  ( -0.5631383031621635116, -9.864917468222230923, 2.372643865078341019 ) ) ;
#17542=CARTESIAN_POINT ( 'NONE',  ( -11.30905858231679417, -23.27327832286945153, 2.298404588716537411 ) ) ;
#17545=CARTESIAN_POINT ( 'NONE',  ( 5.222191417683177406, -19.52099543870834353, 4.586221378810406257 ) ) ;
#17547=CARTESIAN_POINT ( 'NONE',  ( -12.44094141768317741, -21.25705176302044208, 2.828734674606458555 ) ) ;
#17549=CARTESIAN_POINT ( 'NONE',  ( 6.527808582316794173, -23.72900456129165647, 4.275561207030568411 ) ) ;
#17552=CARTESIAN_POINT ( 'NONE',  ( -12.69740987707854707, -17.34330120752609616, 6.298537912489285517 ) ) ;
#17555=CARTESIAN_POINT ( 'NONE',  ( 4.746558582316793284, -21.94931252712234482, 5.250000000000000888 ) ) ;
#17560=( NAMED_UNIT ( * ) SI_UNIT ( $, .STERADIAN. ) SOLID_ANGLE_UNIT ( ) );
#17561=VERTEX_POINT ( 'NONE', #4013 ) ;
#17564=CARTESIAN_POINT ( 'NONE',  ( -6.059058582316793284, -20.72672167713054137, 4.701595411283463477 ) ) ;
#17565=CARTESIAN_POINT ( 'NONE',  ( 12.64691428603184242, -19.14332855539073464, 5.509795676248469221 ) ) ;
#17567=CARTESIAN_POINT ( 'NONE',  ( 1.407845757905374695, -9.114917468222230923, 1.622643865078341463 ) ) ;
#17571=CARTESIAN_POINT ( 'NONE',  ( -13.84497512400090891, 4.233743762047977199, 5.032110966142367303 ) ) ;
#17572=CARTESIAN_POINT ( 'NONE',  ( 5.684058582316794173, -20.79840458871652942, 2.226721677130544030 ) ) ;
#17573=CARTESIAN_POINT ( 'NONE',  ( -13.90439735423812273, 5.734566389025032684, 4.666666666666618113 ) ) ;
#17575=CARTESIAN_POINT ( 'NONE',  ( -5.402808582316795949, -23.08622137881038938, 1.020995438708339309 ) ) ;
#17576=CARTESIAN_POINT ( 'NONE',  ( 8.402808582316794173, -22.77556120703056308, 1.770995438708339975 ) ) ;
#17577=CARTESIAN_POINT ( 'NONE',  ( 7.847191417683175629, -21.53509896474923835, 2.520995438708346192 ) ) ;
#17578=CARTESIAN_POINT ( 'NONE',  ( -9.347191417683177406, -21.22443879296941915, 1.770995438708345748 ) ) ;
#17580=CARTESIAN_POINT ( 'NONE',  ( 13.84501469867711698, 4.235742283194553259, 4.166666666666765551 ) ) ;
#17588=CARTESIAN_POINT ( 'NONE',  ( -13.10821839766814279, 4.152529082241303904, 5.997503362667785609 ) ) ;
#17589=CARTESIAN_POINT ( 'NONE',  ( -1.797604806073912709, -9.120796646272857799, 2.374153755450133740 ) ) ;
#17594=CARTESIAN_POINT ( 'NONE',  ( -12.62524871736568954, -20.23743977303344010, 4.661898514667671023 ) ) ;
#17597=CARTESIAN_POINT ( 'NONE',  ( 13.04271272860988340, 0.09449279482665236263, 6.673537912489449830 ) ) ;
#17598=CARTESIAN_POINT ( 'NONE',  ( -1.837882866761050282, -9.938290523052360825, 2.391487531332776140 ) ) ;
#17600=CARTESIAN_POINT ( 'NONE',  ( -13.87470623115321899, 4.985164673244912414, 4.958488177337359026 ) ) ;
#17602=CARTESIAN_POINT ( 'NONE',  ( 5.128441417683177406, -19.49999999999998934, 3.550687472877664952 ) ) ;
#17603=CARTESIAN_POINT ( 'NONE',  ( -6.909691417683176518, -21.63647391050456648, 4.520995438708348857 ) ) ;
#17604=B_SPLINE_CURVE_WITH_KNOTS ( 'NONE', 3,
 ( #8257, #14835, #507, #6888, #13258, #18678, #5815, #4454, #12185, #20357, #10933, #13851, #4346, #7799, #20154, #17299, #20469, #7491, #6126, #10729, #18989, #18890, #20254, #16993, #10839, #14059, #12495, #2984, #17102, #9158 ),
 .UNSPECIFIED., .F., .F.,
 ( 4, 2, 2, 2, 2, 2, 2, 2, 2, 2, 2, 2, 2, 2, 4 ),
 ( 0.6078525888943429045, 0.6200887121040892236, 0.6309950902025724950, 0.6419014683010558775, 0.6637142244980225314, 0.7073397368919559502, 0.7509652492858893691, 0.7727780054828560230, 0.7836843835813394055, 0.7945907616798226769, 0.8074288390748337596, 0.8202669164698448423, 0.8459430712598670077, 0.8972953808399113385, 1.000000000000000000 ),
 .UNSPECIFIED. ) ;
#17606=CARTESIAN_POINT ( 'NONE',  ( 13.90411326029870409, 5.720219645086723759, 5.230514352905474063 ) ) ;
#17607=CARTESIAN_POINT ( 'NONE',  ( 13.00900269284621302, -0.8578640112522492034, 5.903024842915844062 ) ) ;
#17617=CARTESIAN_POINT ( 'NONE',  ( 2.627360420079438263, -14.25085146736906339, 2.749039333894452763 ) ) ;
#17624=CARTESIAN_POINT ( 'NONE',  ( -2.579281110863027582, -9.822567596814183233, 2.554382554832406615 ) ) ;
#17625=CARTESIAN_POINT ( 'NONE',  ( 9.059058582316795949, -21.25705176302045274, 4.171265325393551215 ) ) ;
#17626=CARTESIAN_POINT ( 'NONE',  ( -13.08080186171710224, 3.517994016715657146, 5.247095106674282583 ) ) ;
#17627=CARTESIAN_POINT ( 'NONE',  ( -12.52780858231679595, -23.72900456129165647, 4.275561207030568411 ) ) ;
#17628=CARTESIAN_POINT ( 'NONE',  ( -6.628441417683177406, -19.49999999999998934, 3.550687472877664952 ) ) ;
#17629=EDGE_LOOP ( 'NONE', ( #12079, #14411 ) ) ;
#17630=CARTESIAN_POINT ( 'NONE',  ( 13.57153706873194032, -9.574878029060977624, 4.950999963380944280 ) ) ;
#17633=ORIENTED_EDGE ( 'NONE', *, *, #20543, .T. ) ;
#17634=FACE_OUTER_BOUND ( 'NONE', #14491, .T. ) ;
#17639=VERTEX_POINT ( 'NONE', #15606 ) ;
#17640=CARTESIAN_POINT ( 'NONE',  ( 11.12844141768317741, -20.24999999999999289, 3.550687472877664952 ) ) ;
#17642=CARTESIAN_POINT ( 'NONE',  ( -1.337453470010121714, -9.114917468222230923, 2.372643865078341019 ) ) ;
#17643=CARTESIAN_POINT ( 'NONE',  ( 2.623717082130370137, -10.12934627674766830, 2.633169448359191644 ) ) ;
#17647=CARTESIAN_POINT ( 'NONE',  ( 7.472191417683176518, -23.72900456129165292, 2.724438792969417822 ) ) ;
#17650=CARTESIAN_POINT ( 'NONE',  ( -11.50344141768317741, -22.05068747287766229, 4.499999999999999112 ) ) ;
#17652=CARTESIAN_POINT ( 'NONE',  ( 8.309058582316795949, -23.80360840875935935, 1.768074502826626260 ) ) ;
#17654=CARTESIAN_POINT ( 'NONE',  ( -13.90439735423812273, 5.734566389025032684, 4.333333333333380999 ) ) ;
#17656=CARTESIAN_POINT ( 'NONE',  ( 6.246558582316794173, -21.94931252712234482, 5.250000000000000888 ) ) ;
#17668=CARTESIAN_POINT ( 'NONE',  ( -12.80905858231679417, -23.80360840875935935, 1.768074502826626260 ) ) ;
#17672=CARTESIAN_POINT ( 'NONE',  ( 2.155282726790247239, -12.05525952636828357, 2.935167462089139256 ) ) ;
#17674=CARTESIAN_POINT ( 'NONE',  ( 12.62499999998404121, -20.24999999996810729, 2.793053905886972998 ) ) ;
#17677=CARTESIAN_POINT ( 'NONE',  ( -13.38090111944825367, -19.20199346786276351, 4.743968713382380464 ) ) ;
#17679=CARTESIAN_POINT ( 'NONE',  ( 9.996558582316794173, -22.05068747287764452, 1.749999999999998446 ) ) ;
#17680=CARTESIAN_POINT ( 'NONE',  ( -13.90439735423465351, 5.734566389025032684, 3.333333333332063386 ) ) ;
#17683=CARTESIAN_POINT ( 'NONE',  ( -7.652808582316796837, -20.91377862118960351, 5.979004561291660913 ) ) ;
#17684=CARTESIAN_POINT ( 'NONE',  ( 8.215308582316792396, -23.77099543870833998, 2.825813738724734847 ) ) ;
#17685=CARTESIAN_POINT ( 'NONE',  ( 6.722191417683176518, -21.02099543870834353, 3.964901035250761208 ) ) ;
#17686=CARTESIAN_POINT ( 'NONE',  ( -8.784691417683177406, -23.77099543870834353, 4.174186261275251830 ) ) ;
#17689=CARTESIAN_POINT ( 'NONE',  ( 13.83531008031826026, 3.745659056069631898, 5.237458296715707284 ) ) ;
#17696=CARTESIAN_POINT ( 'NONE',  ( -13.12119116326504908, 4.807653744879115010, 5.626470997801169105 ) ) ;
#17698=CARTESIAN_POINT ( 'NONE',  ( -0.9854920305337621089, -9.114917468222230923, 2.372643865078341019 ) ) ;
#17702=CARTESIAN_POINT ( 'NONE',  ( -13.12270769621861355, 4.884238659038159902, 5.513847264053151065 ) ) ;
#17703=CARTESIAN_POINT ( 'NONE',  ( 12.24655858231679240, -21.94931252712234482, 5.250000000000000888 ) ) ;
#17705=CARTESIAN_POINT ( 'NONE',  ( 12.85087781109329974, -9.593170539812428288, 6.465204579154565145 ) ) ;
#17707=CARTESIAN_POINT ( 'NONE',  ( -2.327620134574780231, -13.27885108724501251, 3.249410218619480872 ) ) ;
#17711=CARTESIAN_POINT ( 'NONE',  ( -13.87470602645761986, 4.985154336109792972, 4.333333333333382775 ) ) ;
#17713=CARTESIAN_POINT ( 'NONE',  ( 6.159691417683175629, -22.98484643305507191, 0.9790045612916508100 ) ) ;
#17714=CARTESIAN_POINT ( 'NONE',  ( -8.402808582316797725, -22.46490103525074034, 2.520995438708341307 ) ) ;
#17717=CARTESIAN_POINT ( 'NONE',  ( 13.85956729540471066, 3.470648417939721231, 6.731609435864099211 ) ) ;
#17718=CARTESIAN_POINT ( 'NONE',  ( 13.12529397354238192, 5.014845663890295846, 4.833333333333344584 ) ) ;
#17719=CARTESIAN_POINT ( 'NONE',  ( -13.12500000000000533, 4.265117264764102245, 4.000000000000000888 ) ) ;
#17730=CARTESIAN_POINT ( 'NONE',  ( 2.196516900615978152, -11.19187256518208784, 1.963432442569047698 ) ) ;
#17733=AXIS2_PLACEMENT_3D ( 'NONE', #19939, #13435, #10303 ) ;
#17734=EDGE_CURVE ( 'NONE', #8562, #19322, #10557, .T. ) ;
#17738=CARTESIAN_POINT ( 'NONE',  ( -12.24655858231679240, -21.94931252712234482, 5.250000000000000888 ) ) ;
#17740=CARTESIAN_POINT ( 'NONE',  ( -1.824488249492779879, -9.124319963227819130, 2.375058613629473570 ) ) ;
#17741=CARTESIAN_POINT ( 'NONE',  ( -13.09123688038123490, 4.044962459253448550, 5.255034774807352704 ) ) ;
#17742=CARTESIAN_POINT ( 'NONE',  ( -12.24655858231679240, -21.94931252712234482, 5.250000000000000888 ) ) ;
#17743=CARTESIAN_POINT ( 'NONE',  ( -4.659691417683178294, -22.67418626127524917, 1.729004561291651809 ) ) ;
#17745=CARTESIAN_POINT ( 'NONE',  ( 13.84042474920106081, 4.003949834653575124, 5.242612001278796008 ) ) ;
#17754=CARTESIAN_POINT ( 'NONE',  ( 9.159691417683177406, -22.67418626127524917, 1.729004561291651587 ) ) ;
#17756=CARTESIAN_POINT ( 'NONE',  ( -1.957016269584227031, -9.152392576945766578, 2.382268221639079364 ) ) ;
#17757=CARTESIAN_POINT ( 'NONE',  ( 2.203959450683124377, -9.262433282444222371, 2.410528873095051594 ) ) ;
#17758=CARTESIAN_POINT ( 'NONE',  ( -12.99655858231679417, -22.05068747287764452, 1.749999999999998446 ) ) ;
#17761=CARTESIAN_POINT ( 'NONE',  ( 9.253441417683177406, -21.94931252712233061, 1.749999999999998446 ) ) ;
#17763=CARTESIAN_POINT ( 'NONE',  ( -5.784691417683179182, -23.77099543870834353, 4.174186261275252718 ) ) ;
#17766=CARTESIAN_POINT ( 'NONE',  ( 11.87155858231679595, -19.49999999999998934, 3.449312527122348371 ) ) ;
#17767=CARTESIAN_POINT ( 'NONE',  ( 12.64511805349267526, -19.23403829861753422, 5.507852591554869726 ) ) ;
#17768=CARTESIAN_POINT ( 'NONE',  ( -13.15492785973632017, 5.761356916681801721, 5.116543252045025802 ) ) ;
#17776=CARTESIAN_POINT ( 'NONE',  ( 12.74617908753018192, -19.97389846102915456, 3.534610772493881559 ) ) ;
#17778=CARTESIAN_POINT ( 'NONE',  ( -7.652808582316795061, -21.22443879296942626, 5.229004561291659137 ) ) ;
#17780=CARTESIAN_POINT ( 'NONE',  ( 12.62524871736568954, -20.23743977303344010, 4.661898514667671023 ) ) ;
#17782=CARTESIAN_POINT ( 'NONE',  ( 13.08573665985359824, 3.017201322601628100, 5.986358176248492313 ) ) ;
#17784=CARTESIAN_POINT ( 'NONE',  ( -13.84501469867711698, 4.235742283194553259, 2.999999999999999556 ) ) ;
#17785=CARTESIAN_POINT ( 'NONE',  ( 8.684058582316795949, -20.26807450282662160, 1.696391591240633101 ) ) ;
#17786=CARTESIAN_POINT ( 'NONE',  ( -13.15498566372047762, 5.764276017890828108, 4.942557026581394730 ) ) ;
#17787=CARTESIAN_POINT ( 'NONE',  ( -11.87844141768317741, -24.50000000000000000, 3.449312527122335048 ) ) ;
#17790=CARTESIAN_POINT ( 'NONE',  ( 4.068047865639282890, -21.50414067263875850, 5.566613268849052609 ) ) ;
#17792=CARTESIAN_POINT ( 'NONE',  ( 8.027808582316795949, -22.97900456129165647, 3.964901035250747885 ) ) ;
#17793=CARTESIAN_POINT ( 'NONE',  ( -6.065941417683177406, -23.20159541128344927, 2.226721677130534705 ) ) ;
#17796=CARTESIAN_POINT ( 'NONE',  ( 13.37561105820882013, -20.21914156045197686, 4.753815841436231260 ) ) ;
#17804=CARTESIAN_POINT ( 'NONE',  ( -13.12529380813666435, 5.014837310896125722, 5.033295791462342628 ) ) ;
#17806=CARTESIAN_POINT ( 'NONE',  ( -3.475298211275419380, -9.785109117490691233, 1.987377451789144933 ) ) ;
#17808=CARTESIAN_POINT ( 'NONE',  ( 2.012076196476103362, -9.160103213191565175, 1.634248467062433541 ) ) ;
#17809=CARTESIAN_POINT ( 'NONE',  ( -12.62499999999998224, -20.25000000000006395, 4.416666666666681174 ) ) ;
#17810=CARTESIAN_POINT ( 'NONE',  ( 8.871558582316794173, -20.24999999999999289, 3.449312527122348371 ) ) ;
#17812=CARTESIAN_POINT ( 'NONE',  ( 12.62515553039088090, -20.24214571525854467, 4.629702272822510345 ) ) ;
#17816=CARTESIAN_POINT ( 'NONE',  ( -13.83544900551672185, 3.002674778589386140, 5.971513032956590195 ) ) ;
#17818=CARTESIAN_POINT ( 'NONE',  ( 4.472191417683178294, -24.47900456129165292, 2.413778621189595963 ) ) ;
#17819=CARTESIAN_POINT ( 'NONE',  ( -7.652808582316796837, -21.53509896474924901, 4.479004561291659137 ) ) ;
#17821=CARTESIAN_POINT ( 'NONE',  ( 13.90439735423465351, 5.734566389025032684, 3.333333333332063386 ) ) ;
#17822=CARTESIAN_POINT ( 'NONE',  ( 13.09293046926041626, 3.380488697651010011, 5.994170676248444352 ) ) ;
#17830=DIRECTION ( 'NONE',  ( 0.1351665943404306014, 0.9596796555888912339, -0.2464649070825229438 ) ) ;
#17831=CARTESIAN_POINT ( 'NONE',  ( 2.050137595624097031, -10.15260257655714504, 1.696527147986202522 ) ) ;
#17841=CARTESIAN_POINT ( 'NONE',  ( -12.63598464672302590, -18.94527534048458151, 4.764022190007618285 ) ) ;
#17842=CARTESIAN_POINT ( 'NONE',  ( -5.402808582316795949, -22.46490103525074034, 2.520995438708341307 ) ) ;
#17843=CARTESIAN_POINT ( 'NONE',  ( -9.253441417683177406, -21.94931252712233061, 1.749999999999998446 ) ) ;
#17845=CARTESIAN_POINT ( 'NONE',  ( 13.84167967300649238, 4.067323486828401613, 5.231641758301140754 ) ) ;
#17855=CARTESIAN_POINT ( 'NONE',  ( 7.097191417683177406, -22.77556120703057729, 5.229004561291656472 ) ) ;
#17857=CARTESIAN_POINT ( 'NONE',  ( -2.702705060698113115, -10.69015907548275379, 2.777197378435510622 ) ) ;
#17858=CARTESIAN_POINT ( 'NONE',  ( 2.534747216115884161, -9.671180236796224960, 2.515503256513427210 ) ) ;
#17859=CARTESIAN_POINT ( 'NONE',  ( -9.152808582316794173, -21.22443879296942626, 5.229004561291660025 ) ) ;
#17861=CARTESIAN_POINT ( 'NONE',  ( 11.50344141768317563, -22.05068747287765873, 5.250000000000000888 ) ) ;
#17863=CARTESIAN_POINT ( 'NONE',  ( -5.034691417683178294, -20.22900456129164581, 2.825813738724747726 ) ) ;
#17865=CARTESIAN_POINT ( 'NONE',  ( 9.246558582316795949, -21.94931252712234127, 6.000000000000001776 ) ) ;
#17866=CARTESIAN_POINT ( 'NONE',  ( 12.91308523408712183, -5.701695678577235249, 5.798858176249892082 ) ) ;
#17867=CARTESIAN_POINT ( 'NONE',  ( -12.62499999999998224, -20.24999999999991829, 4.333333333333343695 ) ) ;
#17872=SURFACE_STYLE_USAGE ( .BOTH. , #9204 ) ;
#17878=CARTESIAN_POINT ( 'NONE',  ( -5.590308582316794173, -21.32581373872472597, 1.729004561291657582 ) ) ;
#17879=CARTESIAN_POINT ( 'NONE',  ( 13.12503131243110843, 5.001581277770153378, 5.166347330538456184 ) ) ;
#17882=CARTESIAN_POINT ( 'NONE',  ( 13.15498530132288479, 5.764257716805535559, 4.916666666666649199 ) ) ;
#17883=CARTESIAN_POINT ( 'NONE',  ( 4.687312169500630787, -21.51559725698340131, 5.182386163300424009 ) ) ;
#17884=CARTESIAN_POINT ( 'NONE',  ( -13.37597619100657198, -20.20070235416671167, 4.815535977982682070 ) ) ;
#17885=CARTESIAN_POINT ( 'NONE',  ( 12.24655858231679595, -21.94931252712234127, 6.000000000000001776 ) ) ;
#17886=CARTESIAN_POINT ( 'NONE',  ( -13.12519991495504712, 4.260095705229160146, 6.739971950528219402 ) ) ;
#17887=CARTESIAN_POINT ( 'NONE',  ( -5.590308582316795949, -21.01515356694490322, 0.9790045612916562501 ) ) ;
#17891=CARTESIAN_POINT ( 'NONE',  ( 12.62155858231679417, -22.99999999999999645, 3.550687472877652073 ) ) ;
#17892=CARTESIAN_POINT ( 'NONE',  ( -9.065941417683177406, -23.20159541128344927, 2.226721677130534705 ) ) ;
#17895=CARTESIAN_POINT ( 'NONE',  ( 13.84042474920106081, 4.003949834653575124, 5.242612001278796008 ) ) ;
#17902=CARTESIAN_POINT ( 'NONE',  ( 13.81626551376501588, 2.033908445126689557, 5.950679699622869911 ) ) ;
#17906=CARTESIAN_POINT ( 'NONE',  ( -12.62599079447150885, -20.19996487918709249, 4.820256282269618886 ) ) ;
#17907=CARTESIAN_POINT ( 'NONE',  ( 7.559058582316794173, -20.72672167713054137, 4.701595411283463477 ) ) ;
#17909=CARTESIAN_POINT ( 'NONE',  ( 13.12503131243110843, 5.001581277770153378, 5.166347330538456184 ) ) ;
#17910=CARTESIAN_POINT ( 'NONE',  ( -1.743623630681728542, -9.116095536440919744, 2.372946416531167557 ) ) ;
#17911=CARTESIAN_POINT ( 'NONE',  ( -13.84863765609603625, 3.668701632846259830, 5.985835949623216301 ) ) ;
#17913=CARTESIAN_POINT ( 'NONE',  ( 10.19094141768317563, -23.27327832286946219, 4.701595411283453707 ) ) ;
#17914=CARTESIAN_POINT ( 'NONE',  ( -6.152808582316795949, -21.53509896474924901, 4.479004561291659137 ) ) ;
#17916=CARTESIAN_POINT ( 'NONE',  ( 12.62499999999998224, -20.99999999999998934, 4.166666666666637653 ) ) ;
#17917=CARTESIAN_POINT ( 'NONE',  ( 13.12529397354238192, 5.014845663890295846, 3.666666666666500873 ) ) ;
#17927=CARTESIAN_POINT ( 'NONE',  ( 2.031432063436913182, -10.08997855658269671, 1.680444048616273722 ) ) ;
#17929=EDGE_CURVE ( 'NONE', #14618, #17122, #11931, .T. ) ;
#17931=CARTESIAN_POINT ( 'NONE',  ( 12.73406432005743305, -20.51439999008355741, 3.536278562595261299 ) ) ;
#17933=CARTESIAN_POINT ( 'NONE',  ( -8.684058582316794173, -20.79840458871652942, 2.226721677130544030 ) ) ;
#17934=CARTESIAN_POINT ( 'NONE',  ( -3.302240162463773832, -9.695145533921818881, 2.714273006325518711 ) ) ;
#17936=CARTESIAN_POINT ( 'NONE',  ( -12.63036675113625407, -19.22897906761645004, 4.757923088130392664 ) ) ;
#17938=CARTESIAN_POINT ( 'NONE',  ( -11.30905858231679417, -23.27327832286945153, 2.298404588716537411 ) ) ;
#17939=CARTESIAN_POINT ( 'NONE',  ( -8.128441417683175629, -20.24999999999999289, 3.550687472877664952 ) ) ;
#17941=CARTESIAN_POINT ( 'NONE',  ( 13.83710853266996388, 3.836480899831821834, 5.239411421715695738 ) ) ;
#17942=( LENGTH_UNIT ( ) NAMED_UNIT ( * ) SI_UNIT ( .MILLI., .METRE. ) );
#17957=CARTESIAN_POINT ( 'NONE',  ( 10.09719141768317741, -22.77556120703057729, 5.229004561291655584 ) ) ;
#17960=CARTESIAN_POINT ( 'NONE',  ( -4.753441417683176518, -21.94931252712233061, 1.749999999999998446 ) ) ;
#17962=CARTESIAN_POINT ( 'NONE',  ( 11.02780858231679595, -24.47900456129166358, 4.586221378810390270 ) ) ;
#17963=CARTESIAN_POINT ( 'NONE',  ( 13.10624331898488037, 4.052787608736739600, 6.006964772046813117 ) ) ;
#17964=CARTESIAN_POINT ( 'NONE',  ( -12.62503117662529739, -20.24842558042254836, 4.565011198945062354 ) ) ;
#17974=CARTESIAN_POINT ( 'NONE',  ( 12.76889623635853788, -19.95450346923866647, 3.531415919227487432 ) ) ;
#17978=CARTESIAN_POINT ( 'NONE',  ( 13.10821839766814279, 4.152529082241303904, 5.997503362667785609 ) ) ;
#17982=CARTESIAN_POINT ( 'NONE',  ( 12.66849571425264287, -18.05346643024382303, 5.533233176248494978 ) ) ;
#17984=CARTESIAN_POINT ( 'NONE',  ( 10.65280858231679595, -20.91377862118960351, 5.979004561291660913 ) ) ;
#17985=CARTESIAN_POINT ( 'NONE',  ( -12.62499999999998224, -20.24999999999998934, 4.166666666666636765 ) ) ;
#17987=CARTESIAN_POINT ( 'NONE',  ( -11.12844141768317741, -19.49999999999998934, 3.550687472877664952 ) ) ;
#17991=CARTESIAN_POINT ( 'NONE',  ( 12.52780858231679773, -22.97900456129165647, 3.964901035250747885 ) ) ;
#17992=CARTESIAN_POINT ( 'NONE',  ( -4.378441417683176518, -23.74999999999999645, 3.449312527122335492 ) ) ;
#17996=CARTESIAN_POINT ( 'NONE',  ( 13.84504075139246915, 3.487057945321567765, 5.981929699623240282 ) ) ;
#17997=AXIS2_PLACEMENT_3D ( 'NONE', #822, #11799, #8668 ) ;
#18003=CARTESIAN_POINT ( 'NONE',  ( 13.37597619100657198, -20.20070235416671167, 4.815535977982682070 ) ) ;
#18007=CARTESIAN_POINT ( 'NONE',  ( 3.365018999794965548, -10.14078633184679923, 2.828722465802024910 ) ) ;
#18010=CARTESIAN_POINT ( 'NONE',  ( -12.62500000000002132, -19.49999999999450040, 3.833333333368183382 ) ) ;
#18011=CARTESIAN_POINT ( 'NONE',  ( 9.527808582316794173, -23.72900456129165292, 4.275561207030568411 ) ) ;
#18014=CARTESIAN_POINT ( 'NONE',  ( 12.68288333306630378, -17.32689168014509207, 5.548858176248425700 ) ) ;
#18017=CARTESIAN_POINT ( 'NONE',  ( 11.02780858231679595, -22.97900456129165647, 3.964901035250747885 ) ) ;
#18018=CARTESIAN_POINT ( 'NONE',  ( 8.784691417683177406, -23.77099543870834353, 4.174186261275252718 ) ) ;
#18019=CARTESIAN_POINT ( 'NONE',  ( -7.934058582316796837, -22.67126532539354855, 4.242948236979545484 ) ) ;
#18021=CARTESIAN_POINT ( 'NONE',  ( 13.90439771357353038, 5.734584535470497180, 4.942866369314573127 ) ) ;
#18022=CARTESIAN_POINT ( 'NONE',  ( 13.12529397354238192, 5.014845663890295846, 4.583333333333296622 ) ) ;
#18034=CARTESIAN_POINT ( 'NONE',  ( 1.717920576997000737, -9.114924032904250240, 2.372645551019823884 ) ) ;
#18039=AXIS2_PLACEMENT_3D ( 'NONE', #1793, #16229, #8180 ) ;
#18041=CARTESIAN_POINT ( 'NONE',  ( -7.184058582316794173, -20.79840458871652942, 2.226721677130544030 ) ) ;
#18042=CARTESIAN_POINT ( 'NONE',  ( -2.171407406650392780, -8.432416083433171394, 2.389978857884845986 ) ) ;
#18045=CARTESIAN_POINT ( 'NONE',  ( -12.62917185724685254, -19.28932120903463598, 4.753410794856941735 ) ) ;
#18046=CARTESIAN_POINT ( 'NONE',  ( -10.09030858231679595, -21.32581373872472597, 1.729004561291657582 ) ) ;
#18049=CARTESIAN_POINT ( 'NONE',  ( -7.097191417683177406, -22.77556120703057729, 5.229004561291655584 ) ) ;
#18051=CARTESIAN_POINT ( 'NONE',  ( 13.84495141469777479, 4.232546442235974204, 5.040078719623224401 ) ) ;
#18056=ORIENTED_EDGE ( 'NONE', *, *, #9240, .T. ) ;
#18059=ADVANCED_FACE ( 'NONE', ( #13552 ), #15021, .F. ) ;
#18063=CARTESIAN_POINT ( 'NONE',  ( 4.940941417683177406, -20.72672167713052715, 2.298404588716546293 ) ) ;
#18069=CARTESIAN_POINT ( 'NONE',  ( 12.62499999998404299, -20.99999999996810729, 2.793053905886972998 ) ) ;
#18070=DIRECTION ( 'NONE',  ( 0.000000000000000000, 0.000000000000000000, 1.000000000000000000 ) ) ;
#18071=CARTESIAN_POINT ( 'NONE',  ( 9.815941417683177406, -20.79840458871654363, 4.773278322869464851 ) ) ;
#18073=CARTESIAN_POINT ( 'NONE',  ( -9.159691417683175629, -22.36352608949543352, 2.479004561291652031 ) ) ;
#18075=CARTESIAN_POINT ( 'NONE',  ( -7.090308582316795061, -21.01515356694490322, 0.9790045612916562501 ) ) ;
#18077=CARTESIAN_POINT ( 'NONE',  ( 13.08094078691552831, 2.775009739235173356, 5.981149842915306714 ) ) ;
#18078=CARTESIAN_POINT ( 'NONE',  ( -13.13084019862132479, 4.544930030374419339, 6.677052771569639944 ) ) ;
#18088=CARTESIAN_POINT ( 'NONE',  ( 13.26617719913702587, -19.98584313357335773, 3.463688470049236745 ) ) ;
#18092=CARTESIAN_POINT ( 'NONE',  ( 12.65650603190776025, -18.65894538865861563, 5.520212342915047365 ) ) ;
#18097=CARTESIAN_POINT ( 'NONE',  ( 13.15498530132288479, 5.764257716805535559, 4.666666666666618113 ) ) ;
#18099=CARTESIAN_POINT ( 'NONE',  ( 12.71530858231679417, -24.52099543870834708, 2.515153566944913432 ) ) ;
#18100=CARTESIAN_POINT ( 'NONE',  ( -12.62499999999998401, -20.24999999999998934, 2.439580858552613751 ) ) ;
#18101=CARTESIAN_POINT ( 'NONE',  ( -7.378441417683177406, -24.50000000000000000, 3.449312527122335048 ) ) ;
#18106=CARTESIAN_POINT ( 'NONE',  ( 7.090308582316795061, -21.63647391050454871, 2.479004561291657804 ) ) ;
#18111=CARTESIAN_POINT ( 'NONE',  ( 13.87470602645761986, 4.985154336109792972, 3.000000000000000000 ) ) ;
#18119=CARTESIAN_POINT ( 'NONE',  ( 13.85593616229004610, 4.037276195647738319, 5.992122970672676630 ) ) ;
#18121=CARTESIAN_POINT ( 'NONE',  ( 1.513434189748285918, -8.364917468222230923, 2.372643865078341019 ) ) ;
#18123=CARTESIAN_POINT ( 'NONE',  ( -12.62500000000002132, -19.50000000000273559, 4.083333333315724012 ) ) ;
#18124=CARTESIAN_POINT ( 'NONE',  ( 6.434058582316794173, -23.20159541128345992, 4.773278322869455970 ) ) ;
#18126=CARTESIAN_POINT ( 'NONE',  ( 13.05696142222617695, 1.564051822406025583, 5.955108176248398166 ) ) ;
#18128=CARTESIAN_POINT ( 'NONE',  ( -0.2815691515810352930, -9.114917468222230923, 2.372643865078523984 ) ) ;
#18129=CARTESIAN_POINT ( 'NONE',  ( 10.46530858231679595, -20.97900456129165647, 3.863526089495444626 ) ) ;
#18130=CARTESIAN_POINT ( 'NONE',  ( 10.56594141768317741, -23.20159541128344927, 2.226721677130534705 ) ) ;
#18131=CARTESIAN_POINT ( 'NONE',  ( -12.52780858231679595, -23.72900456129165647, 4.275561207030568411 ) ) ;
#18133=CARTESIAN_POINT ( 'NONE',  ( 13.12860732321105139, 4.432169822159808703, 6.709107302035562270 ) ) ;
#18134=CARTESIAN_POINT ( 'NONE',  ( 12.63478567848856571, -19.00582323632600890, 4.762720106674273701 ) ) ;
#18143=CARTESIAN_POINT ( 'NONE',  ( 1.700193846275138032, -9.865151716929458914, 2.372704024825938340 ) ) ;
#18144=DIRECTION ( 'NONE',  ( 0.000000000000000000, -0.000000000000000000, -1.000000000000000000 ) ) ;
#18146=CARTESIAN_POINT ( 'NONE',  ( 13.37500000067116268, -20.29298605568190084, 3.448842523571910679 ) ) ;
#18147=CARTESIAN_POINT ( 'NONE',  ( -2.567175533087980188, -9.771398394011347577, 2.541241281345096859 ) ) ;
#18148=CARTESIAN_POINT ( 'NONE',  ( -8.590308582316794173, -21.32581373872472597, 1.729004561291657582 ) ) ;
#18149=CARTESIAN_POINT ( 'NONE',  ( -3.636036383999129207, -10.90885478516162976, 2.275977788322152584 ) ) ;
#18151=CARTESIAN_POINT ( 'NONE',  ( -13.37503747255156306, -19.49810763614315690, 4.531249681074674740 ) ) ;
#18152=CARTESIAN_POINT ( 'NONE',  ( -8.402808582316794173, -22.77556120703056308, 1.770995438708339975 ) ) ;
#18154=CARTESIAN_POINT ( 'NONE',  ( -6.722191417683177406, -20.27099543870833998, 4.275561207030583510 ) ) ;
#18156=CARTESIAN_POINT ( 'NONE',  ( 13.38921792038197900, -19.53199502070850357, 5.456033026503027017 ) ) ;
#18168=CARTESIAN_POINT ( 'NONE',  ( 4.066879903460562495, -13.96783368734915776, 3.061584679647603391 ) ) ;
#18169=CARTESIAN_POINT ( 'NONE',  ( -7.465308582316795061, -20.22900456129164937, 4.174186261275266929 ) ) ;
#18170=CARTESIAN_POINT ( 'NONE',  ( 13.90439735423812273, 5.734566389025032684, 4.791666666666684726 ) ) ;
#18174=CARTESIAN_POINT ( 'NONE',  ( 10.00344141768317741, -22.05068747287766229, 4.499999999999999112 ) ) ;
#18175=CARTESIAN_POINT ( 'NONE',  ( -12.64387510712649565, -19.29680709011273976, 5.506486987317513737 ) ) ;
#18176=CARTESIAN_POINT ( 'NONE',  ( -9.347191417683177406, -21.53509896474923835, 2.520995438708346192 ) ) ;
#18177=CARTESIAN_POINT ( 'NONE',  ( -6.152808582316795949, -20.91377862118960351, 5.979004561291660913 ) ) ;
#18179=CARTESIAN_POINT ( 'NONE',  ( 13.10821839766814279, 4.152529082241303904, 5.997503362667785609 ) ) ;
#18180=CARTESIAN_POINT ( 'NONE',  ( -12.62499999999998401, -20.24999999999998934, 2.439580858552613751 ) ) ;
#18182=CARTESIAN_POINT ( 'NONE',  ( 0.000000000000000000, -9.114917468222230923, 2.372643865078340575 ) ) ;
#18186=CARTESIAN_POINT ( 'NONE',  ( 13.06532418593161893, -19.87503328927329704, 3.491089126739379989 ) ) ;
#18189=CARTESIAN_POINT ( 'NONE',  ( 13.12512971825177033, 5.006550771716304915, 5.133277049491872468 ) ) ;
#18191=CARTESIAN_POINT ( 'NONE',  ( -0.9854920305337622199, -8.364917468222230923, 1.622643865078341907 ) ) ;
#18194=( BOUNDED_SURFACE ( )  B_SPLINE_SURFACE ( 3, 3, ( 
 ( #6670, #10112, #16086, #16487, #2159, #14401, #84, #182, #6472, #17643, #3318, #4884, #8142, #14504, #16284, #6566, #3426, #17858, #4990, #1855, #11369, #17757, #13041, #11478, #1955, #13646, #18581, #899, #5404, #18482, #7396, #8951, #16579, #18269, #8755, #13549, #18380, #17001, #11776, #11878 ),
 ( #8643, #4143, #5608, #15017, #15223, #19950, #11980, #19852, #20159, #8542, #3931, #4043, #8856, #10624, #12090, #20056, #5503, #14913, #698, #15325, #10317, #7084, #1004, #16686, #7284, #13758, #2366, #15126, #589, #5721, #13448, #10526, #16895, #19746, #10428, #6975, #16796, #2565, #802, #5822 ),
 ( #13345, #18168, #7185, #3833, #12189, #2465, #4245, #10212, #2257, #15534, #17107, #11045, #1422, #20259, #9262, #18685, #15841, #9065, #1218, #20573, #15633, #1320, #5919, #7899, #15435, #4352, #10938, #18793, #17207, #12702, #4555, #14261, #3095, #18996, #2990, #7698, #10737, #12400, #1519, #17306 ),
 ( #13858, #2884, #20669, #9470, #2787, #20475, #4459, #6328, #1119, #7496, #10844, #2677, #4653, #19105, #4759, #11144, #9163, #12290, #14066, #17419, #7593, #13959, #12596, #20363, #18896, #6026, #6131, #12500, #9366, #6225, #15741, #7804, #14166, #11239, #5167, #19413, #8214, #14577, #13118, #468 ),
 ( #6750, #17617, #12807, #2032, #19516, #17730, #8422, #3288, #3398, #8309, #19205, #14790, #13212, #17831, #11548, #9670, #12902, #17927, #6442, #6843, #3596, #15939, #13012, #9566, #19611, #9777, #3498, #364, #9976, #14479, #3194, #16056, #16357, #5072, #250, #6641, #5266, #17512, #158, #1619 ),
 ( #4858, #8000, #14370, #16164, #57, #1729, #1827, #14684, #8113, #6541, #19307, #9876, #4962, #11341, #11449, #16259, #1926, #7365, #13728, #20133, #774, #20027, #666, #15096, #4012, #19825, #16461, #18143, #2135, #8516, #7159, #16769, #977, #10398, #14886, #875, #10499, #12063, #19715, #7055 ),
 ( #563, #13314, #10186, #10286, #6942, #16868, #11751, #7258, #8726, #3808, #18349, #2335, #16656, #2231, #2538, #11645, #13420, #13523, #11952, #8927, #5375, #5479, #16556, #2439, #3907, #4117, #11852, #8616, #18034, #3704, #19925, #8831, #15198, #15297, #5581, #10087, #14988, #18244, #13620, #5689 ) ),
 .UNSPECIFIED., .T., .F., .F. ) 
 B_SPLINE_SURFACE_WITH_KNOTS ( ( 4, 3, 4 ),
 ( 4, 2, 2, 2, 2, 2, 2, 2, 2, 2, 2, 2, 2, 2, 2, 2, 2, 2, 2, 4 ),
 ( 0.000000000000000000, 0.5000000000000000000, 1.000000000000000000 ),
 ( 0.000000000000000000, 0.3100443560520446118, 0.4650665340780669177, 0.5425776230910780429, 0.5813331675975836887, 0.6007109398508364562, 0.6200887121040892236, 0.6309950902025724950, 0.6419014683010558775, 0.6637142244980225314, 0.7073397368919559502, 0.7509652492858893691, 0.7727780054828560230, 0.7836843835813394055, 0.7945907616798226769, 0.8074288390748337596, 0.8202669164698448423, 0.8459430712598670077, 0.8972953808399113385, 1.000000000000000000 ),
 .UNSPECIFIED. ) 
 GEOMETRIC_REPRESENTATION_ITEM ( )  RATIONAL_B_SPLINE_SURFACE ( (
 ( 1.000000000000000000, 1.000000000000000000, 1.000000000000000000, 1.000000000000000000, 1.000000000000000000, 1.000000000000000000, 1.000000000000000000, 1.000000000000000000, 1.000000000000000000, 1.000000000000000000, 1.000000000000000000, 1.000000000000000000, 1.000000000000000000, 1.000000000000000000, 1.000000000000000000, 1.000000000000000000, 1.000000000000000000, 1.000000000000000000, 1.000000000000000000, 1.000000000000000000, 1.000000000000000000, 1.000000000000000000, 1.000000000000000000, 1.000000000000000000, 1.000000000000000000, 1.000000000000000000, 1.000000000000000000, 1.000000000000000000, 1.000000000000000000, 1.000000000000000000, 1.000000000000000000, 1.000000000000000000, 1.000000000000000000, 1.000000000000000000, 1.000000000000000000, 1.000000000000000000, 1.000000000000000000, 1.000000000000000000, 1.000000000000000000, 1.000000000000000000),
 ( 0.3333333333333333703, 0.3333333333333333703, 0.3333333333333333703, 0.3333333333333333703, 0.3333333333333333703, 0.3333333333333333703, 0.3333333333333333703, 0.3333333333333333703, 0.3333333333333333703, 0.3333333333333333703, 0.3333333333333333703, 0.3333333333333333703, 0.3333333333333333703, 0.3333333333333333703, 0.3333333333333333703, 0.3333333333333333703, 0.3333333333333333703, 0.3333333333333333703, 0.3333333333333333703, 0.3333333333333333703, 0.3333333333333333703, 0.3333333333333333703, 0.3333333333333333703, 0.3333333333333333703, 0.3333333333333333703, 0.3333333333333333703, 0.3333333333333333703, 0.3333333333333333703, 0.3333333333333333703, 0.3333333333333333703, 0.3333333333333333703, 0.3333333333333333703, 0.3333333333333333703, 0.3333333333333333703, 0.3333333333333333703, 0.3333333333333333703, 0.3333333333333333703, 0.3333333333333333703, 0.3333333333333333703, 0.3333333333333333703),
 ( 0.3333333333333333703, 0.3333333333333333703, 0.3333333333333333703, 0.3333333333333333703, 0.3333333333333333703, 0.3333333333333333703, 0.3333333333333333703, 0.3333333333333333703, 0.3333333333333333703, 0.3333333333333333703, 0.3333333333333333703, 0.3333333333333333703, 0.3333333333333333703, 0.3333333333333333703, 0.3333333333333333703, 0.3333333333333333703, 0.3333333333333333703, 0.3333333333333333703, 0.3333333333333333703, 0.3333333333333333703, 0.3333333333333333703, 0.3333333333333333703, 0.3333333333333333703, 0.3333333333333333703, 0.3333333333333333703, 0.3333333333333333703, 0.3333333333333333703, 0.3333333333333333703, 0.3333333333333333703, 0.3333333333333333703, 0.3333333333333333703, 0.3333333333333333703, 0.3333333333333333703, 0.3333333333333333703, 0.3333333333333333703, 0.3333333333333333703, 0.3333333333333333703, 0.3333333333333333703, 0.3333333333333333703, 0.3333333333333333703),
 ( 1.000000000000000000, 1.000000000000000000, 1.000000000000000000, 1.000000000000000000, 1.000000000000000000, 1.000000000000000000, 1.000000000000000000, 1.000000000000000000, 1.000000000000000000, 1.000000000000000000, 1.000000000000000000, 1.000000000000000000, 1.000000000000000000, 1.000000000000000000, 1.000000000000000000, 1.000000000000000000, 1.000000000000000000, 1.000000000000000000, 1.000000000000000000, 1.000000000000000000, 1.000000000000000000, 1.000000000000000000, 1.000000000000000000, 1.000000000000000000, 1.000000000000000000, 1.000000000000000000, 1.000000000000000000, 1.000000000000000000, 1.000000000000000000, 1.000000000000000000, 1.000000000000000000, 1.000000000000000000, 1.000000000000000000, 1.000000000000000000, 1.000000000000000000, 1.000000000000000000, 1.000000000000000000, 1.000000000000000000, 1.000000000000000000, 1.000000000000000000),
 ( 0.3333333333333333703, 0.3333333333333333703, 0.3333333333333333703, 0.3333333333333333703, 0.3333333333333333703, 0.3333333333333333703, 0.3333333333333333703, 0.3333333333333333703, 0.3333333333333333703, 0.3333333333333333703, 0.3333333333333333703, 0.3333333333333333703, 0.3333333333333333703, 0.3333333333333333703, 0.3333333333333333703, 0.3333333333333333703, 0.3333333333333333703, 0.3333333333333333703, 0.3333333333333333703, 0.3333333333333333703, 0.3333333333333333703, 0.3333333333333333703, 0.3333333333333333703, 0.3333333333333333703, 0.3333333333333333703, 0.3333333333333333703, 0.3333333333333333703, 0.3333333333333333703, 0.3333333333333333703, 0.3333333333333333703, 0.3333333333333333703, 0.3333333333333333703, 0.3333333333333333703, 0.3333333333333333703, 0.3333333333333333703, 0.3333333333333333703, 0.3333333333333333703, 0.3333333333333333703, 0.3333333333333333703, 0.3333333333333333703),
 ( 0.3333333333333333703, 0.3333333333333333703, 0.3333333333333333703, 0.3333333333333333703, 0.3333333333333333703, 0.3333333333333333703, 0.3333333333333333703, 0.3333333333333333703, 0.3333333333333333703, 0.3333333333333333703, 0.3333333333333333703, 0.3333333333333333703, 0.3333333333333333703, 0.3333333333333333703, 0.3333333333333333703, 0.3333333333333333703, 0.3333333333333333703, 0.3333333333333333703, 0.3333333333333333703, 0.3333333333333333703, 0.3333333333333333703, 0.3333333333333333703, 0.3333333333333333703, 0.3333333333333333703, 0.3333333333333333703, 0.3333333333333333703, 0.3333333333333333703, 0.3333333333333333703, 0.3333333333333333703, 0.3333333333333333703, 0.3333333333333333703, 0.3333333333333333703, 0.3333333333333333703, 0.3333333333333333703, 0.3333333333333333703, 0.3333333333333333703, 0.3333333333333333703, 0.3333333333333333703, 0.3333333333333333703, 0.3333333333333333703),
 ( 1.000000000000000000, 1.000000000000000000, 1.000000000000000000, 1.000000000000000000, 1.000000000000000000, 1.000000000000000000, 1.000000000000000000, 1.000000000000000000, 1.000000000000000000, 1.000000000000000000, 1.000000000000000000, 1.000000000000000000, 1.000000000000000000, 1.000000000000000000, 1.000000000000000000, 1.000000000000000000, 1.000000000000000000, 1.000000000000000000, 1.000000000000000000, 1.000000000000000000, 1.000000000000000000, 1.000000000000000000, 1.000000000000000000, 1.000000000000000000, 1.000000000000000000, 1.000000000000000000, 1.000000000000000000, 1.000000000000000000, 1.000000000000000000, 1.000000000000000000, 1.000000000000000000, 1.000000000000000000, 1.000000000000000000, 1.000000000000000000, 1.000000000000000000, 1.000000000000000000, 1.000000000000000000, 1.000000000000000000, 1.000000000000000000, 1.000000000000000000) ) ) 
 REPRESENTATION_ITEM ( '' )  SURFACE ( )  );
#18195=CARTESIAN_POINT ( 'NONE',  ( 13.12529397354238192, 5.014845663890295846, 4.583333333333296622 ) ) ;
#18199=CARTESIAN_POINT ( 'NONE',  ( 6.434058582316796837, -23.73192549717337130, 5.303608408759367343 ) ) ;
#18200=CARTESIAN_POINT ( 'NONE',  ( -13.10985494974158705, 3.485174961951963191, 6.746454579156001330 ) ) ;
#18201=CARTESIAN_POINT ( 'NONE',  ( -9.440941417683177406, -20.19639159124061933, 1.768074502826635586 ) ) ;
#18206=CARTESIAN_POINT ( 'NONE',  ( 12.34030858231679773, -22.36352608949544418, 4.520995438708343528 ) ) ;
#18210=CARTESIAN_POINT ( 'NONE',  ( 13.40382044110196347, -18.79456772435387890, 5.502763032956559108 ) ) ;
#18216=CARTESIAN_POINT ( 'NONE',  ( 13.39542766346049518, -19.21840299524461315, 5.493648449623241170 ) ) ;
#18219=CARTESIAN_POINT ( 'NONE',  ( 4.066879903460562495, -13.96783368734915776, 3.061584679647603391 ) ) ;
#18222=CARTESIAN_POINT ( 'NONE',  ( -13.12512971825177033, 5.006550771716304915, 5.133277049491872468 ) ) ;
#18225=CARTESIAN_POINT ( 'NONE',  ( 12.69247507894198712, -16.84250851341299082, 5.559274842915185033 ) ) ;
#18227=CARTESIAN_POINT ( 'NONE',  ( 12.43405858231679595, -22.67126532539354855, 4.242948236979545484 ) ) ;
#18229=CARTESIAN_POINT ( 'NONE',  ( 9.722191417683177406, -20.27099543870833998, 4.275561207030583510 ) ) ;
#18230=CARTESIAN_POINT ( 'NONE',  ( -10.65280858231679240, -21.22443879296942626, 5.229004561291659137 ) ) ;
#18232=CARTESIAN_POINT ( 'NONE',  ( 12.65017171054692113, -19.72882861737994631, 6.192581331858542981 ) ) ;
#18233=CARTESIAN_POINT ( 'NONE',  ( 12.62499999999998224, -19.49999999999998934, 4.291666666666699825 ) ) ;
#18244=CARTESIAN_POINT ( 'NONE',  ( 0.5631383031621635116, -9.114917468222230923, 2.372643865078341019 ) ) ;
#18247=CARTESIAN_POINT ( 'NONE',  ( 13.20683383907801733, -20.56345410174260735, 3.472004214064662975 ) ) ;
#18248=CARTESIAN_POINT ( 'NONE',  ( -2.559937518207947793, -9.746075135043517079, 2.534737762559237773 ) ) ;
#18249=CARTESIAN_POINT ( 'NONE',  ( -9.527808582316792396, -23.72900456129165647, 4.275561207030568411 ) ) ;
#18250=CARTESIAN_POINT ( 'NONE',  ( -3.537356407578672535, -11.36437789272258669, 3.142965222332344766 ) ) ;
#18253=CARTESIAN_POINT ( 'NONE',  ( -13.57153706873194032, -9.574878029060977624, 4.950999963380944280 ) ) ;
#18254=CARTESIAN_POINT ( 'NONE',  ( -5.027808582316793284, -23.72900456129165647, 4.275561207030568411 ) ) ;
#18256=CARTESIAN_POINT ( 'NONE',  ( -9.253441417683177406, -21.94931252712233061, 2.499999999999999112 ) ) ;
#18258=CARTESIAN_POINT ( 'NONE',  ( 13.41820805991576826, -18.06799297425606454, 5.518388032956592859 ) ) ;
#18260=ORIENTED_EDGE ( 'NONE', *, *, #20136, .F. ) ;
#18264=CARTESIAN_POINT ( 'NONE',  ( -13.38238173943565990, -19.87722215849730034, 5.285856107751903288 ) ) ;
#18266=CARTESIAN_POINT ( 'NONE',  ( 5.034691417683179182, -20.22900456129164581, 2.825813738724748170 ) ) ;
#18269=CARTESIAN_POINT ( 'NONE',  ( 1.407845757905374695, -9.114917468222230923, 2.372643865078341019 ) ) ;
#18272=CARTESIAN_POINT ( 'NONE',  ( 12.64802275499843454, -19.83735087257960927, 6.157588447769994922 ) ) ;
#18274=CARTESIAN_POINT ( 'NONE',  ( 9.253441417683177406, -21.94931252712233061, 2.499999999999999112 ) ) ;
#18276=CARTESIAN_POINT ( 'NONE',  ( -4.003441417683175629, -22.05068747287766229, 4.499999999999999112 ) ) ;
#18277=CARTESIAN_POINT ( 'NONE',  ( -8.972191417683177406, -24.47900456129165292, 2.413778621189595963 ) ) ;
#18279=CARTESIAN_POINT ( 'NONE',  ( 12.62917185724685254, -19.28932120903463598, 4.753410794856941735 ) ) ;
#18280=CARTESIAN_POINT ( 'NONE',  ( -13.12503131243110843, 5.001581277770153378, 5.166347330538456184 ) ) ;
#18291=CARTESIAN_POINT ( 'NONE',  ( -2.830107938415192148, -10.43856789473369950, 1.962583737180462418 ) ) ;
#18294=CARTESIAN_POINT ( 'NONE',  ( 13.09293046926041626, 3.380488697651010011, 5.994170676248444352 ) ) ;
#18295=CYLINDRICAL_SURFACE ( 'NONE', #3337, 0.3750000000000003331 ) ;
#18296=CARTESIAN_POINT ( 'NONE',  ( 5.871558582316795949, -19.49999999999998934, 3.449312527122348371 ) ) ;
#18297=CARTESIAN_POINT ( 'NONE',  ( -12.72125031657057015, -15.38935901321805133, 5.590524842915047365 ) ) ;
#18298=CARTESIAN_POINT ( 'NONE',  ( -9.815941417683177406, -20.26807450282663225, 5.303608408759377113 ) ) ;
#18300=CARTESIAN_POINT ( 'NONE',  ( 12.15280858231679595, -21.22443879296942626, 5.229004561291659137 ) ) ;
#18302=CARTESIAN_POINT ( 'NONE',  ( -13.86316420010827777, 3.652292105464413297, 6.735515685864076119 ) ) ;
#18304=CARTESIAN_POINT ( 'NONE',  ( 5.496558582316795949, -22.05068747287764452, 2.499999999999999112 ) ) ;
#18308=CARTESIAN_POINT ( 'NONE',  ( 13.87470586348985258, 4.985146106231644225, 5.033049509202228933 ) ) ;
#18318=CARTESIAN_POINT ( 'NONE',  ( 13.12499999999999467, 5.000000000000047073, 3.999999999999996447 ) ) ;
#18319=CARTESIAN_POINT ( 'NONE',  ( 13.40382044110196347, -18.79456772435387890, 5.502763032956559108 ) ) ;
#18320=( BOUNDED_CURVE ( )  B_SPLINE_CURVE ( 3, ( #14368, #15631, #11141, #12594 ),
 .UNSPECIFIED., .F., .T. ) 
 B_SPLINE_CURVE_WITH_KNOTS ( ( 4, 4 ),
 ( 0.000000000000000000, 1.468430546537837468E-05 ),
 .UNSPECIFIED. ) 
 CURVE ( )  GEOMETRIC_REPRESENTATION_ITEM ( )  RATIONAL_B_SPLINE_CURVE ( ( 1.000000000000000000, 0.9870550161812301493, 0.9743613912715626268, 0.9619191252709974327 ) ) 
 REPRESENTATION_ITEM ( '' )  );
#18322=CARTESIAN_POINT ( 'NONE',  ( 0.5631383031621635116, -9.114917468222230923, 2.372643865078341019 ) ) ;
#18324=CARTESIAN_POINT ( 'NONE',  ( -12.64917329730235096, -18.27924848622803466, 4.778345106674467324 ) ) ;
#18325=CARTESIAN_POINT ( 'NONE',  ( 13.87500000000000178, 5.000000000000047962, 4.000000000000000000 ) ) ;
#18327=CARTESIAN_POINT ( 'NONE',  ( -13.85956729540471066, 3.470648417939721231, 6.731609435864099211 ) ) ;
#18330=CARTESIAN_POINT ( 'NONE',  ( 12.62155858231679417, -22.99999999999999645, 3.550687472877652073 ) ) ;
#18333=CARTESIAN_POINT ( 'NONE',  ( 6.253441417683176518, -21.94931252712233061, 1.749999999999998446 ) ) ;
#18334=CARTESIAN_POINT ( 'NONE',  ( -4.717959273841179524, -21.82295283170803302, 4.493595146365858994 ) ) ;
#18336=CARTESIAN_POINT ( 'NONE',  ( 13.14123030749026277, 5.069630528265579805, 6.418963484850015000 ) ) ;
#18337=CARTESIAN_POINT ( 'NONE',  ( 12.65396917024039958, -18.03705690286155772, 4.783553440007634272 ) ) ;
#18349=CARTESIAN_POINT ( 'NONE',  ( 2.616536356806028696, -10.07836329504444706, 2.620076000170431296 ) ) ;
#18353=CARTESIAN_POINT ( 'NONE',  ( -6.340308582316793284, -22.67418626127525982, 5.270995438708342640 ) ) ;
#18355=CARTESIAN_POINT ( 'NONE',  ( -1.948765222931501784, -9.143197003266354983, 1.629906614618163552 ) ) ;
#18358=CARTESIAN_POINT ( 'NONE',  ( -13.09560264576187905, 4.265433610975056133, 4.791666666666684726 ) ) ;
#18359=CARTESIAN_POINT ( 'NONE',  ( -6.996558582316793284, -22.05068747287764452, 1.749999999999998446 ) ) ;
#18361=CARTESIAN_POINT ( 'NONE',  ( 12.43405858231679595, -23.73192549717337130, 5.303608408759367343 ) ) ;
#18362=CARTESIAN_POINT ( 'NONE',  ( -11.87844141768317741, -22.99999999999999645, 3.449312527122335048 ) ) ;
#18366=CARTESIAN_POINT ( 'NONE',  ( 13.85528666703740619, 4.004476685417483139, 5.993048563355776182 ) ) ;
#18369=VERTEX_POINT ( 'NONE', #12192 ) ;
#18378=CIRCLE ( 'NONE', #19383, 0.3749999999999997224 ) ;
#18380=CARTESIAN_POINT ( 'NONE',  ( 0.9854920305337621089, -9.114917468222230923, 2.372643865078341019 ) ) ;
#18384=CARTESIAN_POINT ( 'NONE',  ( 12.62505438222622622, -20.99725369757571869, 4.613400783263607252 ) ) ;
#18386=CARTESIAN_POINT ( 'NONE',  ( 3.944195004867016241, -21.61378581760806838, 5.207602947182413899 ) ) ;
#18387=CARTESIAN_POINT ( 'NONE',  ( -12.62499999999998579, -20.24999999999999289, 3.666666666666653640 ) ) ;
#18388=CARTESIAN_POINT ( 'NONE',  ( -8.034691417683175629, -20.97900456129164581, 3.136473910504570917 ) ) ;
#18389=CARTESIAN_POINT ( 'NONE',  ( -11.31594141768317741, -20.26807450282663225, 5.303608408759377113 ) ) ;
#18391=CARTESIAN_POINT ( 'NONE',  ( 13.12529397354238192, 5.014845663890295846, 4.583333333333296622 ) ) ;
#18392=CARTESIAN_POINT ( 'NONE',  ( -13.12529397354238192, 5.014845663890295846, 4.791666666666685614 ) ) ;
#18403=CARTESIAN_POINT ( 'NONE',  ( -2.780192134145684779, -10.08406280675441735, 1.871539748636713130 ) ) ;
#18407=CARTESIAN_POINT ( 'NONE',  ( 12.53469141768317741, -19.47900456129164581, 2.515153566944927199 ) ) ;
#18408=CARTESIAN_POINT ( 'NONE',  ( -13.10372118337080849, 3.925419760224517329, 6.005889426248455010 ) ) ;
#18409=CARTESIAN_POINT ( 'NONE',  ( -8.784691417683177406, -24.52099543870834708, 4.484846433055073689 ) ) ;
#18411=CIRCLE ( 'NONE', #8064, 0.3749999999999998890 ) ;
#18413=CARTESIAN_POINT ( 'NONE',  ( 13.27780858231679595, -20.27099543870833642, 2.724438792969431589 ) ) ;
#18415=CARTESIAN_POINT ( 'NONE',  ( -13.40653076352726103, -19.40769644187082932, 6.236886054669082746 ) ) ;
#18416=CARTESIAN_POINT ( 'NONE',  ( 12.71530858231679240, -23.77099543870833998, 2.825813738724734847 ) ) ;
#18420=CARTESIAN_POINT ( 'NONE',  ( 13.39662663169496781, -19.15785509940297615, 5.494950532956567102 ) ) ;
#18427=CARTESIAN_POINT ( 'NONE',  ( 13.87444723674697755, 4.972085455720938185, 5.163895512850782410 ) ) ;
#18429=CARTESIAN_POINT ( 'NONE',  ( 1.126276606324276619, -9.114917468222230923, 2.372643865078341019 ) ) ;
#18432=CARTESIAN_POINT ( 'NONE',  ( -12.63478567848856571, -19.00582323632600890, 4.762720106674273701 ) ) ;
#18435=CARTESIAN_POINT ( 'NONE',  ( -13.41475008041063433, -18.99262093926051520, 6.248536519197435801 ) ) ;
#18437=CARTESIAN_POINT ( 'NONE',  ( 10.84030858231679240, -22.67418626127525982, 5.270995438708342640 ) ) ;
#18440=CARTESIAN_POINT ( 'NONE',  ( 5.878441417683177406, -23.74999999999999645, 3.449312527122335492 ) ) ;
#18441=CARTESIAN_POINT ( 'NONE',  ( -11.02780858231679595, -23.72900456129165647, 4.275561207030568411 ) ) ;
#18443=CARTESIAN_POINT ( 'NONE',  ( 12.64183575740756993, -20.14979425091403087, 6.022201559249563907 ) ) ;
#18445=CARTESIAN_POINT ( 'NONE',  ( 12.89855869007488209, -5.685286151195387383, 5.049178440009032265 ) ) ;
#18450=CARTESIAN_POINT ( 'NONE',  ( -12.63249216759192350, -19.87164553660301536, 5.297612231341934041 ) ) ;
#18451=CARTESIAN_POINT ( 'NONE',  ( -3.277163086644854229, -14.76879761173520578, 3.824673233536266537 ) ) ;
#18455=CARTESIAN_POINT ( 'NONE',  ( -12.62672070884157804, -20.24999999999991473, 3.550922209436377042 ) ) ;
#18458=CARTESIAN_POINT ( 'NONE',  ( 4.413027396565882832, -21.45855829990031438, 5.554906804930435982 ) ) ;
#18459=CARTESIAN_POINT ( 'NONE',  ( -10.84030858231679595, -22.98484643305508612, 6.020995438708344416 ) ) ;
#18460=CARTESIAN_POINT ( 'NONE',  ( -1.407845757905374695, -9.114917468222230923, 1.622643865078341463 ) ) ;
#18462=CARTESIAN_POINT ( 'NONE',  ( -13.79214722387705905, 1.565934805775630601, 5.190583296715636230 ) ) ;
#18465=CARTESIAN_POINT ( 'NONE',  ( 11.59719141768317741, -23.08622137881040359, 5.979004561291654696 ) ) ;
#18466=CARTESIAN_POINT ( 'NONE',  ( -9.909691417683175629, -21.63647391050456648, 4.520995438708348857 ) ) ;
#18468=CARTESIAN_POINT ( 'NONE',  ( 13.37500000000002132, -20.24999999999450040, 3.833333333368183382 ) ) ;
#18475=CARTESIAN_POINT ( 'NONE',  ( -13.39902456816392906, -19.03675930772010361, 5.497554699623231400 ) ) ;
#18476=EDGE_LOOP ( 'NONE', ( #18808, #692, #2873, #7710, #15037, #14494 ) ) ;
#18482=CARTESIAN_POINT ( 'NONE',  ( 1.655860418491166941, -9.114909740826840689, 2.372641880528837621 ) ) ;
#18484=CARTESIAN_POINT ( 'NONE',  ( 13.90439735423812273, 5.734566389025032684, 4.666666666666618113 ) ) ;
#18488=CARTESIAN_POINT ( 'NONE',  ( 9.815941417683177406, -21.32873467460645145, 4.242948236979555254 ) ) ;
#18489=CARTESIAN_POINT ( 'NONE',  ( -12.62745083560477966, -20.12623280195927933, 5.001038150054709419 ) ) ;
#18490=CARTESIAN_POINT ( 'NONE',  ( -7.378441417683177406, -22.99999999999999645, 3.449312527122335048 ) ) ;
#18491=CARTESIAN_POINT ( 'NONE',  ( -5.121558582316795061, -24.50000000000000000, 3.550687472877651629 ) ) ;
#18493=CARTESIAN_POINT ( 'NONE',  ( 12.78345773956433895, -11.49788415197707181, 4.924178440007425550 ) ) ;
#18494=CARTESIAN_POINT ( 'NONE',  ( -12.72125031657057015, -15.38935901321805133, 5.590524842915047365 ) ) ;
#18508=CARTESIAN_POINT ( 'NONE',  ( -1.407845757905374695, -9.114917468222230923, 1.622643865078341463 ) ) ;
#18512=CARTESIAN_POINT ( 'NONE',  ( 4.934058582316795061, -23.73192549717337130, 5.303608408759367343 ) ) ;
#18513=CARTESIAN_POINT ( 'NONE',  ( -12.65650603190776025, -18.65894538865861563, 5.520212342915047365 ) ) ;
#18514=CARTESIAN_POINT ( 'NONE',  ( -6.065941417683177406, -23.73192549717336064, 1.696391591240623331 ) ) ;
#18516=CARTESIAN_POINT ( 'NONE',  ( 11.96530858231679595, -20.22900456129164937, 4.174186261275266929 ) ) ;
#18518=CARTESIAN_POINT ( 'NONE',  ( -13.41475008041063433, -18.99262093926051520, 6.248536519197435801 ) ) ;
#18520=CARTESIAN_POINT ( 'NONE',  ( 6.527808582316795949, -22.97900456129165647, 3.964901035250747885 ) ) ;
#18524=CARTESIAN_POINT ( 'NONE',  ( 13.37500000000002132, -21.00000000000274269, 4.083333333315724012 ) ) ;
#18529=CARTESIAN_POINT ( 'NONE',  ( -9.059058582316794173, -20.72672167713054137, 4.701595411283463477 ) ) ;
#18530=CARTESIAN_POINT ( 'NONE',  ( 13.87454419214980739, 4.976981703567351367, 5.131312659523921127 ) ) ;
#18532=CARTESIAN_POINT ( 'NONE',  ( 2.722060606927515725, -8.660968749821154944, 1.698675748411476283 ) ) ;
#18534=CARTESIAN_POINT ( 'NONE',  ( -13.09123688038123490, 4.044962459253448550, 5.255034774807352704 ) ) ;
#18535=CARTESIAN_POINT ( 'NONE',  ( 13.18405858231679417, -20.79840458871652942, 2.226721677130544030 ) ) ;
#18536=CARTESIAN_POINT ( 'NONE',  ( -13.87005939078915873, 4.000499234880882327, 6.742989431566016378 ) ) ;
#18538=CARTESIAN_POINT ( 'NONE',  ( 11.87155858231679417, -20.24999999999999289, 3.449312527122348371 ) ) ;
#18540=CARTESIAN_POINT ( 'NONE',  ( 5.503441417683176518, -22.05068747287765873, 5.250000000000000888 ) ) ;
#18541=CARTESIAN_POINT ( 'NONE',  ( -8.871558582316794173, -20.24999999999999289, 3.449312527122348371 ) ) ;
#18543=CARTESIAN_POINT ( 'NONE',  ( 12.78345773956433895, -11.49788415197707181, 4.924178440007425550 ) ) ;
#18548=CARTESIAN_POINT ( 'NONE',  ( -12.62500016093973620, -20.24999187254239175, 4.532396751752561848 ) ) ;
#18551=CARTESIAN_POINT ( 'NONE',  ( -13.38450946332969771, -19.76977210184853462, 5.359796180098093998 ) ) ;
#18553=CARTESIAN_POINT ( 'NONE',  ( -12.62499999999998579, -20.24999999999999289, 3.146526952850934755 ) ) ;
#18556=CARTESIAN_POINT ( 'NONE',  ( -1.619022621591187150, -9.114917468222230923, 2.372643865078341019 ) ) ;
#18557=CARTESIAN_POINT ( 'NONE',  ( -8.402808582316797725, -23.08622137881038938, 1.020995438708339309 ) ) ;
#18558=CARTESIAN_POINT ( 'NONE',  ( -1.126276606324276619, -8.364917468222230923, 1.622643865078341907 ) ) ;
#18559=ORIENTED_EDGE ( 'NONE', *, *, #1187, .F. ) ;
#18560=CARTESIAN_POINT ( 'NONE',  ( -13.09560264576187905, 4.265433610975056133, 4.833333333333343695 ) ) ;
#18562=CARTESIAN_POINT ( 'NONE',  ( 11.12844141768317741, -19.49999999999998934, 3.550687472877664952 ) ) ;
#18563=CARTESIAN_POINT ( 'NONE',  ( -8.128441417683177406, -20.99999999999999645, 3.550687472877664952 ) ) ;
#18565=CARTESIAN_POINT ( 'NONE',  ( 13.84501469867711698, 4.235742283194553259, 2.999999999999999556 ) ) ;
#18573=CARTESIAN_POINT ( 'NONE',  ( -13.87470602645761986, 4.985154336109792972, 4.916666666666650087 ) ) ;
#18581=CARTESIAN_POINT ( 'NONE',  ( 1.797604806073912709, -9.120796646272857799, 2.374153755450133740 ) ) ;
#18583=CARTESIAN_POINT ( 'NONE',  ( 13.11704875914858270, 3.848462337001107070, 6.754267079155989784 ) ) ;
#18587=CARTESIAN_POINT ( 'NONE',  ( 11.50344141768317741, -22.05068747287766229, 4.499999999999999112 ) ) ;
#18588=CARTESIAN_POINT ( 'NONE',  ( -12.62500000000001954, -20.25000000000274269, 4.083333333315724012 ) ) ;
#18589=CARTESIAN_POINT ( 'NONE',  ( -8.777808582316797725, -21.02099543870833998, 3.035098964749253003 ) ) ;
#18590=CARTESIAN_POINT ( 'NONE',  ( -8.315941417683177406, -20.26807450282663225, 5.303608408759377113 ) ) ;
#18592=CARTESIAN_POINT ( 'NONE',  ( 13.12270769621861355, 4.884238659038159902, 5.513847264053151065 ) ) ;
#18593=CARTESIAN_POINT ( 'NONE',  ( -13.06655316810189227, 2.048434989138931961, 5.965524842914772030 ) ) ;
#18599=CARTESIAN_POINT ( 'NONE',  ( 1.126276606324276619, -9.864917468222230923, 2.372643865078341019 ) ) ;
#18604=CARTESIAN_POINT ( 'NONE',  ( -2.557403344953185442, -14.91030650174552896, 3.668400560659690779 ) ) ;
#18610=CARTESIAN_POINT ( 'NONE',  ( 7.090308582316795061, -21.01515356694490322, 0.9790045612916562501 ) ) ;
#18611=CARTESIAN_POINT ( 'NONE',  ( -13.12529380813666435, 5.014837310896125722, 5.033295791462342628 ) ) ;
#18612=CARTESIAN_POINT ( 'NONE',  ( -9.253441417683177406, -21.94931252712233061, 1.749999999999998446 ) ) ;
#18614=VERTEX_POINT ( 'NONE', #19419 ) ;
#18615=CARTESIAN_POINT ( 'NONE',  ( 10.18405858231679417, -20.79840458871652942, 2.226721677130544030 ) ) ;
#18616=DIRECTION ( 'NONE',  ( -0.000000000000000000, -0.000000000000000000, -1.000000000000000000 ) ) ;
#18617=CARTESIAN_POINT ( 'NONE',  ( -13.40432071140796744, -19.51930407389869515, 6.223619713037471968 ) ) ;
#18618=CARTESIAN_POINT ( 'NONE',  ( 10.74655858231679417, -21.94931252712234482, 5.250000000000000888 ) ) ;
#18624=CARTESIAN_POINT ( 'NONE',  ( 13.37499999999998401, -20.99999999999999645, 3.666666666666654084 ) ) ;
#18630=CARTESIAN_POINT ( 'NONE',  ( -10.18405858231679417, -20.79840458871652942, 2.226721677130544030 ) ) ;
#18631=CARTESIAN_POINT ( 'NONE',  ( 13.87470602645761986, 4.985154336109792972, 4.791666666666685614 ) ) ;
#18633=CARTESIAN_POINT ( 'NONE',  ( 3.475298211275419380, -9.785109117490691233, 1.987377451789144933 ) ) ;
#18636=CARTESIAN_POINT ( 'NONE',  ( -13.37939227869017600, -19.27818992614120575, 4.741950614318236390 ) ) ;
#18638=CARTESIAN_POINT ( 'NONE',  ( -13.40957725085194241, -19.25384883197511243, 6.242932005802575901 ) ) ;
#18640=CARTESIAN_POINT ( 'NONE',  ( 11.77780858231679417, -20.27099543870833642, 2.724438792969431589 ) ) ;
#18641=CARTESIAN_POINT ( 'NONE',  ( 10.47219141768317741, -22.97900456129165292, 3.035098964749240125 ) ) ;
#18642=CARTESIAN_POINT ( 'NONE',  ( -6.152808582316793284, -21.22443879296942626, 5.229004561291659137 ) ) ;
#18644=CARTESIAN_POINT ( 'NONE',  ( 13.37499999999998224, -19.49999999999998934, 4.291666666666699825 ) ) ;
#18651=CARTESIAN_POINT ( 'NONE',  ( -13.09892531043291086, 3.683228176858501790, 6.000681092915118420 ) ) ;
#18652=FACE_OUTER_BOUND ( 'NONE', #9198, .T. ) ;
#18653=CARTESIAN_POINT ( 'NONE',  ( -13.83065313257865370, 2.760483195222930952, 5.966304699623404595 ) ) ;
#18660=CARTESIAN_POINT ( 'NONE',  ( -11.59030858231679595, -21.01515356694490322, 0.9790045612916562501 ) ) ;
#18661=CARTESIAN_POINT ( 'NONE',  ( -1.720709671993384093, -9.114925383610804843, 1.622645897908254753 ) ) ;
#18663=CARTESIAN_POINT ( 'NONE',  ( -13.37597619100657198, -20.20070235416671167, 4.815535977982682070 ) ) ;
#18665=CARTESIAN_POINT ( 'NONE',  ( 10.94094141768317741, -20.19639159124061933, 1.768074502826635586 ) ) ;
#18666=CARTESIAN_POINT ( 'NONE',  ( -4.190941417683176518, -23.27327832286946219, 4.701595411283453707 ) ) ;
#18668=CARTESIAN_POINT ( 'NONE',  ( 13.87215786865436762, 4.856472367046606564, 5.506273593909547515 ) ) ;
#18678=CARTESIAN_POINT ( 'NONE',  ( 2.567175533087980188, -9.771398394011347577, 2.541241281345096859 ) ) ;
#18685=CARTESIAN_POINT ( 'NONE',  ( 3.451003380014874722, -9.682417022083358304, 1.961004070207825523 ) ) ;
#18687=CARTESIAN_POINT ( 'NONE',  ( 13.12529397353891270, 5.014845663890295846, 3.333333333333220239 ) ) ;
#18693=CARTESIAN_POINT ( 'NONE',  ( 5.597191417683177406, -22.46490103525075810, 4.479004561291653808 ) ) ;
#18694=CARTESIAN_POINT ( 'NONE',  ( -13.10192273101908000, 3.834597916462216816, 6.003936301248457674 ) ) ;
#18695=CARTESIAN_POINT ( 'NONE',  ( -10.93405858231679595, -22.67126532539354855, 4.242948236979545484 ) ) ;
#18696=CARTESIAN_POINT ( 'NONE',  ( -4.687312169500634340, -21.32903648725300272, 5.908812401261035241 ) ) ;
#18699=CARTESIAN_POINT ( 'NONE',  ( 12.63118877378512828, -19.18746692385052555, 4.758813856674282583 ) ) ;
#18700=CARTESIAN_POINT ( 'NONE',  ( -13.12526104302547836, 5.013182672784613381, 5.066812735559260261 ) ) ;
#18705=CARTESIAN_POINT ( 'NONE',  ( 2.567175533087980188, -9.771398394011347577, 2.541241281345096859 ) ) ;
#18712=CARTESIAN_POINT ( 'NONE',  ( -1.337453470010121714, -9.864917468222230923, 1.622643865078341907 ) ) ;
#18717=CARTESIAN_POINT ( 'NONE',  ( 5.128441417683177406, -19.49999999999998934, 3.550687472877664952 ) ) ;
#18719=CARTESIAN_POINT ( 'NONE',  ( -7.940941417683176518, -20.72672167713052715, 2.298404588716546293 ) ) ;
#18721=CARTESIAN_POINT ( 'NONE',  ( 8.965308582316794173, -20.22900456129164937, 4.174186261275266929 ) ) ;
#18723=CARTESIAN_POINT ( 'NONE',  ( -13.37499999999998224, -21.00000000000006395, 4.416666666666682062 ) ) ;
#18726=CARTESIAN_POINT ( 'NONE',  ( 12.90280858231679773, -22.77556120703056308, 1.770995438708339975 ) ) ;
#18730=CARTESIAN_POINT ( 'NONE',  ( 13.40995420747273670, -19.23481252262645924, 6.243328185864100988 ) ) ;
#18735=ORIENTED_EDGE ( 'NONE', *, *, #16817, .T. ) ;
#18736=CARTESIAN_POINT ( 'NONE',  ( -10.37155858231679417, -20.24999999999999289, 3.449312527122348371 ) ) ;
#18739=CARTESIAN_POINT ( 'NONE',  ( 3.502569552650398155, -9.961070227720959736, 2.032567780072621400 ) ) ;
#18745=CARTESIAN_POINT ( 'NONE',  ( -13.09206359972826661, 4.086711786274932479, 5.245812454509717782 ) ) ;
#18746=CARTESIAN_POINT ( 'NONE',  ( 10.46530858231679417, -20.22900456129164937, 4.174186261275266929 ) ) ;
#18747=CARTESIAN_POINT ( 'NONE',  ( -13.37499999999998224, -20.99999999999998934, 4.166666666666637653 ) ) ;
#18749=CARTESIAN_POINT ( 'NONE',  ( 11.68405858231679417, -20.79840458871652942, 2.226721677130544030 ) ) ;
#18750=CARTESIAN_POINT ( 'NONE',  ( 3.974842109207561425, -21.82955800590261575, 5.256404853634145447 ) ) ;
#18751=CARTESIAN_POINT ( 'NONE',  ( -11.03469141768317918, -20.22900456129164581, 2.825813738724748170 ) ) ;
#18753=CARTESIAN_POINT ( 'NONE',  ( 13.39169183355864590, -18.65706240528901105, 4.755687463382285429 ) ) ;
#18762=CARTESIAN_POINT ( 'NONE',  ( -12.83635126708105823, -9.576761012430582198, 5.715524842913705328 ) ) ;
#18763=CARTESIAN_POINT ( 'NONE',  ( -2.513306525444908512, -9.622685169956881168, 2.503048754562789746 ) ) ;
#18764=CARTESIAN_POINT ( 'NONE',  ( -13.87470602645761986, 4.985154336109792972, 4.791666666666685614 ) ) ;
#18770=CARTESIAN_POINT ( 'NONE',  ( -10.65280858231679595, -20.91377862118960351, 5.979004561291660913 ) ) ;
#18772=CARTESIAN_POINT ( 'NONE',  ( 0.000000000000000000, -8.364917468222230923, 1.622643865078341241 ) ) ;
#18774=CARTESIAN_POINT ( 'NONE',  ( -13.37500015856764435, -20.24999199233421265, 4.532157119432948633 ) ) ;
#18776=CARTESIAN_POINT ( 'NONE',  ( 10.47219141768317741, -24.47900456129165292, 2.413778621189595963 ) ) ;
#18777=CARTESIAN_POINT ( 'NONE',  ( -5.597191417683177406, -22.46490103525075810, 4.479004561291653808 ) ) ;
#18779=CARTESIAN_POINT ( 'NONE',  ( 13.37607268932110038, -20.94582918928111681, 4.945564004704174010 ) ) ;
#18793=CARTESIAN_POINT ( 'NONE',  ( 1.798207051321043304, -8.367281747657623114, 1.623251059268568053 ) ) ;
#18795=CARTESIAN_POINT ( 'NONE',  ( 13.10624331898488037, 4.052787608736739600, 6.006964772046813117 ) ) ;
#18800=CARTESIAN_POINT ( 'NONE',  ( 8.315941417683177406, -21.32873467460645145, 4.242948236979555254 ) ) ;
#18801=CARTESIAN_POINT ( 'NONE',  ( -12.65051119073526564, -18.96168486786632457, 5.513701926248478102 ) ) ;
#18802=CARTESIAN_POINT ( 'NONE',  ( -13.18405858231679595, -21.32873467460644079, 2.757051763020455404 ) ) ;
#18804=CARTESIAN_POINT ( 'NONE',  ( -4.753441417683176518, -21.94931252712233061, 0.9999999999999978906 ) ) ;
#18806=CARTESIAN_POINT ( 'NONE',  ( 13.37523871602689596, -19.48794484064217514, 4.577160611493482634 ) ) ;
#18808=ORIENTED_EDGE ( 'NONE', *, *, #9614, .T. ) ;
#18811=CARTESIAN_POINT ( 'NONE',  ( 1.896776615114361908, -10.21987218505477024, 2.463803327293850209 ) ) ;
#18815=CIRCLE ( 'NONE', #2790, 0.3749999999999997224 ) ;
#18818=CARTESIAN_POINT ( 'NONE',  ( -2.627360420079438263, -14.25085146736906339, 2.749039333894452763 ) ) ;
#18823=CARTESIAN_POINT ( 'NONE',  ( 6.628441417683177406, -19.49999999999998934, 3.550687472877664952 ) ) ;
#18825=CARTESIAN_POINT ( 'NONE',  ( -8.878441417683177406, -23.74999999999999645, 3.449312527122335492 ) ) ;
#18827=CARTESIAN_POINT ( 'NONE',  ( 7.371558582316794173, -20.24999999999999289, 3.449312527122348371 ) ) ;
#18829=CARTESIAN_POINT ( 'NONE',  ( -12.62499999999998224, -20.99999999999998934, 4.291666666666699825 ) ) ;
#18834=CARTESIAN_POINT ( 'NONE',  ( 13.83079205777725917, 2.017498917744843023, 6.700359435863729729 ) ) ;
#18837=EDGE_CURVE ( 'NONE', #9910, #13028, #10106, .T. ) ;
#18840=CARTESIAN_POINT ( 'NONE',  ( -13.09030858231679417, -21.32581373872472597, 1.729004561291657582 ) ) ;
#18844=DIRECTION ( 'NONE',  ( 0.1351665943404306014, -0.9596796555888912339, 0.2464649070825229438 ) ) ;
#18845=CARTESIAN_POINT ( 'NONE',  ( 1.652577328807104839, -9.114908150887895744, 1.622641472200749835 ) ) ;
#18846=EDGE_CURVE ( 'NONE', #6462, #19322, #3618, .T. ) ;
#18848=CARTESIAN_POINT ( 'NONE',  ( -13.09533517714100093, 4.251926445620864747, 5.084080158857392284 ) ) ;
#18849=CARTESIAN_POINT ( 'NONE',  ( 9.715308582316794173, -23.77099543870833998, 2.825813738724734847 ) ) ;
#18850=CARTESIAN_POINT ( 'NONE',  ( -13.87372783958217681, 4.185755898898970706, 6.732634959205082481 ) ) ;
#18852=CARTESIAN_POINT ( 'NONE',  ( 7.277808582316794173, -20.27099543870833642, 2.724438792969431589 ) ) ;
#18854=CARTESIAN_POINT ( 'NONE',  ( 4.940941417683177406, -20.72672167713052715, 2.298404588716546293 ) ) ;
#18855=CARTESIAN_POINT ( 'NONE',  ( -7.652808582316795061, -21.22443879296942626, 5.229004561291659137 ) ) ;
#18857=CARTESIAN_POINT ( 'NONE',  ( 13.37514942709654164, -19.49245393162283690, 4.562067678168288509 ) ) ;
#18859=ORIENTED_EDGE ( 'NONE', *, *, #1611, .F. ) ;
#18863=CARTESIAN_POINT ( 'NONE',  ( -13.10252221513633941, 3.864871864382954048, 6.004587342915129966 ) ) ;
#18865=CARTESIAN_POINT ( 'NONE',  ( -1.728780693989796724, -8.364929292255887106, 2.372646901726390478 ) ) ;
#18866=CARTESIAN_POINT ( 'NONE',  ( -13.85163507668220539, 3.820071372449974412, 5.989091157956555556 ) ) ;
#18872=CARTESIAN_POINT ( 'NONE',  ( -4.717959273841178636, -21.72818306014730183, 5.243595146365860771 ) ) ;
#18873=CARTESIAN_POINT ( 'NONE',  ( -1.733187991654075777, -9.867296153774269385, 1.623254759047128237 ) ) ;
#18874=ORIENTED_EDGE ( 'NONE', *, *, #15642, .T. ) ;
#18875=CARTESIAN_POINT ( 'NONE',  ( -13.84042474920106081, 4.003949834653575124, 5.242612001278796008 ) ) ;
#18877=CARTESIAN_POINT ( 'NONE',  ( 6.996558582316795949, -22.05068747287764452, 0.9999999999999978906 ) ) ;
#18878=CARTESIAN_POINT ( 'NONE',  ( -11.77780858231679595, -21.02099543870833998, 3.035098964749253003 ) ) ;
#18880=CARTESIAN_POINT ( 'NONE',  ( 13.87470623115321899, 4.985164673244912414, 4.958488177337359026 ) ) ;
#18888=CARTESIAN_POINT ( 'NONE',  ( -13.87470602645761986, 4.985154336109792972, 4.166666666666758445 ) ) ;
#18890=CARTESIAN_POINT ( 'NONE',  ( 1.548630333695928396, -9.114917468222230923, 2.372643865078341019 ) ) ;
#18894=CARTESIAN_POINT ( 'NONE',  ( 2.567175533087980188, -9.771398394011347577, 2.541241281345096859 ) ) ;
#18896=CARTESIAN_POINT ( 'NONE',  ( 1.948765222931501784, -9.143197003266354983, 1.629906614618163552 ) ) ;
#18904=CARTESIAN_POINT ( 'NONE',  ( 6.909691417683176518, -21.63647391050456648, 4.520995438708348857 ) ) ;
#18905=CARTESIAN_POINT ( 'NONE',  ( -12.62499999999998401, -19.49999999999998934, 3.666666666666654084 ) ) ;
#18906=CARTESIAN_POINT ( 'NONE',  ( -10.18405858231679595, -21.32873467460644079, 2.757051763020455404 ) ) ;
#18907=CARTESIAN_POINT ( 'NONE',  ( -11.22219141768317741, -20.27099543870833998, 4.275561207030583510 ) ) ;
#18909=CARTESIAN_POINT ( 'NONE',  ( 13.08080186171710224, 3.517994016715657146, 5.247095106674282583 ) ) ;
#18914=CARTESIAN_POINT ( 'NONE',  ( 1.837882866761050282, -9.938290523052360825, 2.391487531332776140 ) ) ;
#18916=CARTESIAN_POINT ( 'NONE',  ( 8.503441417683177406, -22.05068747287765873, 5.250000000000000888 ) ) ;
#18918=CARTESIAN_POINT ( 'NONE',  ( -1.407845757905374695, -9.864917468222230923, 1.622643865078341907 ) ) ;
#18923=CARTESIAN_POINT ( 'NONE',  ( 7.753441417683177406, -21.94931252712233061, 0.9999999999999978906 ) ) ;
#18925=CARTESIAN_POINT ( 'NONE',  ( -7.003441417683177406, -22.05068747287765873, 5.250000000000000888 ) ) ;
#18928=CARTESIAN_POINT ( 'NONE',  ( 9.902808582316794173, -22.77556120703056308, 1.770995438708339975 ) ) ;
#18930=CARTESIAN_POINT ( 'NONE',  ( -12.62500000000002132, -21.00000000000274269, 4.083333333315724012 ) ) ;
#18937=ORIENTED_EDGE ( 'NONE', *, *, #1049, .T. ) ;
#18940=CARTESIAN_POINT ( 'NONE',  ( -9.902808582316794173, -22.77556120703056308, 1.770995438708339975 ) ) ;
#18941=CARTESIAN_POINT ( 'NONE',  ( 12.63465172146706728, -19.76258806590802664, 5.372658420469845986 ) ) ;
#18943=CARTESIAN_POINT ( 'NONE',  ( 1.513434189748285696, -9.114917468222230923, 1.622643865078341463 ) ) ;
#18946=CARTESIAN_POINT ( 'NONE',  ( -13.37593719518949698, -19.45267164293252193, 4.647380496992003174 ) ) ;
#18947=CARTESIAN_POINT ( 'NONE',  ( 6.340308582316793284, -22.67418626127525982, 5.270995438708342640 ) ) ;
#18948=CARTESIAN_POINT ( 'NONE',  ( -12.62499999999998224, -21.00000000000006395, 4.416666666666682062 ) ) ;
#18951=CARTESIAN_POINT ( 'NONE',  ( 6.527808582316794173, -23.72900456129165647, 4.275561207030568411 ) ) ;
#18952=CARTESIAN_POINT ( 'NONE',  ( 7.753441417683177406, -21.94931252712233061, 2.499999999999999112 ) ) ;
#18953=CARTESIAN_POINT ( 'NONE',  ( -10.84719141768317741, -21.22443879296941915, 1.770995438708345748 ) ) ;
#18956=CARTESIAN_POINT ( 'NONE',  ( 13.37593719518949698, -19.45267164293252193, 4.647380496992003174 ) ) ;
#18959=CARTESIAN_POINT ( 'NONE',  ( -0.2815691515810352930, -9.114917468222230923, 1.622643865078524206 ) ) ;
#18965=CARTESIAN_POINT ( 'NONE',  ( -3.321934647848983957, -9.834888441627915867, 2.750161776669472591 ) ) ;
#18966=CARTESIAN_POINT ( 'NONE',  ( -13.85343352903393388, 3.910893216212274925, 5.991044282956552891 ) ) ;
#18967=CARTESIAN_POINT ( 'NONE',  ( 2.762374231067749708, -9.968169115173667549, 1.841775933429679268 ) ) ;
#18969=CARTESIAN_POINT ( 'NONE',  ( 11.96530858231679417, -20.22900456129164937, 4.174186261275266929 ) ) ;
#18972=CARTESIAN_POINT ( 'NONE',  ( 13.15498501280115917, 5.764243146453090105, 5.045733045595949484 ) ) ;
#18974=CARTESIAN_POINT ( 'NONE',  ( -5.777808582316795949, -19.52099543870833642, 2.413778621189609286 ) ) ;
#18975=CARTESIAN_POINT ( 'NONE',  ( -1.732184490400474175, -9.869581059509965115, 2.373841568485653308 ) ) ;
#18977=CARTESIAN_POINT ( 'NONE',  ( -13.38238173943565990, -19.87722215849730034, 5.285856107751903288 ) ) ;
#18980=CARTESIAN_POINT ( 'NONE',  ( 5.222191417683177406, -19.52099543870834353, 4.586221378810406257 ) ) ;
#18981=CARTESIAN_POINT ( 'NONE',  ( -4.284691417683177406, -23.02099543870834353, 3.863526089495429972 ) ) ;
#18983=CARTESIAN_POINT ( 'NONE',  ( 13.39995901559228031, -19.73956971259024229, 6.178279423016713956 ) ) ;
#18989=CARTESIAN_POINT ( 'NONE',  ( 1.619022621591187150, -9.114917468222230923, 2.372643865078341019 ) ) ;
#18994=( BOUNDED_SURFACE ( )  B_SPLINE_SURFACE ( 3, 2, ( 
 ( #8790, #18413, #12124, #3866, #12325, #15158, #834, #20293, #4177, #5855, #10352, #4075, #10661, #18300, #7319, #18516, #19981, #16929, #12225, #5642, #13680, #2601, #15256, #9095, #15362, #1150, #5950, #2289, #933, #16726, #2399, #7217, #1045, #7429, #18615, #6064, #7737, #18928, #3026, #7834, #6478, #1250, #1354, #7625, #14295, #12629, #4689, #18721, #1455, #10875, #12432, #6369, #17450, #15567, #4585, #13992, #20603, #9597, #19142, #20706, #19033, #14408, #6255, #11176, #18827, #4390, #1657, #12739, #9502, #2918, #10771, #15875, #14196, #17549, #9403, #20509, #15670, #9192, #10973, #17343, #14100, #17140, #2819, #11079, #3129, #1550, #3226, #7928, #20401, #6163, #15975, #4489, #4795, #17239, #8042 ),
 ( #92, #9295, #12530, #15775, #14722, #3535, #4024, #16669, #11963, #19449, #18361, #7170, #9911, #19935, #11271, #5204, #17766, #14513, #288, #19242, #6573, #785, #190, #5106, #1763, #17962, #9812, #11582, #13533, #11486, #6679, #12937, #16198, #16292, #8245, #19342, #5593, #13048, #4997, #8150, #400, #1964, #10408, #16780, #17865, #3434, #11376, #8346, #1863, #6782, #13152, #19549, #3917, #2448, #17652, #14611, #10298, #2346, #3325, #8841, #8739, #15108, #15208, #884, #12838, #4891, #9707, #16094, #18877, #15725, #2657, #2768, #7577, #12485, #8936, #9047, #7377, #12383, #17288, #1201, #15615, #4443, #15416, #1100, #2970, #7479, #13740, #20457, #13840, #20143, #16879, #15516, #17091, #1298, #7679 ),
 ( #12273, #2549, #9147, #13940, #20342, #20243, #6114, #12074, #15307, #5803, #5901, #18465, #4538, #12174, #2868, #4334, #18562, #6006, #18665, #10718, #4227, #10923, #7269, #18776, #10826, #17191, #9346, #988, #9245, #10607, #14048, #10508, #16980, #13630, #20038, #5702, #4127, #14354, #14463, #6529, #14565, #12789, #1406, #19087, #11434, #12684, #6426, #15925, #9653, #7788, #1602, #7981, #6627, #1813, #15826, #19192, #3178, #19398, #14151, #11326, #20653, #9552, #12579, #8199, #5057, #238, #17398, #12996, #17498, #17713, #11028, #40, #143, #20558, #4845, #6209, #3485, #11226, #1715, #18980, #17602, #12890, #19294, #1503, #9763, #3275, #16039, #17818, #4947, #9861, #8100, #4635, #16148, #3384, #3080 ),
 ( #9454, #7885, #14244, #6310, #4742, #11129, #2120, #5155, #650, #13199, #14972, #16639, #14873, #10073, #16343, #19598, #19697, #5251, #8707, #11534, #5360, #14669, #18130, #8502, #16245, #19912, #17913, #349, #3996, #13101, #6929, #18229, #451, #11628, #2218, #6736, #1914, #5466, #9961, #3580, #761, #18018, #6830, #3689, #11738, #8295, #19503, #16447, #549, #11937, #16542, #11838, #2018, #13296, #2319, #8408, #3795, #10172, #8601, #7038, #3891, #13407, #19812, #10271, #15079, #7146, #13510, #5566, #18333, #14775, #10585, #10485, #18440, #16855, #12249, #2844, #18540, #4102, #20117, #16953, #15390, #20218, #18854, #13606, #13711, #20010, #5981, #4307, #17063, #10381, #13816, #2522, #8914, #18750, #9123 ),
 ( #10692, #15590, #12045, #5780, #15282, #15491, #5674, #960, #4416, #7553, #20433, #16754, #2632, #2743, #1175, #9220, #1075, #2425, #7349, #6092, #12149, #7454, #4203, #18641, #8816, #9019, #5879, #1274, #10800, #13916, #20318, #12356, #7654, #15184, #17169, #14024, #12460, #861, #7244, #1787, #11298, #20533, #9735, #20629, #119, #14128, #11106, #4823, #10899, #14326, #3251, #17577, #18952, #12866, #6399, #15899, #16120, #8072, #3356, #17477, #8174, #19268, #1578, #17685, #2941, #9623, #9430, #6186, #12656, #17262, #4607, #4920, #12554, #3155, #11001, #16009, #1479, #1686, #14542, #9527, #19059, #17370, #7859, #7953, #6282, #3056, #214, #4717, #15802, #14221, #12766, #11, #6600, #12967, #19169 ),
 ( #11204, #14437, #6504, #4515, #9323, #15698, #1382, #7763, #17891, #17991, #3458, #18206, #19478, #14946, #16420, #5131, #5336, #10046, #3661, #9938, #10246, #7122, #14750, #14848, #19671, #3868, #322, #428, #11510, #3770, #1890, #16317, #7015, #16520, #8685, #19371, #11606, #11709, #10149, #11813, #2097, #5026, #1993, #15056, #8378, #8480, #13175, #6903, #11406, #19574, #5228, #16613, #19784, #13076, #524, #6807, #2293, #17792, #8577, #3558, #13271, #9836, #5444, #738, #16223, #14640, #8270, #18106, #626, #6707, #2194, #13382, #11913, #18520, #5543, #15570, #16932, #12329, #13794, #1254, #2497, #5954, #2403, #2604, #18304, #15366, #20094, #13486, #17146, #8794, #3969, #19887, #10356, #4180, #15471 ),
 ( #16730, #15161, #2718, #7220, #837, #18726, #8893, #18416, #937, #8994, #13583, #19984, #4078, #10466, #9196, #20198, #9099, #5647, #7323, #20296, #12020, #1050, #7432, #15259, #5859, #1153, #13685, #12228, #18618, #5757, #4393, #4280, #10776, #16833, #12128, #10563, #10666, #17040, #7530, #13896, #2823, #15780, #15675, #17349, #7838, #12633, #17454, #16098, #10879, #10977, #17242, #3230, #1555, #14299, #7628, #11083, #20513, #1359, #15980, #6375, #4494, #14200, #2922, #97, #13998, #6166, #4799, #20609, #6260, #9300, #7742, #7933, #1661, #11180, #3031, #1459, #17656, #9506, #19246, #8049, #9601, #20711, #3330, #15878, #6482, #14105, #20406, #11276, #14412, #19145, #12534, #6068, #17555, #3132, #12842 ) ),
 .UNSPECIFIED., .T., .F., .F. ) 
 B_SPLINE_SURFACE_WITH_KNOTS ( ( 4, 3, 4 ),
 ( 3, 2, 2, 2, 2, 2, 2, 2, 2, 2, 2, 2, 2, 2, 2, 2, 2, 2, 2, 2, 2, 2, 2, 2, 2, 2, 2, 2, 2, 2, 2, 2, 2, 2, 2, 2, 2, 2, 2, 2, 2, 2, 2, 2, 2, 2, 2, 3 ),
 ( 0.000000000000000000, 0.5000000000000000000, 1.000000000000000000 ),
 ( 0.000000000000000000, 0.02083333333333333218, 0.04166666666666666435, 0.06250000000000000000, 0.08333333333333332871, 0.1041666666666666713, 0.1250000000000000000, 0.1458333333333333426, 0.1666666666666666574, 0.1875000000000000000, 0.2083333333333333426, 0.2291666666666666574, 0.2500000000000000000, 0.2708333333333333148, 0.2916666666666666852, 0.3125000000000000000, 0.3333333333333333148, 0.3541666666666666852, 0.3750000000000000000, 0.3958333333333333148, 0.4166666666666666852, 0.4375000000000000000, 0.4583333333333333148, 0.4791666666666666852, 0.5000000000000000000, 0.5208333333333333703, 0.5416666666666666297, 0.5625000000000000000, 0.5833333333333333703, 0.6041666666666666297, 0.6250000000000000000, 0.6458333333333333703, 0.6666666666666666297, 0.6875000000000000000, 0.7083333333333333703, 0.7291666666666666297, 0.7500000000000000000, 0.7708333333333333703, 0.7916666666666666297, 0.8125000000000000000, 0.8333333333333333703, 0.8541666666666666297, 0.8750000000000000000, 0.8958333333333333703, 0.9166666666666666297, 0.9375000000000000000, 0.9583333333333333703, 0.9650437087885355147 ),
 .UNSPECIFIED. ) 
 GEOMETRIC_REPRESENTATION_ITEM ( )  RATIONAL_B_SPLINE_SURFACE ( (
 ( 1.000000000000000000, 0.9238795325112867385, 1.000000000000000000, 0.9238795325112867385, 1.000000000000000000, 0.9238795325112867385, 1.000000000000000000, 0.9238795325112867385, 1.000000000000000000, 0.9238795325112867385, 1.000000000000000000, 0.9238795325112867385, 1.000000000000000000, 0.9238795325112867385, 1.000000000000000000, 0.9238795325112867385, 1.000000000000000000, 0.9238795325112867385, 1.000000000000000000, 0.9238795325112867385, 1.000000000000000000, 0.9238795325112867385, 1.000000000000000000, 0.9238795325112867385, 1.000000000000000000, 0.9238795325112867385, 1.000000000000000000, 0.9238795325112867385, 1.000000000000000000, 0.9238795325112867385, 1.000000000000000000, 0.9238795325112867385, 1.000000000000000000, 0.9238795325112867385, 1.000000000000000000, 0.9238795325112867385, 1.000000000000000000, 0.9238795325112867385, 1.000000000000000000, 0.9238795325112867385, 1.000000000000000000, 0.9238795325112867385, 1.000000000000000000, 0.9238795325112867385, 1.000000000000000000, 0.9238795325112867385, 1.000000000000000000, 0.9238795325112867385, 1.000000000000000000, 0.9238795325112867385, 1.000000000000000000, 0.9238795325112867385, 1.000000000000000000, 0.9238795325112867385, 1.000000000000000000, 0.9238795325112867385, 1.000000000000000000, 0.9238795325112867385, 1.000000000000000000, 0.9238795325112867385, 1.000000000000000000, 0.9238795325112867385, 1.000000000000000000, 0.9238795325112867385, 1.000000000000000000, 0.9238795325112867385, 1.000000000000000000, 0.9238795325112867385, 1.000000000000000000, 0.9238795325112867385, 1.000000000000000000, 0.9238795325112867385, 1.000000000000000000, 0.9238795325112867385, 1.000000000000000000, 0.9238795325112867385, 1.000000000000000000, 0.9238795325112867385, 1.000000000000000000, 0.9238795325112867385, 1.000000000000000000, 0.9238795325112867385, 1.000000000000000000, 0.9238795325112867385, 1.000000000000000000, 0.9238795325112867385, 1.000000000000000000, 0.9238795325112867385, 1.000000000000000000, 0.9238795325112867385, 1.000000000000000000, 0.9238795325112867385, 1.000000000000000000, 0.9754817479996107377, 0.9667580569362973497),
 ( 0.3333333333333333703, 0.3079598441704289313, 0.3333333333333333703, 0.3079598441704289313, 0.3333333333333333703, 0.3079598441704289313, 0.3333333333333333703, 0.3079598441704289313, 0.3333333333333333703, 0.3079598441704289313, 0.3333333333333333703, 0.3079598441704289313, 0.3333333333333333703, 0.3079598441704289313, 0.3333333333333333703, 0.3079598441704289313, 0.3333333333333333703, 0.3079598441704289313, 0.3333333333333333703, 0.3079598441704289313, 0.3333333333333333703, 0.3079598441704289313, 0.3333333333333333703, 0.3079598441704289313, 0.3333333333333333703, 0.3079598441704289313, 0.3333333333333333703, 0.3079598441704289313, 0.3333333333333333703, 0.3079598441704289313, 0.3333333333333333703, 0.3079598441704289313, 0.3333333333333333703, 0.3079598441704289313, 0.3333333333333333703, 0.3079598441704289313, 0.3333333333333333703, 0.3079598441704289313, 0.3333333333333333703, 0.3079598441704289313, 0.3333333333333333703, 0.3079598441704289313, 0.3333333333333333703, 0.3079598441704289313, 0.3333333333333333703, 0.3079598441704289313, 0.3333333333333333703, 0.3079598441704289313, 0.3333333333333333703, 0.3079598441704289313, 0.3333333333333333703, 0.3079598441704289313, 0.3333333333333333703, 0.3079598441704289313, 0.3333333333333333703, 0.3079598441704289313, 0.3333333333333333703, 0.3079598441704289313, 0.3333333333333333703, 0.3079598441704289313, 0.3333333333333333703, 0.3079598441704289313, 0.3333333333333333703, 0.3079598441704289313, 0.3333333333333333703, 0.3079598441704289313, 0.3333333333333333703, 0.3079598441704289313, 0.3333333333333333703, 0.3079598441704289313, 0.3333333333333333703, 0.3079598441704289313, 0.3333333333333333703, 0.3079598441704289313, 0.3333333333333333703, 0.3079598441704289313, 0.3333333333333333703, 0.3079598441704289313, 0.3333333333333333703, 0.3079598441704289313, 0.3333333333333333703, 0.3079598441704289313, 0.3333333333333333703, 0.3079598441704289313, 0.3333333333333333703, 0.3079598441704289313, 0.3333333333333333703, 0.3079598441704289313, 0.3333333333333333703, 0.3079598441704289313, 0.3333333333333333703, 0.3079598441704289313, 0.3333333333333333703, 0.3251605826665369681, 0.3222526856454325239),
 ( 0.3333333333333333703, 0.3079598441704289313, 0.3333333333333333703, 0.3079598441704289313, 0.3333333333333333703, 0.3079598441704289313, 0.3333333333333333703, 0.3079598441704289313, 0.3333333333333333703, 0.3079598441704289313, 0.3333333333333333703, 0.3079598441704289313, 0.3333333333333333703, 0.3079598441704289313, 0.3333333333333333703, 0.3079598441704289313, 0.3333333333333333703, 0.3079598441704289313, 0.3333333333333333703, 0.3079598441704289313, 0.3333333333333333703, 0.3079598441704289313, 0.3333333333333333703, 0.3079598441704289313, 0.3333333333333333703, 0.3079598441704289313, 0.3333333333333333703, 0.3079598441704289313, 0.3333333333333333703, 0.3079598441704289313, 0.3333333333333333703, 0.3079598441704289313, 0.3333333333333333703, 0.3079598441704289313, 0.3333333333333333703, 0.3079598441704289313, 0.3333333333333333703, 0.3079598441704289313, 0.3333333333333333703, 0.3079598441704289313, 0.3333333333333333703, 0.3079598441704289313, 0.3333333333333333703, 0.3079598441704289313, 0.3333333333333333703, 0.3079598441704289313, 0.3333333333333333703, 0.3079598441704289313, 0.3333333333333333703, 0.3079598441704289313, 0.3333333333333333703, 0.3079598441704289313, 0.3333333333333333703, 0.3079598441704289313, 0.3333333333333333703, 0.3079598441704289313, 0.3333333333333333703, 0.3079598441704289313, 0.3333333333333333703, 0.3079598441704289313, 0.3333333333333333703, 0.3079598441704289313, 0.3333333333333333703, 0.3079598441704289313, 0.3333333333333333703, 0.3079598441704289313, 0.3333333333333333703, 0.3079598441704289313, 0.3333333333333333703, 0.3079598441704289313, 0.3333333333333333703, 0.3079598441704289313, 0.3333333333333333703, 0.3079598441704289313, 0.3333333333333333703, 0.3079598441704289313, 0.3333333333333333703, 0.3079598441704289313, 0.3333333333333333703, 0.3079598441704289313, 0.3333333333333333703, 0.3079598441704289313, 0.3333333333333333703, 0.3079598441704289313, 0.3333333333333333703, 0.3079598441704289313, 0.3333333333333333703, 0.3079598441704289313, 0.3333333333333333703, 0.3079598441704289313, 0.3333333333333333703, 0.3079598441704289313, 0.3333333333333333703, 0.3251605826665369681, 0.3222526856454325239),
 ( 1.000000000000000000, 0.9238795325112867385, 1.000000000000000000, 0.9238795325112867385, 1.000000000000000000, 0.9238795325112867385, 1.000000000000000000, 0.9238795325112867385, 1.000000000000000000, 0.9238795325112867385, 1.000000000000000000, 0.9238795325112867385, 1.000000000000000000, 0.9238795325112867385, 1.000000000000000000, 0.9238795325112867385, 1.000000000000000000, 0.9238795325112867385, 1.000000000000000000, 0.9238795325112867385, 1.000000000000000000, 0.9238795325112867385, 1.000000000000000000, 0.9238795325112867385, 1.000000000000000000, 0.9238795325112867385, 1.000000000000000000, 0.9238795325112867385, 1.000000000000000000, 0.9238795325112867385, 1.000000000000000000, 0.9238795325112867385, 1.000000000000000000, 0.9238795325112867385, 1.000000000000000000, 0.9238795325112867385, 1.000000000000000000, 0.9238795325112867385, 1.000000000000000000, 0.9238795325112867385, 1.000000000000000000, 0.9238795325112867385, 1.000000000000000000, 0.9238795325112867385, 1.000000000000000000, 0.9238795325112867385, 1.000000000000000000, 0.9238795325112867385, 1.000000000000000000, 0.9238795325112867385, 1.000000000000000000, 0.9238795325112867385, 1.000000000000000000, 0.9238795325112867385, 1.000000000000000000, 0.9238795325112867385, 1.000000000000000000, 0.9238795325112867385, 1.000000000000000000, 0.9238795325112867385, 1.000000000000000000, 0.9238795325112867385, 1.000000000000000000, 0.9238795325112867385, 1.000000000000000000, 0.9238795325112867385, 1.000000000000000000, 0.9238795325112867385, 1.000000000000000000, 0.9238795325112867385, 1.000000000000000000, 0.9238795325112867385, 1.000000000000000000, 0.9238795325112867385, 1.000000000000000000, 0.9238795325112867385, 1.000000000000000000, 0.9238795325112867385, 1.000000000000000000, 0.9238795325112867385, 1.000000000000000000, 0.9238795325112867385, 1.000000000000000000, 0.9238795325112867385, 1.000000000000000000, 0.9238795325112867385, 1.000000000000000000, 0.9238795325112867385, 1.000000000000000000, 0.9238795325112867385, 1.000000000000000000, 0.9238795325112867385, 1.000000000000000000, 0.9754817479996107377, 0.9667580569362973497),
 ( 0.3333333333333333703, 0.3079598441704289313, 0.3333333333333333703, 0.3079598441704289313, 0.3333333333333333703, 0.3079598441704289313, 0.3333333333333333703, 0.3079598441704289313, 0.3333333333333333703, 0.3079598441704289313, 0.3333333333333333703, 0.3079598441704289313, 0.3333333333333333703, 0.3079598441704289313, 0.3333333333333333703, 0.3079598441704289313, 0.3333333333333333703, 0.3079598441704289313, 0.3333333333333333703, 0.3079598441704289313, 0.3333333333333333703, 0.3079598441704289313, 0.3333333333333333703, 0.3079598441704289313, 0.3333333333333333703, 0.3079598441704289313, 0.3333333333333333703, 0.3079598441704289313, 0.3333333333333333703, 0.3079598441704289313, 0.3333333333333333703, 0.3079598441704289313, 0.3333333333333333703, 0.3079598441704289313, 0.3333333333333333703, 0.3079598441704289313, 0.3333333333333333703, 0.3079598441704289313, 0.3333333333333333703, 0.3079598441704289313, 0.3333333333333333703, 0.3079598441704289313, 0.3333333333333333703, 0.3079598441704289313, 0.3333333333333333703, 0.3079598441704289313, 0.3333333333333333703, 0.3079598441704289313, 0.3333333333333333703, 0.3079598441704289313, 0.3333333333333333703, 0.3079598441704289313, 0.3333333333333333703, 0.3079598441704289313, 0.3333333333333333703, 0.3079598441704289313, 0.3333333333333333703, 0.3079598441704289313, 0.3333333333333333703, 0.3079598441704289313, 0.3333333333333333703, 0.3079598441704289313, 0.3333333333333333703, 0.3079598441704289313, 0.3333333333333333703, 0.3079598441704289313, 0.3333333333333333703, 0.3079598441704289313, 0.3333333333333333703, 0.3079598441704289313, 0.3333333333333333703, 0.3079598441704289313, 0.3333333333333333703, 0.3079598441704289313, 0.3333333333333333703, 0.3079598441704289313, 0.3333333333333333703, 0.3079598441704289313, 0.3333333333333333703, 0.3079598441704289313, 0.3333333333333333703, 0.3079598441704289313, 0.3333333333333333703, 0.3079598441704289313, 0.3333333333333333703, 0.3079598441704289313, 0.3333333333333333703, 0.3079598441704289313, 0.3333333333333333703, 0.3079598441704289313, 0.3333333333333333703, 0.3079598441704289313, 0.3333333333333333703, 0.3251605826665369681, 0.3222526856454325239),
 ( 0.3333333333333333703, 0.3079598441704289313, 0.3333333333333333703, 0.3079598441704289313, 0.3333333333333333703, 0.3079598441704289313, 0.3333333333333333703, 0.3079598441704289313, 0.3333333333333333703, 0.3079598441704289313, 0.3333333333333333703, 0.3079598441704289313, 0.3333333333333333703, 0.3079598441704289313, 0.3333333333333333703, 0.3079598441704289313, 0.3333333333333333703, 0.3079598441704289313, 0.3333333333333333703, 0.3079598441704289313, 0.3333333333333333703, 0.3079598441704289313, 0.3333333333333333703, 0.3079598441704289313, 0.3333333333333333703, 0.3079598441704289313, 0.3333333333333333703, 0.3079598441704289313, 0.3333333333333333703, 0.3079598441704289313, 0.3333333333333333703, 0.3079598441704289313, 0.3333333333333333703, 0.3079598441704289313, 0.3333333333333333703, 0.3079598441704289313, 0.3333333333333333703, 0.3079598441704289313, 0.3333333333333333703, 0.3079598441704289313, 0.3333333333333333703, 0.3079598441704289313, 0.3333333333333333703, 0.3079598441704289313, 0.3333333333333333703, 0.3079598441704289313, 0.3333333333333333703, 0.3079598441704289313, 0.3333333333333333703, 0.3079598441704289313, 0.3333333333333333703, 0.3079598441704289313, 0.3333333333333333703, 0.3079598441704289313, 0.3333333333333333703, 0.3079598441704289313, 0.3333333333333333703, 0.3079598441704289313, 0.3333333333333333703, 0.3079598441704289313, 0.3333333333333333703, 0.3079598441704289313, 0.3333333333333333703, 0.3079598441704289313, 0.3333333333333333703, 0.3079598441704289313, 0.3333333333333333703, 0.3079598441704289313, 0.3333333333333333703, 0.3079598441704289313, 0.3333333333333333703, 0.3079598441704289313, 0.3333333333333333703, 0.3079598441704289313, 0.3333333333333333703, 0.3079598441704289313, 0.3333333333333333703, 0.3079598441704289313, 0.3333333333333333703, 0.3079598441704289313, 0.3333333333333333703, 0.3079598441704289313, 0.3333333333333333703, 0.3079598441704289313, 0.3333333333333333703, 0.3079598441704289313, 0.3333333333333333703, 0.3079598441704289313, 0.3333333333333333703, 0.3079598441704289313, 0.3333333333333333703, 0.3079598441704289313, 0.3333333333333333703, 0.3251605826665369681, 0.3222526856454325239),
 ( 1.000000000000000000, 0.9238795325112867385, 1.000000000000000000, 0.9238795325112867385, 1.000000000000000000, 0.9238795325112867385, 1.000000000000000000, 0.9238795325112867385, 1.000000000000000000, 0.9238795325112867385, 1.000000000000000000, 0.9238795325112867385, 1.000000000000000000, 0.9238795325112867385, 1.000000000000000000, 0.9238795325112867385, 1.000000000000000000, 0.9238795325112867385, 1.000000000000000000, 0.9238795325112867385, 1.000000000000000000, 0.9238795325112867385, 1.000000000000000000, 0.9238795325112867385, 1.000000000000000000, 0.9238795325112867385, 1.000000000000000000, 0.9238795325112867385, 1.000000000000000000, 0.9238795325112867385, 1.000000000000000000, 0.9238795325112867385, 1.000000000000000000, 0.9238795325112867385, 1.000000000000000000, 0.9238795325112867385, 1.000000000000000000, 0.9238795325112867385, 1.000000000000000000, 0.9238795325112867385, 1.000000000000000000, 0.9238795325112867385, 1.000000000000000000, 0.9238795325112867385, 1.000000000000000000, 0.9238795325112867385, 1.000000000000000000, 0.9238795325112867385, 1.000000000000000000, 0.9238795325112867385, 1.000000000000000000, 0.9238795325112867385, 1.000000000000000000, 0.9238795325112867385, 1.000000000000000000, 0.9238795325112867385, 1.000000000000000000, 0.9238795325112867385, 1.000000000000000000, 0.9238795325112867385, 1.000000000000000000, 0.9238795325112867385, 1.000000000000000000, 0.9238795325112867385, 1.000000000000000000, 0.9238795325112867385, 1.000000000000000000, 0.9238795325112867385, 1.000000000000000000, 0.9238795325112867385, 1.000000000000000000, 0.9238795325112867385, 1.000000000000000000, 0.9238795325112867385, 1.000000000000000000, 0.9238795325112867385, 1.000000000000000000, 0.9238795325112867385, 1.000000000000000000, 0.9238795325112867385, 1.000000000000000000, 0.9238795325112867385, 1.000000000000000000, 0.9238795325112867385, 1.000000000000000000, 0.9238795325112867385, 1.000000000000000000, 0.9238795325112867385, 1.000000000000000000, 0.9238795325112867385, 1.000000000000000000, 0.9238795325112867385, 1.000000000000000000, 0.9754817479996107377, 0.9667580569362973497) ) ) 
 REPRESENTATION_ITEM ( '' )  SURFACE ( )  );
#18995=CARTESIAN_POINT ( 'NONE',  ( 13.87490072368896676, 4.990068513505961256, 3.999999999999998224 ) ) ;
#18996=CARTESIAN_POINT ( 'NONE',  ( 1.407845757905374695, -8.364917468222230923, 1.622643865078341907 ) ) ;
#19003=CARTESIAN_POINT ( 'NONE',  ( -2.645259258103298983, -10.28229522185712241, 2.672449792925449596 ) ) ;
#19005=CARTESIAN_POINT ( 'NONE',  ( 13.27780858231679417, -21.02099543870833998, 3.035098964749253003 ) ) ;
#19006=CARTESIAN_POINT ( 'NONE',  ( -12.62500000000002132, -19.50000000000273559, 4.083333333315724012 ) ) ;
#19007=CARTESIAN_POINT ( 'NONE',  ( -12.90280858231679595, -22.46490103525074034, 2.520995438708341307 ) ) ;
#19008=CARTESIAN_POINT ( 'NONE',  ( -7.284691417683176518, -24.52099543870834708, 4.484846433055073689 ) ) ;
#19012=CARTESIAN_POINT ( 'NONE',  ( 13.37499999999998401, -19.49999999999998934, 2.439580858552613751 ) ) ;
#19015=CIRCLE ( 'NONE', #9973, 0.3749999999999997224 ) ;
#19018=CARTESIAN_POINT ( 'NONE',  ( 3.277163086644854229, -14.76879761173520578, 3.824673233536266537 ) ) ;
#19022=CARTESIAN_POINT ( 'NONE',  ( 10.75344141768317741, -21.94931252712233061, 1.749999999999998446 ) ) ;
#19025=CARTESIAN_POINT ( 'NONE',  ( -1.797604806073912709, -9.120796646272857799, 2.374153755450133740 ) ) ;
#19027=CARTESIAN_POINT ( 'NONE',  ( -10.27780858231679417, -20.27099543870833642, 2.724438792969431589 ) ) ;
#19029=CARTESIAN_POINT ( 'NONE',  ( 4.378441417683176518, -24.50000000000000000, 3.449312527122335048 ) ) ;
#19031=CARTESIAN_POINT ( 'NONE',  ( -8.690941417683177406, -23.27327832286946219, 4.701595411283453707 ) ) ;
#19032=ORIENTED_EDGE ( 'NONE', *, *, #9784, .T. ) ;
#19033=CARTESIAN_POINT ( 'NONE',  ( 7.746558582316794173, -21.94931252712234482, 5.250000000000000888 ) ) ;
#19036=CARTESIAN_POINT ( 'NONE',  ( -12.66383876651304874, -19.03864229108970463, 6.262079579155994224 ) ) ;
#19048=CARTESIAN_POINT ( 'NONE',  ( -13.27780858231679417, -19.52099543870833642, 2.413778621189609286 ) ) ;
#19051=CARTESIAN_POINT ( 'NONE',  ( 2.088806020750596737, -10.42712783963456857, 1.767030719737609168 ) ) ;
#19054=CARTESIAN_POINT ( 'NONE',  ( -13.64827103573800571, -5.699812695207630675, 5.034333296717131034 ) ) ;
#19055=CARTESIAN_POINT ( 'NONE',  ( 10.09030858231679595, -21.32581373872472597, 1.729004561291657582 ) ) ;
#19056=CARTESIAN_POINT ( 'NONE',  ( -12.66204031416134335, -19.12946413485185104, 6.260126454156002218 ) ) ;
#19058=CARTESIAN_POINT ( 'NONE',  ( 4.717959273841178636, -21.72818306014730183, 5.243595146365860771 ) ) ;
#19059=CARTESIAN_POINT ( 'NONE',  ( 5.128441417683177406, -20.99999999999999645, 3.550687472877664952 ) ) ;
#19060=CARTESIAN_POINT ( 'NONE',  ( -6.996558582316793284, -22.05068747287764452, 1.749999999999998446 ) ) ;
#19062=CARTESIAN_POINT ( 'NONE',  ( 13.68663801924254741, -3.762280028282741551, 5.075999963380942503 ) ) ;
#19063=CARTESIAN_POINT ( 'NONE',  ( 0.000000000000000000, -9.114917468222230923, 1.622643865078341019 ) ) ;
#19064=ORIENTED_EDGE ( 'NONE', *, *, #2699, .T. ) ;
#19068=AXIS2_PLACEMENT_3D ( 'NONE', #13508, #20114, #15388 ) ;
#19072=CARTESIAN_POINT ( 'NONE',  ( -3.722205087890566144, -11.52065056559861134, 2.433099166587254558 ) ) ;
#19075=CARTESIAN_POINT ( 'NONE',  ( -12.63465172146706728, -19.76258806590802664, 5.372658420469845986 ) ) ;
#19076=CARTESIAN_POINT ( 'NONE',  ( 11.87155858231679417, -20.24999999999999289, 3.449312527122348371 ) ) ;
#19079=CARTESIAN_POINT ( 'NONE',  ( 13.12860732321105139, 4.432169822159808703, 6.709107302035562270 ) ) ;
#19080=CARTESIAN_POINT ( 'NONE',  ( -6.434058582316796837, -23.73192549717337130, 5.303608408759367343 ) ) ;
#19081=CARTESIAN_POINT ( 'NONE',  ( -2.124709647372160060, -10.68204274815009924, 1.832497960681391147 ) ) ;
#19083=CARTESIAN_POINT ( 'NONE',  ( -13.87066368810231154, 4.781016249162736820, 5.617237349937618696 ) ) ;
#19087=CARTESIAN_POINT ( 'NONE',  ( 8.597191417683177406, -23.08622137881040359, 5.979004561291654696 ) ) ;
#19088=CARTESIAN_POINT ( 'NONE',  ( -5.222191417683177406, -21.02099543870834353, 3.964901035250761208 ) ) ;
#19091=CARTESIAN_POINT ( 'NONE',  ( 13.37500027835944039, -20.99998594284889464, 4.544258551573043370 ) ) ;
#19092=AXIS2_PLACEMENT_3D ( 'NONE', #11661, #9795, #3517 ) ;
#19094=DIRECTION ( 'NONE',  ( -1.000000000000000000, -0.000000000000000000, -0.000000000000000000 ) ) ;
#19102=CARTESIAN_POINT ( 'NONE',  ( 2.109407804498405703, -9.207748739546751438, 2.396484790045401603 ) ) ;
#19105=CARTESIAN_POINT ( 'NONE',  ( 2.768424032093183662, -10.00067216410020166, 1.850123365707658785 ) ) ;
#19112=CARTESIAN_POINT ( 'NONE',  ( -1.797604806073912709, -9.120796646272857799, 2.374153755450133740 ) ) ;
#19113=CARTESIAN_POINT ( 'NONE',  ( 3.944195004867014909, -21.80034658733847053, 4.481176709221804444 ) ) ;
#19114=CARTESIAN_POINT ( 'NONE',  ( -12.65650603190776025, -18.65894538865861563, 5.520212342915047365 ) ) ;
#19116=CARTESIAN_POINT ( 'NONE',  ( -12.34030858231679240, -22.67418626127525982, 5.270995438708342640 ) ) ;
#19117=CARTESIAN_POINT ( 'NONE',  ( -11.59719141768317563, -22.77556120703057729, 5.229004561291655584 ) ) ;
#19119=CARTESIAN_POINT ( 'NONE',  ( 13.09455366754861139, 4.212460211200554916, 5.160171780694988719 ) ) ;
#19126=EDGE_CURVE ( 'NONE', #17639, #17561, #2541, .T. ) ;
#19127=( BOUNDED_CURVE ( )  B_SPLINE_CURVE ( 2, ( #6358, #6244, #7919, #9587, #15963, #9695, #7822, #12727, #4574, #12617, #6563, #1852, #14600, #17329, #11365, #14283, #17640, #19328, #1646, #8028, #19022, #11259, #12926, #20694, #14398, #3314, #79, #9801, #6468, #16185, #275, #1444, #178, #4675, #12828, #11070, #19230, #17754, #4881, #3117, #16082, #8236, #1753, #9492, #18916, #4986, #6666, #10961, #3014, #9391, #15763, #14185, #20593, #3729, #16576, #14813, #2253, #10003, #6969, #17855, #13340, #389, #10209, #19632, #5290, #16281, #16381, #3522, #8640, #1952, #19742, #11875, #2059, #8445, #488, #6867, #8333, #7081, #10312, #11666, #5094, #18266, #18063, #14710, #6772, #13235, #3928, #13445, #13141, #10108, #16484, #16682, #11474, #2156, #8539 ),
 .UNSPECIFIED., .F., .F. ) 
 B_SPLINE_CURVE_WITH_KNOTS ( ( 3, 2, 2, 2, 2, 2, 2, 2, 2, 2, 2, 2, 2, 2, 2, 2, 2, 2, 2, 2, 2, 2, 2, 2, 2, 2, 2, 2, 2, 2, 2, 2, 2, 2, 2, 2, 2, 2, 2, 2, 2, 2, 2, 2, 2, 2, 2, 3 ),
 ( 0.000000000000000000, 0.02083333333333333218, 0.04166666666666666435, 0.06250000000000000000, 0.08333333333333332871, 0.1041666666666666713, 0.1250000000000000000, 0.1458333333333333426, 0.1666666666666666574, 0.1875000000000000000, 0.2083333333333333426, 0.2291666666666666574, 0.2500000000000000000, 0.2708333333333333148, 0.2916666666666666852, 0.3124999999999999445, 0.3333333333333333148, 0.3541666666666666852, 0.3750000000000000000, 0.3958333333333333148, 0.4166666666666666852, 0.4375000000000000555, 0.4583333333333333148, 0.4791666666666666852, 0.5000000000000000000, 0.5208333333333333703, 0.5416666666666666297, 0.5625000000000000000, 0.5833333333333333703, 0.6041666666666666297, 0.6249999999999998890, 0.6458333333333333703, 0.6666666666666666297, 0.6875000000000000000, 0.7083333333333333703, 0.7291666666666666297, 0.7500000000000000000, 0.7708333333333333703, 0.7916666666666666297, 0.8125000000000000000, 0.8333333333333333703, 0.8541666666666666297, 0.8750000000000001110, 0.8958333333333333703, 0.9166666666666666297, 0.9375000000000000000, 0.9583333333333333703, 0.9650437087885355147 ),
 .UNSPECIFIED. ) 
 CURVE ( )  GEOMETRIC_REPRESENTATION_ITEM ( )  RATIONAL_B_SPLINE_CURVE ( ( 1.000000000000000000, 0.9238795325112867385, 1.000000000000000000, 0.9238795325112867385, 1.000000000000000000, 0.9238795325112867385, 1.000000000000000000, 0.9238795325112867385, 1.000000000000000000, 0.9238795325112867385, 1.000000000000000000, 0.9238795325112867385, 1.000000000000000000, 0.9238795325112867385, 1.000000000000000000, 0.9238795325112867385, 1.000000000000000000, 0.9238795325112867385, 1.000000000000000000, 0.9238795325112867385, 1.000000000000000000, 0.9238795325112867385, 1.000000000000000000, 0.9238795325112867385, 1.000000000000000000, 0.9238795325112867385, 1.000000000000000000, 0.9238795325112867385, 1.000000000000000000, 0.9238795325112867385, 1.000000000000000000, 0.9238795325112867385, 1.000000000000000000, 0.9238795325112867385, 1.000000000000000000, 0.9238795325112867385, 1.000000000000000000, 0.9238795325112867385, 1.000000000000000000, 0.9238795325112867385, 1.000000000000000000, 0.9238795325112867385, 1.000000000000000000, 0.9238795325112867385, 1.000000000000000000, 0.9238795325112867385, 1.000000000000000000, 0.9238795325112867385, 1.000000000000000000, 0.9238795325112867385, 1.000000000000000000, 0.9238795325112867385, 1.000000000000000000, 0.9238795325112867385, 1.000000000000000000, 0.9238795325112867385, 1.000000000000000000, 0.9238795325112867385, 1.000000000000000000, 0.9238795325112867385, 1.000000000000000000, 0.9238795325112867385, 1.000000000000000000, 0.9238795325112867385, 1.000000000000000000, 0.9238795325112867385, 1.000000000000000000, 0.9238795325112867385, 1.000000000000000000, 0.9238795325112867385, 1.000000000000000000, 0.9238795325112867385, 1.000000000000000000, 0.9238795325112867385, 1.000000000000000000, 0.9238795325112867385, 1.000000000000000000, 0.9238795325112867385, 1.000000000000000000, 0.9238795325112867385, 1.000000000000000000, 0.9238795325112867385, 1.000000000000000000, 0.9238795325112867385, 1.000000000000000000, 0.9238795325112867385, 1.000000000000000000, 0.9238795325112867385, 1.000000000000000000, 0.9238795325112867385, 1.000000000000000000, 0.9238795325112867385, 1.000000000000000000, 0.9754817479996107377, 0.9667580569362973497 ) ) 
 REPRESENTATION_ITEM ( '' )  );
#19130=CARTESIAN_POINT ( 'NONE',  ( 13.12500000000000178, 5.000000000000047962, 2.000000000000000000 ) ) ;
#19132=CARTESIAN_POINT ( 'NONE',  ( -1.407845757905374695, -9.114917468222230923, 2.372643865078341019 ) ) ;
#19134=CARTESIAN_POINT ( 'NONE',  ( -9.996558582316794173, -22.05068747287764452, 1.749999999999998446 ) ) ;
#19137=CARTESIAN_POINT ( 'NONE',  ( 6.440941417683175629, -20.19639159124061933, 1.768074502826635586 ) ) ;
#19140=CARTESIAN_POINT ( 'NONE',  ( -5.972191417683179182, -23.72900456129165292, 2.724438792969417822 ) ) ;
#19142=CARTESIAN_POINT ( 'NONE',  ( 7.934058582316792396, -23.20159541128345992, 4.773278322869455970 ) ) ;
#19144=CARTESIAN_POINT ( 'NONE',  ( -13.90439735423812273, 5.734566389025032684, 2.999999999999999556 ) ) ;
#19145=CARTESIAN_POINT ( 'NONE',  ( 5.027808582316793284, -23.72900456129165647, 4.275561207030568411 ) ) ;
#19155=CARTESIAN_POINT ( 'NONE',  ( -6.527808582316794173, -23.72900456129165647, 4.275561207030568411 ) ) ;
#19156=CARTESIAN_POINT ( 'NONE',  ( 12.64387510712649565, -19.29680709011273976, 5.506486987317513737 ) ) ;
#19159=CARTESIAN_POINT ( 'NONE',  ( 1.859341899742023463, -9.902476528685241419, 1.632289782122827271 ) ) ;
#19161=CARTESIAN_POINT ( 'NONE',  ( -13.84074239313819277, 4.019990853478630832, 5.241358430878110930 ) ) ;
#19162=CARTESIAN_POINT ( 'NONE',  ( 6.059058582316793284, -20.72672167713054137, 4.701595411283463477 ) ) ;
#19163=CARTESIAN_POINT ( 'NONE',  ( -12.68302225826488616, -18.06987595762608478, 6.282912912489355683 ) ) ;
#19167=CARTESIAN_POINT ( 'NONE',  ( -9.996558582316795949, -22.05068747287764452, 0.9999999999999978906 ) ) ;
#19168=CARTESIAN_POINT ( 'NONE',  ( 5.121558582316794173, -23.74999999999999645, 3.550687472877651629 ) ) ;
#19169=CARTESIAN_POINT ( 'NONE',  ( 3.944195004867014909, -21.80034658733847053, 4.481176709221804444 ) ) ;
#19170=CARTESIAN_POINT ( 'NONE',  ( -4.190941417683176518, -23.27327832286946219, 4.701595411283453707 ) ) ;
#19172=CARTESIAN_POINT ( 'NONE',  ( 13.84476264919594612, 4.223013784394161974, 5.079233071712400793 ) ) ;
#19180=CARTESIAN_POINT ( 'NONE',  ( -3.422464802389687311, -10.54865018547243061, 2.933470051312085936 ) ) ;
#19182=DIRECTION ( 'NONE',  ( 0.1351665943404306014, -0.9596796555888912339, 0.2464649070825229438 ) ) ;
#19183=CARTESIAN_POINT ( 'NONE',  ( -13.10821839766814279, 4.152529082241303904, 5.997503362667785609 ) ) ;
#19184=CARTESIAN_POINT ( 'NONE',  ( 13.27780858231679595, -20.27099543870833642, 2.724438792969431589 ) ) ;
#19186=CARTESIAN_POINT ( 'NONE',  ( 13.11644927503132330, 3.818188389080370282, 6.753616037489316604 ) ) ;
#19187=CARTESIAN_POINT ( 'NONE',  ( -1.863950040896528604, -9.995453039732266731, 2.406168007552154098 ) ) ;
#19189=CARTESIAN_POINT ( 'NONE',  ( -13.87467358130843387, 4.983515856073828409, 5.065827972856573602 ) ) ;
#19191=ADVANCED_FACE ( 'NONE', ( #10574 ), #17510, .T. ) ;
#19192=CARTESIAN_POINT ( 'NONE',  ( 7.472191417683177406, -24.47900456129165292, 2.413778621189595963 ) ) ;
#19193=CARTESIAN_POINT ( 'NONE',  ( -4.940941417683177406, -21.25705176302044208, 2.828734674606458555 ) ) ;
#19195=CARTESIAN_POINT ( 'NONE',  ( 12.62499963760179256, -21.00001830110826972, 4.442557003548452066 ) ) ;
#19196=CARTESIAN_POINT ( 'NONE',  ( 13.12529397354238192, 5.014845663890295846, 4.666666666666619889 ) ) ;
#19205=CARTESIAN_POINT ( 'NONE',  ( 2.081625295426255295, -10.37614485793134556, 1.753937271548854815 ) ) ;
#19207=CARTESIAN_POINT ( 'NONE',  ( 2.693754455098655409, -9.955255285363838524, 2.600628789231445470 ) ) ;
#19208=DIRECTION ( 'NONE',  ( 0.1351665943404306014, -0.9596796555888912339, 0.2464649070825229438 ) ) ;
#19213=CARTESIAN_POINT ( 'NONE',  ( 10.27780858231679595, -21.02099543870833998, 3.035098964749253003 ) ) ;
#19214=CARTESIAN_POINT ( 'NONE',  ( -13.09073190589589331, 4.019461247742575516, 5.257453802652931607 ) ) ;
#19215=CARTESIAN_POINT ( 'NONE',  ( -13.37155858231679417, -20.24999999999999289, 3.449312527122348371 ) ) ;
#19216=EDGE_CURVE ( 'NONE', #10614, #7438, #16845, .T. ) ;
#19217=CARTESIAN_POINT ( 'NONE',  ( -4.659691417683177406, -22.98484643305507191, 0.9790045612916508100 ) ) ;
#19219=CARTESIAN_POINT ( 'NONE',  ( 13.38569699238614952, -18.95980188449660986, 4.749177046715717054 ) ) ;
#19230=CARTESIAN_POINT ( 'NONE',  ( 9.253441417683177406, -21.94931252712233061, 1.749999999999998446 ) ) ;
#19232=CARTESIAN_POINT ( 'NONE',  ( -2.203959450683124377, -9.262433282444222371, 2.410528873095051594 ) ) ;
#19233=FACE_OUTER_BOUND ( 'NONE', #4748, .T. ) ;
#19237=CARTESIAN_POINT ( 'NONE',  ( 10.47219141768317563, -23.72900456129165292, 2.724438792969417822 ) ) ;
#19239=CARTESIAN_POINT ( 'NONE',  ( -11.87844141768317741, -22.99999999999999645, 3.449312527122335048 ) ) ;
#19242=CARTESIAN_POINT ( 'NONE',  ( 11.59030858231679595, -21.01515356694490322, 0.9790045612916562501 ) ) ;
#19244=CARTESIAN_POINT ( 'NONE',  ( -12.62499999999998401, -20.99999999999999645, 3.146526952850934755 ) ) ;
#19245=ORIENTED_EDGE ( 'NONE', *, *, #18846, .F. ) ;
#19246=CARTESIAN_POINT ( 'NONE',  ( 6.059058582316793284, -20.72672167713054137, 4.701595411283463477 ) ) ;
#19254=CARTESIAN_POINT ( 'NONE',  ( -4.746558582316793284, -21.94931252712234482, 5.250000000000000888 ) ) ;
#19257=CARTESIAN_POINT ( 'NONE',  ( 2.049450250860079592, -10.15122911285664564, 1.696174415070213382 ) ) ;
#19258=CARTESIAN_POINT ( 'NONE',  ( 12.65650603190776025, -18.65894538865861563, 5.520212342915047365 ) ) ;
#19260=CARTESIAN_POINT ( 'NONE',  ( -13.39888564296547635, -18.29377503024027263, 4.763499963382565205 ) ) ;
#19261=CARTESIAN_POINT ( 'NONE',  ( 8.215308582316792396, -23.77099543870833998, 2.825813738724734847 ) ) ;
#19262=CARTESIAN_POINT ( 'NONE',  ( -12.65457057572495181, -19.50668592589112293, 6.238308001337955488 ) ) ;
#19266=CARTESIAN_POINT ( 'NONE',  ( -9.340308582316795949, -22.98484643305508612, 6.020995438708344416 ) ) ;
#19267=CARTESIAN_POINT ( 'NONE',  ( 5.965308582316793284, -20.22900456129164937, 4.174186261275266929 ) ) ;
#19268=CARTESIAN_POINT ( 'NONE',  ( 6.909691417683176518, -21.63647391050456648, 4.520995438708348857 ) ) ;
#19269=CARTESIAN_POINT ( 'NONE',  ( -6.159691417683176518, -22.67418626127524917, 1.729004561291651587 ) ) ;
#19272=CARTESIAN_POINT ( 'NONE',  ( 13.84256985046264710, 4.112277448363203192, 5.213861325540929847 ) ) ;
#19275=VERTEX_POINT ( 'NONE', #10150 ) ;
#19282=CARTESIAN_POINT ( 'NONE',  ( -1.884282074604925583, -8.375506800461993251, 2.375363417140690547 ) ) ;
#19285=CARTESIAN_POINT ( 'NONE',  ( -13.12119116326504908, 4.807653744879115010, 5.626470997801169105 ) ) ;
#19286=CARTESIAN_POINT ( 'NONE',  ( 12.34030858231679240, -22.67418626127525982, 5.270995438708342640 ) ) ;
#19288=CARTESIAN_POINT ( 'NONE',  ( 12.62500000000001954, -20.24999999999450040, 3.833333333368183382 ) ) ;
#19289=CARTESIAN_POINT ( 'NONE',  ( -2.557403344953185442, -14.91030650174552896, 3.668400560659690779 ) ) ;
#19292=CARTESIAN_POINT ( 'NONE',  ( -13.85343352903393388, 3.910893216212274925, 5.991044282956552891 ) ) ;
#19294=CARTESIAN_POINT ( 'NONE',  ( 4.940941417683177406, -20.19639159124061933, 1.768074502826635586 ) ) ;
#19295=CARTESIAN_POINT ( 'NONE',  ( -9.996558582316795949, -22.05068747287764452, 2.499999999999999112 ) ) ;
#19297=CARTESIAN_POINT ( 'NONE',  ( 12.62927505847832776, -20.78410954684871825, 5.373974324164845662 ) ) ;
#19298=CARTESIAN_POINT ( 'NONE',  ( 13.12424783836753228, 4.962015837561366993, 5.328858059679200565 ) ) ;
#19307=CARTESIAN_POINT ( 'NONE',  ( 1.896776615114361908, -10.21987218505477024, 2.463803327293850209 ) ) ;
#19310=DIRECTION ( 'NONE',  ( 0.1351665943404306014, -0.9596796555888911229, 0.2464649070825229160 ) ) ;
#19315=CARTESIAN_POINT ( 'NONE',  ( -13.09455366754861139, 4.212460211200554916, 5.160171780694988719 ) ) ;
#19316=CARTESIAN_POINT ( 'NONE',  ( -12.80905858231679417, -23.27327832286945153, 2.298404588716537411 ) ) ;
#19317=CARTESIAN_POINT ( 'NONE',  ( -8.315941417683177406, -20.79840458871654363, 4.773278322869464851 ) ) ;
#19319=CARTESIAN_POINT ( 'NONE',  ( 13.37847682517167947, -19.32442032882675775, 4.733786629989340078 ) ) ;
#19321=ORIENTED_EDGE ( 'NONE', *, *, #18837, .F. ) ;
#19322=VERTEX_POINT ( 'NONE', #8686 ) ;
#19328=CARTESIAN_POINT ( 'NONE',  ( 11.03469141768317918, -20.22900456129164581, 2.825813738724748170 ) ) ;
#19333=CARTESIAN_POINT ( 'NONE',  ( -9.715308582316794173, -23.77099543870833998, 2.825813738724734847 ) ) ;
#19334=VECTOR ( 'NONE', #3990, 1000.000000000000000 ) ;
#19338=CARTESIAN_POINT ( 'NONE',  ( 9.065941417683177406, -23.20159541128344927, 2.226721677130534705 ) ) ;
#19340=CARTESIAN_POINT ( 'NONE',  ( -10.75344141768317741, -21.94931252712233061, 2.499999999999999112 ) ) ;
#19342=CARTESIAN_POINT ( 'NONE',  ( 10.09030858231679595, -21.01515356694490322, 0.9790045612916562501 ) ) ;
#19343=CARTESIAN_POINT ( 'NONE',  ( 13.11017182064853159, 4.251176942750957366, 5.979809059808775196 ) ) ;
#19344=CARTESIAN_POINT ( 'NONE',  ( -13.10745701327265778, 3.364079170269163921, 6.743850412489304169 ) ) ;
#19355=CARTESIAN_POINT ( 'NONE',  ( -12.15280858231679950, -20.91377862118960351, 5.979004561291660913 ) ) ;
#19356=CARTESIAN_POINT ( 'NONE',  ( 12.62499999999998224, -20.25000000000006395, 4.416666666666681174 ) ) ;
#19359=CARTESIAN_POINT ( 'NONE',  ( 2.081625295426255295, -10.37614485793134556, 1.753937271548854815 ) ) ;
#19360=CARTESIAN_POINT ( 'NONE',  ( 13.06655316810189227, 2.048434989138931961, 5.965524842914772030 ) ) ;
#19362=CARTESIAN_POINT ( 'NONE',  ( -13.57153706873194032, -9.574878029060977624, 4.950999963380944280 ) ) ;
#19364=CARTESIAN_POINT ( 'NONE',  ( 10.37155858231679595, -19.49999999999998934, 3.449312527122348371 ) ) ;
#19365=CARTESIAN_POINT ( 'NONE',  ( -13.11644927503132330, 3.818188389080370282, 6.753616037489316604 ) ) ;
#19371=CARTESIAN_POINT ( 'NONE',  ( 10.09030858231679595, -21.63647391050454871, 2.479004561291657804 ) ) ;
#19372=CARTESIAN_POINT ( 'NONE',  ( -6.253441417683176518, -21.94931252712233061, 1.749999999999998446 ) ) ;
#19374=ORIENTED_EDGE ( 'NONE', *, *, #10896, .F. ) ;
#19375=CARTESIAN_POINT ( 'NONE',  ( 13.37500000000002132, -20.25000000000274269, 4.083333333315724012 ) ) ;
#19381=CARTESIAN_POINT ( 'NONE',  ( -13.12512971825177033, 5.006550771716304915, 5.133277049491872468 ) ) ;
#19383=AXIS2_PLACEMENT_3D ( 'NONE', #6404, #12770, #4420 ) ;
#19386=CARTESIAN_POINT ( 'NONE',  ( -2.708677329869237482, -9.785633270066144362, 1.794897081886200230 ) ) ;
#19389=CARTESIAN_POINT ( 'NONE',  ( -13.12424783836753228, 4.962015837561366993, 5.328858059679200565 ) ) ;
#19392=CARTESIAN_POINT ( 'NONE',  ( 12.64387510712649565, -19.29680709011273976, 5.506486987317513737 ) ) ;
#19396=CARTESIAN_POINT ( 'NONE',  ( -13.39542766346049518, -19.21840299524461315, 5.493648449623241170 ) ) ;
#19398=CARTESIAN_POINT ( 'NONE',  ( 7.284691417683176518, -24.52099543870834708, 4.484846433055073689 ) ) ;
#19399=CARTESIAN_POINT ( 'NONE',  ( -9.809058582316795949, -22.74294823697954016, 2.828734674606448785 ) ) ;
#19400=COLOUR_RGB ( '', 0.66274510, 0.83137255, 0.94901961) ;
#19402=CARTESIAN_POINT ( 'NONE',  ( 13.88684657106908205, 4.848251838987907014, 6.535242036940271504 ) ) ;
#19403=CARTESIAN_POINT ( 'NONE',  ( 12.64387510712649565, -19.29680709011273976, 5.506486987317513737 ) ) ;
#19409=CARTESIAN_POINT ( 'NONE',  ( 4.315753587183824180, -21.65797192216093947, 4.831781436261117335 ) ) ;
#19413=CARTESIAN_POINT ( 'NONE',  ( 1.126276606324276619, -9.114917468222230923, 1.622643865078341463 ) ) ;
#19419=CARTESIAN_POINT ( 'NONE',  ( -4.315753587183824180, -21.65797192216093947, 4.831781436261117335 ) ) ;
#19422=CARTESIAN_POINT ( 'NONE',  ( -3.162271481458107658, -13.95306990448253437, 3.615178062515473911 ) ) ;
#19424=CARTESIAN_POINT ( 'NONE',  ( -13.07840392524817474, 3.396898225032857432, 5.244490940007585422 ) ) ;
#19425=CARTESIAN_POINT ( 'NONE',  ( -6.246558582316795949, -21.94931252712234127, 4.499999999999999112 ) ) ;
#19427=CARTESIAN_POINT ( 'NONE',  ( -9.440941417683177406, -20.72672167713052715, 2.298404588716546293 ) ) ;
#19428=ORIENTED_EDGE ( 'NONE', *, *, #17435, .F. ) ;
#19429=CARTESIAN_POINT ( 'NONE',  ( 13.38449802415168932, -19.02034978033825396, 4.747874963382372471 ) ) ;
#19441=CARTESIAN_POINT ( 'NONE',  ( -1.513434189748285918, -9.864917468222230923, 2.372643865078341019 ) ) ;
#19443=CARTESIAN_POINT ( 'NONE',  ( -9.621558582316794173, -23.74999999999999645, 3.550687472877651629 ) ) ;
#19444=CARTESIAN_POINT ( 'NONE',  ( 6.440941417683176518, -20.72672167713052715, 2.298404588716546293 ) ) ;
#19446=CARTESIAN_POINT ( 'NONE',  ( -11.97219141768317918, -22.97900456129165292, 3.035098964749240125 ) ) ;
#19449=CARTESIAN_POINT ( 'NONE',  ( 12.52780858231679773, -24.47900456129166358, 4.586221378810390270 ) ) ;
#19450=CARTESIAN_POINT ( 'NONE',  ( 12.62503117662529739, -20.24842558042254836, 4.565011198945062354 ) ) ;
#19451=CARTESIAN_POINT ( 'NONE',  ( -12.62524871736568954, -20.23743977303344010, 4.661898514667671023 ) ) ;
#19460=CARTESIAN_POINT ( 'NONE',  ( 13.32807253909975920, -20.06651685969616494, 3.455426783468704244 ) ) ;
#19462=CARTESIAN_POINT ( 'NONE',  ( -8.215308582316792396, -23.77099543870833998, 2.825813738724734847 ) ) ;
#19464=CARTESIAN_POINT ( 'NONE',  ( 12.68288333306630378, -17.32689168014509207, 5.548858176248425700 ) ) ;
#19467=CARTESIAN_POINT ( 'NONE',  ( 12.64511805349267526, -19.23403829861753422, 5.507852591554869726 ) ) ;
#19469=CARTESIAN_POINT ( 'NONE',  ( -13.37500000000002132, -20.25000000000274269, 4.083333333315724012 ) ) ;
#19470=CARTESIAN_POINT ( 'NONE',  ( 11.77780858231679595, -19.52099543870833642, 2.413778621189609286 ) ) ;
#19472=CARTESIAN_POINT ( 'NONE',  ( -13.02352923685845631, -0.8742735386340954040, 6.652704579156702991 ) ) ;
#19473=CARTESIAN_POINT ( 'NONE',  ( -9.909691417683175629, -21.01515356694492098, 6.020995438708349745 ) ) ;
#19478=CARTESIAN_POINT ( 'NONE',  ( 12.24655858231679595, -21.94931252712234127, 4.499999999999999112 ) ) ;
#19479=CARTESIAN_POINT ( 'NONE',  ( -7.378441417683176518, -23.74999999999999645, 3.449312527122335492 ) ) ;
#19482=CARTESIAN_POINT ( 'NONE',  ( 13.84439157666246878, 4.204274621457510186, 5.123803251657143676 ) ) ;
#19490=CARTESIAN_POINT ( 'NONE',  ( 13.37499999999998224, -20.24999999999991829, 4.333333333333343695 ) ) ;
#19494=CARTESIAN_POINT ( 'NONE',  ( 1.548630333695928396, -9.114917468222230923, 1.622643865078341463 ) ) ;
#19495=CARTESIAN_POINT ( 'NONE',  ( -12.62500016093973620, -20.24999187254239175, 4.532396751752561848 ) ) ;
#19496=CARTESIAN_POINT ( 'NONE',  ( 4.717959273841178636, -21.72818306014730183, 5.243595146365860771 ) ) ;
#19498=CARTESIAN_POINT ( 'NONE',  ( 13.12119116326504908, 4.807653744879115010, 5.626470997801169105 ) ) ;
#19499=CARTESIAN_POINT ( 'NONE',  ( -2.109407804498405703, -9.207748739546751438, 2.396484790045401603 ) ) ;
#19500=CARTESIAN_POINT ( 'NONE',  ( -13.84983662433050178, 3.729249528687784920, 5.987138032956566214 ) ) ;
#19503=CARTESIAN_POINT ( 'NONE',  ( 8.315941417683177406, -20.79840458871654363, 4.773278322869464851 ) ) ;
#19505=CARTESIAN_POINT ( 'NONE',  ( -8.684058582316795949, -21.32873467460644079, 2.757051763020455404 ) ) ;
#19507=CARTESIAN_POINT ( 'NONE',  ( 12.62499999999998401, -20.99999999999998934, 2.439580858552613751 ) ) ;
#19508=CARTESIAN_POINT ( 'NONE',  ( 13.11740841389447709, 4.616624901677048420, 5.813473370769506765 ) ) ;
#19516=CARTESIAN_POINT ( 'NONE',  ( 2.282685604506861754, -11.80366834561962364, 2.120553820834011116 ) ) ;
#19521=CARTESIAN_POINT ( 'NONE',  ( -8.965308582316794173, -20.22900456129164937, 4.174186261275266929 ) ) ;
#19522=CARTESIAN_POINT ( 'NONE',  ( -1.513434189748285918, -8.364917468222230923, 2.372643865078341019 ) ) ;
#19524=CARTESIAN_POINT ( 'NONE',  ( -12.62958809053144549, -19.26830142816300295, 4.757073430686623361 ) ) ;
#19525=CARTESIAN_POINT ( 'NONE',  ( -4.840308582316795061, -22.36352608949544418, 4.520995438708343528 ) ) ;
#19527=CARTESIAN_POINT ( 'NONE',  ( -7.003441417683177406, -22.05068747287765873, 5.250000000000000888 ) ) ;
#19530=CARTESIAN_POINT ( 'NONE',  ( 13.82092246150448211, 3.019084305971233562, 5.221833296715730377 ) ) ;
#19539=EDGE_CURVE ( 'NONE', #11657, #4418, #7991, .T. ) ;
#19545=CARTESIAN_POINT ( 'NONE',  ( 11.22219141768317741, -20.27099543870833998, 4.275561207030583510 ) ) ;
#19547=CARTESIAN_POINT ( 'NONE',  ( -9.909691417683175629, -21.63647391050456648, 4.520995438708348857 ) ) ;
#19549=CARTESIAN_POINT ( 'NONE',  ( 8.590308582316797725, -21.01515356694490322, 0.9790045612916562501 ) ) ;
#19550=CARTESIAN_POINT ( 'NONE',  ( 13.09892531043291086, 3.683228176858501790, 6.000681092915118420 ) ) ;
#19551=CARTESIAN_POINT ( 'NONE',  ( -12.63249216759192350, -19.87164553660301536, 5.297612231341934041 ) ) ;
#19560=ORIENTED_EDGE ( 'NONE', *, *, #2699, .F. ) ;
#19561=CARTESIAN_POINT ( 'NONE',  ( 13.50000000000000178, 5.000000000000047962, 2.000000000000000000 ) ) ;
#19563=CARTESIAN_POINT ( 'NONE',  ( 13.12529397354238192, 5.014845663890295846, 4.666666666666619889 ) ) ;
#19566=CARTESIAN_POINT ( 'NONE',  ( 12.63249216759192350, -19.87164553660301536, 5.297612231341934041 ) ) ;
#19568=CARTESIAN_POINT ( 'NONE',  ( -13.37524505148396514, -20.23762490005974968, 4.659512268729234741 ) ) ;
#19569=CARTESIAN_POINT ( 'NONE',  ( 9.059058582316795949, -20.19639159124062999, 5.231925497173373074 ) ) ;
#19570=CARTESIAN_POINT ( 'NONE',  ( -13.11704875914858270, 3.848462337001107070, 6.754267079155989784 ) ) ;
#19571=CARTESIAN_POINT ( 'NONE',  ( -5.684058582316795949, -20.26807450282662160, 1.696391591240633101 ) ) ;
#19574=CARTESIAN_POINT ( 'NONE',  ( 8.777808582316797725, -21.02099543870833998, 3.035098964749253003 ) ) ;
#19575=CARTESIAN_POINT ( 'NONE',  ( -8.315941417683177406, -20.79840458871654363, 4.773278322869464851 ) ) ;
#19578=CARTESIAN_POINT ( 'NONE',  ( 13.79214722387705905, 1.565934805775630601, 5.190583296715636230 ) ) ;
#19584=CARTESIAN_POINT ( 'NONE',  ( 13.39482594849551944, -19.24878960097397140, 5.493002502378098839 ) ) ;
#19586=CARTESIAN_POINT ( 'NONE',  ( 1.513434189748285696, -9.114917468222230923, 2.372643865078341019 ) ) ;
#19590=CARTESIAN_POINT ( 'NONE',  ( -12.70672377255832686, -15.37294948583620346, 4.840845106674187548 ) ) ;
#19591=CARTESIAN_POINT ( 'NONE',  ( 7.184058582316794173, -20.79840458871652942, 2.226721677130544030 ) ) ;
#19593=CARTESIAN_POINT ( 'NONE',  ( 12.64571531779736979, -19.20387645123237164, 5.508493592915143289 ) ) ;
#19594=CARTESIAN_POINT ( 'NONE',  ( -1.797604806073912709, -9.120796646272857799, 2.374153755450133740 ) ) ;
#19596=CARTESIAN_POINT ( 'NONE',  ( 7.277808582316795061, -21.02099543870833998, 3.035098964749253003 ) ) ;
#19598=CARTESIAN_POINT ( 'NONE',  ( 11.22219141768317741, -20.27099543870833998, 4.275561207030583510 ) ) ;
#19599=CARTESIAN_POINT ( 'NONE',  ( -9.715308582316795949, -23.02099543870833998, 3.136473910504556262 ) ) ;
#19601=CARTESIAN_POINT ( 'NONE',  ( 13.90439735423812273, 5.734566389025032684, 4.333333333333380999 ) ) ;
#19602=CARTESIAN_POINT ( 'NONE',  ( 12.64511805349267526, -19.23403829861753422, 5.507852591554869726 ) ) ;
#19611=CARTESIAN_POINT ( 'NONE',  ( 1.776440835594205847, -9.874406767442327038, 1.625080906685880233 ) ) ;
#19615=CARTESIAN_POINT ( 'NONE',  ( -2.579281110863027582, -9.822567596814183233, 2.554382554832406615 ) ) ;
#19616=CARTESIAN_POINT ( 'NONE',  ( -6.434058582316794173, -23.20159541128345992, 4.773278322869455970 ) ) ;
#19617=CARTESIAN_POINT ( 'NONE',  ( -1.787053415088318609, -8.367039355952382351, 2.373188808236395886 ) ) ;
#19619=CARTESIAN_POINT ( 'NONE',  ( -12.89855869007488209, -5.685286151195387383, 5.049178440009032265 ) ) ;
#19620=CARTESIAN_POINT ( 'NONE',  ( -6.246558582316794173, -21.94931252712234482, 5.250000000000000888 ) ) ;
#19621=CARTESIAN_POINT ( 'NONE',  ( -9.815941417683177406, -20.79840458871654363, 4.773278322869464851 ) ) ;
#19623=CARTESIAN_POINT ( 'NONE',  ( 13.84402619238587206, 4.185822715484293077, 5.150938132831436533 ) ) ;
#19630=CARTESIAN_POINT ( 'NONE',  ( -13.39542766346049518, -19.21840299524461315, 5.493648449623241170 ) ) ;
#19632=CARTESIAN_POINT ( 'NONE',  ( 6.722191417683176518, -20.27099543870833998, 4.275561207030583510 ) ) ;
#19638=CARTESIAN_POINT ( 'NONE',  ( -5.496558582316794173, -22.05068747287764452, 1.749999999999998446 ) ) ;
#19641=CARTESIAN_POINT ( 'NONE',  ( 8.972191417683177406, -23.72900456129165292, 2.724438792969417822 ) ) ;
#19643=CARTESIAN_POINT ( 'NONE',  ( -6.253441417683175629, -21.94931252712233061, 2.499999999999999112 ) ) ;
#19644=CARTESIAN_POINT ( 'NONE',  ( -8.590308582316797725, -21.01515356694490322, 0.9790045612916562501 ) ) ;
#19646=CARTESIAN_POINT ( 'NONE',  ( 12.63943061533661982, -19.52125392549825733, 5.470334935344855154 ) ) ;
#19647=CARTESIAN_POINT ( 'NONE',  ( -13.15498530132288479, 5.764257716805535559, 4.666666666666618113 ) ) ;
#19649=EDGE_CURVE ( 'NONE', #2750, #17639, #2675, .T. ) ;
#19657=CARTESIAN_POINT ( 'NONE',  ( 13.10192273101908000, 3.834597916462216816, 6.003936301248457674 ) ) ;
#19659=CARTESIAN_POINT ( 'NONE',  ( 0.000000000000000000, -9.114917468222230923, 2.372643865078340575 ) ) ;
#19663=CARTESIAN_POINT ( 'NONE',  ( 13.15498530131898214, 5.764257716805535559, 3.333333333333075466 ) ) ;
#19665=CARTESIAN_POINT ( 'NONE',  ( 8.402808582316797725, -23.08622137881038938, 1.020995438708339309 ) ) ;
#19666=CARTESIAN_POINT ( 'NONE',  ( -13.15492785973632017, 5.761356916681801721, 5.116543252045025802 ) ) ;
#19667=CARTESIAN_POINT ( 'NONE',  ( -11.78469141768317741, -24.52099543870834708, 4.484846433055073689 ) ) ;
#19671=CARTESIAN_POINT ( 'NONE',  ( 11.12155858231679595, -22.99999999999999645, 3.550687472877652073 ) ) ;
#19676=CARTESIAN_POINT ( 'NONE',  ( 13.84264281492353987, 3.365962153638767607, 5.979325532956542233 ) ) ;
#19683=CARTESIAN_POINT ( 'NONE',  ( 13.85223456079946303, 3.850345320370711644, 5.989742199623227847 ) ) ;
#19687=CARTESIAN_POINT ( 'NONE',  ( 3.302240162463773832, -9.695145533921818881, 2.714273006325518711 ) ) ;
#19690=CARTESIAN_POINT ( 'NONE',  ( -12.99447614883396973, -0.8414544838704021146, 5.153345106674984244 ) ) ;
#19691=CARTESIAN_POINT ( 'NONE',  ( 8.027808582316792396, -23.72900456129165292, 4.275561207030568411 ) ) ;
#19693=CARTESIAN_POINT ( 'NONE',  ( 12.64131715375063258, -19.42598373559290792, 5.491151580003103660 ) ) ;
#19694=CARTESIAN_POINT ( 'NONE',  ( -1.407845757905374695, -9.864917468222230923, 2.372643865078341019 ) ) ;
#19696=CARTESIAN_POINT ( 'NONE',  ( 12.52780858231679773, -22.97900456129165647, 3.964901035250747885 ) ) ;
#19697=CARTESIAN_POINT ( 'NONE',  ( 11.12844141768317741, -20.24999999999999289, 3.550687472877664952 ) ) ;
#19698=CARTESIAN_POINT ( 'NONE',  ( -6.434058582316796837, -22.67126532539354855, 4.242948236979545484 ) ) ;
#19700=CARTESIAN_POINT ( 'NONE',  ( 12.96597876160390683, -3.780572539034193102, 6.590204579154564257 ) ) ;
#19701=CARTESIAN_POINT ( 'NONE',  ( 12.62837453896009876, -19.32958578251692572, 4.742959489302074338 ) ) ;
#19703=CARTESIAN_POINT ( 'NONE',  ( -12.80505314591509070, -19.91502843109724097, 3.526594361829830326 ) ) ;
#19714=CARTESIAN_POINT ( 'NONE',  ( -4.121804964265450621, -21.50709082768453939, 5.525644484121333022 ) ) ;
#19715=CARTESIAN_POINT ( 'NONE',  ( 0.2815691515810352374, -9.864917468222230923, 2.372643865078523540 ) ) ;
#19718=CARTESIAN_POINT ( 'NONE',  ( 13.26220787538139589, -20.51810926806117763, 3.464229958566896084 ) ) ;
#19721=CARTESIAN_POINT ( 'NONE',  ( -5.496558582316794173, -22.05068747287764452, 1.749999999999998446 ) ) ;
#19722=CARTESIAN_POINT ( 'NONE',  ( -4.066879903460562495, -13.96783368734915776, 3.061584679647603391 ) ) ;
#19724=CARTESIAN_POINT ( 'NONE',  ( -13.68663801924254741, -3.762280028282741551, 5.075999963380942503 ) ) ;
#19725=CARTESIAN_POINT ( 'NONE',  ( -9.152808582316794173, -21.22443879296942626, 5.229004561291659137 ) ) ;
#19727=CARTESIAN_POINT ( 'NONE',  ( -5.222191417683178294, -20.27099543870833998, 4.275561207030583510 ) ) ;
#19729=CARTESIAN_POINT ( 'NONE',  ( 13.37500015856764435, -20.24999199233421265, 4.532157119432948633 ) ) ;
#19741=CIRCLE ( 'NONE', #17733, 0.3749999999999997224 ) ;
#19742=CARTESIAN_POINT ( 'NONE',  ( 6.065941417683177406, -23.20159541128344927, 2.226721677130534705 ) ) ;
#19746=CARTESIAN_POINT ( 'NONE',  ( 1.407845757905374695, -8.364917468222230923, 2.372643865078341019 ) ) ;
#19747=CARTESIAN_POINT ( 'NONE',  ( -6.246558582316794173, -21.94931252712234482, 5.250000000000000888 ) ) ;
#19748=CARTESIAN_POINT ( 'NONE',  ( 13.90439771357353038, 5.734584535470497180, 4.942866369314573127 ) ) ;
#19750=CARTESIAN_POINT ( 'NONE',  ( 11.40969141768317918, -21.63647391050456648, 4.520995438708348857 ) ) ;
#19752=CARTESIAN_POINT ( 'NONE',  ( -8.128441417683177406, -20.99999999999999645, 3.550687472877664952 ) ) ;
#19753=CARTESIAN_POINT ( 'NONE',  ( -6.621558582316796837, -24.50000000000000000, 3.550687472877651629 ) ) ;
#19755=CARTESIAN_POINT ( 'NONE',  ( 12.95145221759166354, -3.764163011652346569, 5.840524842913703552 ) ) ;
#19756=CARTESIAN_POINT ( 'NONE',  ( -12.62499999999998224, -20.25000000000006395, 4.416666666666681174 ) ) ;
#19769=CYLINDRICAL_SURFACE ( 'NONE', #17997, 0.3749999999999997224 ) ;
#19770=CARTESIAN_POINT ( 'NONE',  ( 13.08573665985359824, 3.017201322601628100, 5.986358176248492313 ) ) ;
#19771=CARTESIAN_POINT ( 'NONE',  ( -3.232228556578340850, -13.29361487011126464, 2.695816835751057461 ) ) ;
#19772=CARTESIAN_POINT ( 'NONE',  ( 0.5631383031621635116, -9.114917468222230923, 2.372643865078341019 ) ) ;
#19777=CARTESIAN_POINT ( 'NONE',  ( 12.34030858231679773, -22.98484643305508612, 6.020995438708344416 ) ) ;
#19778=CARTESIAN_POINT ( 'NONE',  ( -13.07148796623841847, 1.547642295024179493, 6.704787912489258872 ) ) ;
#19779=CARTESIAN_POINT ( 'NONE',  ( -7.940941417683175629, -20.19639159124061933, 1.768074502826635586 ) ) ;
#19784=CARTESIAN_POINT ( 'NONE',  ( 8.496558582316795949, -22.05068747287764452, 2.499999999999999112 ) ) ;
#19790=CARTESIAN_POINT ( 'NONE',  ( 13.54769662923970763, -11.52882022337116119, 5.659013032956382361 ) ) ;
#19798=CARTESIAN_POINT ( 'NONE',  ( 13.86106797245302147, 4.296432608878145487, 5.947261916831099171 ) ) ;
#19799=( BOUNDED_SURFACE ( )  B_SPLINE_SURFACE ( 3, 2, ( 
 ( #12349, #15486, #18535, #12244, #15074, #10687, #7239, #17059, #3991, #10375, #755, #7142, #19907, #4198, #13911, #5561, #7344, #16947, #11932, #16749, #13601, #2420, #8811, #9014, #20312, #5669, #5976, #4097, #16850, #15277, #15386, #18746, #13706, #1069, #20528, #19055, #17679, #12454, #12549, #18849, #4818, #3148, #15893, #9215, #12651, #1378, #2937, #12859, #4, #7947, #10894, #9317, #14430, #1678, #7853, #19261, #4603, #9618, #1573, #112, #15586, #17258, #11292, #12759, #14319, #6182, #1270, #15693, #16001, #17471, #7647, #9521, #3244, #6394, #8067, #18947, #10995, #14019, #19162, #7756, #11195, #4510, #17572, #6498, #20427, #4915, #14123, #17364, #3051, #6087, #9426, #15795, #14217, #1476, #20624 ),
 ( #6277, #4712, #11100, #11505, #5020, #10037, #10144, #18099, #5125, #7006, #13169, #19777, #17885, #11400, #13071, #16312, #16515, #19470, #3453, #13374, #3350, #1985, #16415, #8475, #2187, #14745, #9730, #8571, #5435, #17984, #6898, #14631, #19364, #11702, #16114, #11808, #3655, #3764, #8372, #421, #3552, #619, #1782, #8169, #6801, #9932, #19569, #14941, #14535, #210, #17785, #6594, #5222, #19665, #12962, #9831, #13266, #16216, #11600, #14842, #1884, #8265, #316, #5328, #6700, #2090, #517, #18610, #4270, #15045, #10554, #5638, #19977, #12011, #18199, #828, #10239, #3862, #8883, #13887, #18296, #19880, #16605, #5536, #20083, #2597, #8985, #2490, #15252, #9091, #18512, #2395, #10657, #4172, #2709 ),
 ( #13575, #18407, #7523, #5750, #15461, #17031, #13786, #16923, #4071, #15358, #7213, #5851, #20288, #1038, #2285, #5946, #12220, #10457, #8676, #16826, #1146, #928, #7315, #15154, #7114, #7424, #13676, #3959, #730, #13477, #20191, #12120, #11906, #10347, #16719, #8785, #3022, #6251, #6159, #12526, #2814, #20702, #14291, #13988, #4789, #1350, #9188, #7830, #17339, #10767, #9593, #3223, #18923, #17235, #1546, #14192, #3124, #10870, #9499, #7731, #20599, #6365, #14403, #12734, #18823, #15970, #19137, #15770, #15870, #1653, #7925, #4486, #11172, #15563, #1246, #8037, #88, #12319, #1452, #17545, #18717, #4581, #12625, #4384, #17135, #2914, #7619, #20396, #19029, #17446, #6059, #4684, #12429, #9290, #20505 ),
 ( #15665, #14096, #10968, #9398, #11075, #11267, #5299, #6568, #2067, #3531, #12933, #13148, #17861, #14606, #8145, #19545, #13243, #494, #8241, #10119, #16288, #2163, #284, #19237, #14508, #8342, #11578, #17957, #11481, #9906, #18071, #6778, #11372, #8547, #10010, #3629, #17761, #14917, #19338, #19641, #14718, #4887, #395, #6874, #5200, #11674, #9807, #1858, #12834, #16389, #4993, #8452, #16089, #14819, #3737, #17647, #16491, #3430, #186, #16194, #3321, #6675, #13044, #5102, #9703, #6475, #19444, #1759, #1959, #7088, #7289, #11988, #8759, #2261, #13652, #7403, #15332, #2371, #4250, #10432, #17007, #15132, #8650, #10324, #13553, #13764, #16693, #703, #10630, #595, #19954, #20063, #5727, #20168, #18386 ),
 ( #15230, #4149, #11882, #16584, #8957, #13349, #2684, #904, #1012, #5612, #4049, #806, #18587, #19750, #5408, #16801, #7190, #2470, #5828, #9070, #12197, #15022, #6981, #8861, #16901, #10216, #11782, #10532, #18174, #12098, #18488, #3837, #13453, #19857, #2572, #5510, #18274, #3936, #15848, #1527, #12296, #7810, #2892, #17214, #9268, #15442, #18800, #7504, #1126, #6137, #11151, #15544, #17113, #4359, #1429, #4561, #1224, #13867, #20266, #14172, #10946, #18904, #14270, #15747, #3202, #12506, #9373, #15640, #1329, #5925, #3101, #17425, #2795, #7906, #4466, #18693, #17312, #20481, #10743, #12711, #6340, #7705, #20371, #4661, #2997, #6232, #13966, #12602, #10851, #20579, #9478, #17521, #20677, #7599, #19113 ),
 ( #4766, #19005, #6034, #9169, #12406, #14073, #11052, #5564, #18330, #19696, #18227, #9573, #16446, #5359, #15946, #14381, #16065, #64, #6450, #13295, #14970, #19911, #2216, #8008, #12814, #18017, #11736, #8599, #649, #8706, #450, #18129, #1628, #19213, #13198, #4867, #5465, #3794, #16541, #11246, #10171, #1738, #3297, #13509, #7037, #13405, #17625, #9679, #15077, #2317, #8501, #11936, #5249, #10269, #19811, #760, #8120, #14487, #11837, #11627, #3687, #6828, #3890, #7145, #16638, #19596, #10071, #2119, #14871, #547, #6926, #6090, #2741, #10379, #20432, #12355, #16952, #16752, #5778, #2842, #9018, #12148, #958, #10799, #1273, #17166, #20009, #9218, #20115, #20316, #13604, #14023, #13914, #2424, #20217 ),
 ( #5672, #15589, #13709, #860, #5878, #15389, #8815, #7652, #12458, #10584, #8913, #5980, #12248, #15490, #2521, #1173, #18538, #18640, #18749, #3995, #4413, #10484, #15183, #7243, #7453, #7552, #12044, #18437, #16854, #4101, #15281, #7348, #4202, #2630, #1072, #13814, #4306, #10691, #17062, #9121, #4513, #2940, #4606, #9321, #15697, #1577, #3248, #8172, #11201, #17261, #1381, #6281, #10, #17576, #9622, #17684, #9429, #7951, #6599, #7761, #1478, #14127, #14435, #12763, #4822, #18852, #14325, #10999, #12552, #1786, #16006, #1685, #20531, #18951, #3354, #11296, #17476, #14539, #14220, #19267, #8071, #9734, #10898, #6185, #6398, #20627, #12655, #213, #19168, #16118, #4919, #117, #6503, #19058, #12863 ) ),
 .UNSPECIFIED., .T., .F., .T. ) 
 B_SPLINE_SURFACE_WITH_KNOTS ( ( 4, 3, 4 ),
 ( 3, 2, 2, 2, 2, 2, 2, 2, 2, 2, 2, 2, 2, 2, 2, 2, 2, 2, 2, 2, 2, 2, 2, 2, 2, 2, 2, 2, 2, 2, 2, 2, 2, 2, 2, 2, 2, 2, 2, 2, 2, 2, 2, 2, 2, 2, 2, 3 ),
 ( 0.000000000000000000, 0.5000000000000000000, 1.000000000000000000 ),
 ( 0.000000000000000000, 0.02083333333333333218, 0.04166666666666666435, 0.06250000000000000000, 0.08333333333333332871, 0.1041666666666666713, 0.1250000000000000000, 0.1458333333333333426, 0.1666666666666666574, 0.1875000000000000000, 0.2083333333333333426, 0.2291666666666666574, 0.2500000000000000000, 0.2708333333333333148, 0.2916666666666666852, 0.3125000000000000000, 0.3333333333333333148, 0.3541666666666666852, 0.3750000000000000000, 0.3958333333333333148, 0.4166666666666666852, 0.4375000000000000000, 0.4583333333333333148, 0.4791666666666666852, 0.5000000000000000000, 0.5208333333333333703, 0.5416666666666666297, 0.5625000000000000000, 0.5833333333333333703, 0.6041666666666666297, 0.6250000000000000000, 0.6458333333333333703, 0.6666666666666666297, 0.6875000000000000000, 0.7083333333333333703, 0.7291666666666666297, 0.7500000000000000000, 0.7708333333333333703, 0.7916666666666666297, 0.8125000000000000000, 0.8333333333333333703, 0.8541666666666666297, 0.8750000000000000000, 0.8958333333333333703, 0.9166666666666666297, 0.9375000000000000000, 0.9583333333333333703, 0.9650437087885355147 ),
 .UNSPECIFIED. ) 
 GEOMETRIC_REPRESENTATION_ITEM ( )  RATIONAL_B_SPLINE_SURFACE ( (
 ( 1.000000000000000000, 0.9238795325112867385, 1.000000000000000000, 0.9238795325112867385, 1.000000000000000000, 0.9238795325112867385, 1.000000000000000000, 0.9238795325112867385, 1.000000000000000000, 0.9238795325112867385, 1.000000000000000000, 0.9238795325112867385, 1.000000000000000000, 0.9238795325112867385, 1.000000000000000000, 0.9238795325112867385, 1.000000000000000000, 0.9238795325112867385, 1.000000000000000000, 0.9238795325112867385, 1.000000000000000000, 0.9238795325112867385, 1.000000000000000000, 0.9238795325112867385, 1.000000000000000000, 0.9238795325112867385, 1.000000000000000000, 0.9238795325112867385, 1.000000000000000000, 0.9238795325112867385, 1.000000000000000000, 0.9238795325112867385, 1.000000000000000000, 0.9238795325112867385, 1.000000000000000000, 0.9238795325112867385, 1.000000000000000000, 0.9238795325112867385, 1.000000000000000000, 0.9238795325112867385, 1.000000000000000000, 0.9238795325112867385, 1.000000000000000000, 0.9238795325112867385, 1.000000000000000000, 0.9238795325112867385, 1.000000000000000000, 0.9238795325112867385, 1.000000000000000000, 0.9238795325112867385, 1.000000000000000000, 0.9238795325112867385, 1.000000000000000000, 0.9238795325112867385, 1.000000000000000000, 0.9238795325112867385, 1.000000000000000000, 0.9238795325112867385, 1.000000000000000000, 0.9238795325112867385, 1.000000000000000000, 0.9238795325112867385, 1.000000000000000000, 0.9238795325112867385, 1.000000000000000000, 0.9238795325112867385, 1.000000000000000000, 0.9238795325112867385, 1.000000000000000000, 0.9238795325112867385, 1.000000000000000000, 0.9238795325112867385, 1.000000000000000000, 0.9238795325112867385, 1.000000000000000000, 0.9238795325112867385, 1.000000000000000000, 0.9238795325112867385, 1.000000000000000000, 0.9238795325112867385, 1.000000000000000000, 0.9238795325112867385, 1.000000000000000000, 0.9238795325112867385, 1.000000000000000000, 0.9238795325112867385, 1.000000000000000000, 0.9238795325112867385, 1.000000000000000000, 0.9238795325112867385, 1.000000000000000000, 0.9238795325112867385, 1.000000000000000000, 0.9754817479996107377, 0.9667580569362973497),
 ( 0.3333333333333333703, 0.3079598441704289313, 0.3333333333333333703, 0.3079598441704289313, 0.3333333333333333703, 0.3079598441704289313, 0.3333333333333333703, 0.3079598441704289313, 0.3333333333333333703, 0.3079598441704289313, 0.3333333333333333703, 0.3079598441704289313, 0.3333333333333333703, 0.3079598441704289313, 0.3333333333333333703, 0.3079598441704289313, 0.3333333333333333703, 0.3079598441704289313, 0.3333333333333333703, 0.3079598441704289313, 0.3333333333333333703, 0.3079598441704289313, 0.3333333333333333703, 0.3079598441704289313, 0.3333333333333333703, 0.3079598441704289313, 0.3333333333333333703, 0.3079598441704289313, 0.3333333333333333703, 0.3079598441704289313, 0.3333333333333333703, 0.3079598441704289313, 0.3333333333333333703, 0.3079598441704289313, 0.3333333333333333703, 0.3079598441704289313, 0.3333333333333333703, 0.3079598441704289313, 0.3333333333333333703, 0.3079598441704289313, 0.3333333333333333703, 0.3079598441704289313, 0.3333333333333333703, 0.3079598441704289313, 0.3333333333333333703, 0.3079598441704289313, 0.3333333333333333703, 0.3079598441704289313, 0.3333333333333333703, 0.3079598441704289313, 0.3333333333333333703, 0.3079598441704289313, 0.3333333333333333703, 0.3079598441704289313, 0.3333333333333333703, 0.3079598441704289313, 0.3333333333333333703, 0.3079598441704289313, 0.3333333333333333703, 0.3079598441704289313, 0.3333333333333333703, 0.3079598441704289313, 0.3333333333333333703, 0.3079598441704289313, 0.3333333333333333703, 0.3079598441704289313, 0.3333333333333333703, 0.3079598441704289313, 0.3333333333333333703, 0.3079598441704289313, 0.3333333333333333703, 0.3079598441704289313, 0.3333333333333333703, 0.3079598441704289313, 0.3333333333333333703, 0.3079598441704289313, 0.3333333333333333703, 0.3079598441704289313, 0.3333333333333333703, 0.3079598441704289313, 0.3333333333333333703, 0.3079598441704289313, 0.3333333333333333703, 0.3079598441704289313, 0.3333333333333333703, 0.3079598441704289313, 0.3333333333333333703, 0.3079598441704289313, 0.3333333333333333703, 0.3079598441704289313, 0.3333333333333333703, 0.3079598441704289313, 0.3333333333333333703, 0.3251605826665369681, 0.3222526856454325239),
 ( 0.3333333333333333703, 0.3079598441704289313, 0.3333333333333333703, 0.3079598441704289313, 0.3333333333333333703, 0.3079598441704289313, 0.3333333333333333703, 0.3079598441704289313, 0.3333333333333333703, 0.3079598441704289313, 0.3333333333333333703, 0.3079598441704289313, 0.3333333333333333703, 0.3079598441704289313, 0.3333333333333333703, 0.3079598441704289313, 0.3333333333333333703, 0.3079598441704289313, 0.3333333333333333703, 0.3079598441704289313, 0.3333333333333333703, 0.3079598441704289313, 0.3333333333333333703, 0.3079598441704289313, 0.3333333333333333703, 0.3079598441704289313, 0.3333333333333333703, 0.3079598441704289313, 0.3333333333333333703, 0.3079598441704289313, 0.3333333333333333703, 0.3079598441704289313, 0.3333333333333333703, 0.3079598441704289313, 0.3333333333333333703, 0.3079598441704289313, 0.3333333333333333703, 0.3079598441704289313, 0.3333333333333333703, 0.3079598441704289313, 0.3333333333333333703, 0.3079598441704289313, 0.3333333333333333703, 0.3079598441704289313, 0.3333333333333333703, 0.3079598441704289313, 0.3333333333333333703, 0.3079598441704289313, 0.3333333333333333703, 0.3079598441704289313, 0.3333333333333333703, 0.3079598441704289313, 0.3333333333333333703, 0.3079598441704289313, 0.3333333333333333703, 0.3079598441704289313, 0.3333333333333333703, 0.3079598441704289313, 0.3333333333333333703, 0.3079598441704289313, 0.3333333333333333703, 0.3079598441704289313, 0.3333333333333333703, 0.3079598441704289313, 0.3333333333333333703, 0.3079598441704289313, 0.3333333333333333703, 0.3079598441704289313, 0.3333333333333333703, 0.3079598441704289313, 0.3333333333333333703, 0.3079598441704289313, 0.3333333333333333703, 0.3079598441704289313, 0.3333333333333333703, 0.3079598441704289313, 0.3333333333333333703, 0.3079598441704289313, 0.3333333333333333703, 0.3079598441704289313, 0.3333333333333333703, 0.3079598441704289313, 0.3333333333333333703, 0.3079598441704289313, 0.3333333333333333703, 0.3079598441704289313, 0.3333333333333333703, 0.3079598441704289313, 0.3333333333333333703, 0.3079598441704289313, 0.3333333333333333703, 0.3079598441704289313, 0.3333333333333333703, 0.3251605826665369681, 0.3222526856454325239),
 ( 1.000000000000000000, 0.9238795325112867385, 1.000000000000000000, 0.9238795325112867385, 1.000000000000000000, 0.9238795325112867385, 1.000000000000000000, 0.9238795325112867385, 1.000000000000000000, 0.9238795325112867385, 1.000000000000000000, 0.9238795325112867385, 1.000000000000000000, 0.9238795325112867385, 1.000000000000000000, 0.9238795325112867385, 1.000000000000000000, 0.9238795325112867385, 1.000000000000000000, 0.9238795325112867385, 1.000000000000000000, 0.9238795325112867385, 1.000000000000000000, 0.9238795325112867385, 1.000000000000000000, 0.9238795325112867385, 1.000000000000000000, 0.9238795325112867385, 1.000000000000000000, 0.9238795325112867385, 1.000000000000000000, 0.9238795325112867385, 1.000000000000000000, 0.9238795325112867385, 1.000000000000000000, 0.9238795325112867385, 1.000000000000000000, 0.9238795325112867385, 1.000000000000000000, 0.9238795325112867385, 1.000000000000000000, 0.9238795325112867385, 1.000000000000000000, 0.9238795325112867385, 1.000000000000000000, 0.9238795325112867385, 1.000000000000000000, 0.9238795325112867385, 1.000000000000000000, 0.9238795325112867385, 1.000000000000000000, 0.9238795325112867385, 1.000000000000000000, 0.9238795325112867385, 1.000000000000000000, 0.9238795325112867385, 1.000000000000000000, 0.9238795325112867385, 1.000000000000000000, 0.9238795325112867385, 1.000000000000000000, 0.9238795325112867385, 1.000000000000000000, 0.9238795325112867385, 1.000000000000000000, 0.9238795325112867385, 1.000000000000000000, 0.9238795325112867385, 1.000000000000000000, 0.9238795325112867385, 1.000000000000000000, 0.9238795325112867385, 1.000000000000000000, 0.9238795325112867385, 1.000000000000000000, 0.9238795325112867385, 1.000000000000000000, 0.9238795325112867385, 1.000000000000000000, 0.9238795325112867385, 1.000000000000000000, 0.9238795325112867385, 1.000000000000000000, 0.9238795325112867385, 1.000000000000000000, 0.9238795325112867385, 1.000000000000000000, 0.9238795325112867385, 1.000000000000000000, 0.9238795325112867385, 1.000000000000000000, 0.9238795325112867385, 1.000000000000000000, 0.9754817479996107377, 0.9667580569362973497),
 ( 0.3333333333333333703, 0.3079598441704289313, 0.3333333333333333703, 0.3079598441704289313, 0.3333333333333333703, 0.3079598441704289313, 0.3333333333333333703, 0.3079598441704289313, 0.3333333333333333703, 0.3079598441704289313, 0.3333333333333333703, 0.3079598441704289313, 0.3333333333333333703, 0.3079598441704289313, 0.3333333333333333703, 0.3079598441704289313, 0.3333333333333333703, 0.3079598441704289313, 0.3333333333333333703, 0.3079598441704289313, 0.3333333333333333703, 0.3079598441704289313, 0.3333333333333333703, 0.3079598441704289313, 0.3333333333333333703, 0.3079598441704289313, 0.3333333333333333703, 0.3079598441704289313, 0.3333333333333333703, 0.3079598441704289313, 0.3333333333333333703, 0.3079598441704289313, 0.3333333333333333703, 0.3079598441704289313, 0.3333333333333333703, 0.3079598441704289313, 0.3333333333333333703, 0.3079598441704289313, 0.3333333333333333703, 0.3079598441704289313, 0.3333333333333333703, 0.3079598441704289313, 0.3333333333333333703, 0.3079598441704289313, 0.3333333333333333703, 0.3079598441704289313, 0.3333333333333333703, 0.3079598441704289313, 0.3333333333333333703, 0.3079598441704289313, 0.3333333333333333703, 0.3079598441704289313, 0.3333333333333333703, 0.3079598441704289313, 0.3333333333333333703, 0.3079598441704289313, 0.3333333333333333703, 0.3079598441704289313, 0.3333333333333333703, 0.3079598441704289313, 0.3333333333333333703, 0.3079598441704289313, 0.3333333333333333703, 0.3079598441704289313, 0.3333333333333333703, 0.3079598441704289313, 0.3333333333333333703, 0.3079598441704289313, 0.3333333333333333703, 0.3079598441704289313, 0.3333333333333333703, 0.3079598441704289313, 0.3333333333333333703, 0.3079598441704289313, 0.3333333333333333703, 0.3079598441704289313, 0.3333333333333333703, 0.3079598441704289313, 0.3333333333333333703, 0.3079598441704289313, 0.3333333333333333703, 0.3079598441704289313, 0.3333333333333333703, 0.3079598441704289313, 0.3333333333333333703, 0.3079598441704289313, 0.3333333333333333703, 0.3079598441704289313, 0.3333333333333333703, 0.3079598441704289313, 0.3333333333333333703, 0.3079598441704289313, 0.3333333333333333703, 0.3251605826665369681, 0.3222526856454325239),
 ( 0.3333333333333333703, 0.3079598441704289313, 0.3333333333333333703, 0.3079598441704289313, 0.3333333333333333703, 0.3079598441704289313, 0.3333333333333333703, 0.3079598441704289313, 0.3333333333333333703, 0.3079598441704289313, 0.3333333333333333703, 0.3079598441704289313, 0.3333333333333333703, 0.3079598441704289313, 0.3333333333333333703, 0.3079598441704289313, 0.3333333333333333703, 0.3079598441704289313, 0.3333333333333333703, 0.3079598441704289313, 0.3333333333333333703, 0.3079598441704289313, 0.3333333333333333703, 0.3079598441704289313, 0.3333333333333333703, 0.3079598441704289313, 0.3333333333333333703, 0.3079598441704289313, 0.3333333333333333703, 0.3079598441704289313, 0.3333333333333333703, 0.3079598441704289313, 0.3333333333333333703, 0.3079598441704289313, 0.3333333333333333703, 0.3079598441704289313, 0.3333333333333333703, 0.3079598441704289313, 0.3333333333333333703, 0.3079598441704289313, 0.3333333333333333703, 0.3079598441704289313, 0.3333333333333333703, 0.3079598441704289313, 0.3333333333333333703, 0.3079598441704289313, 0.3333333333333333703, 0.3079598441704289313, 0.3333333333333333703, 0.3079598441704289313, 0.3333333333333333703, 0.3079598441704289313, 0.3333333333333333703, 0.3079598441704289313, 0.3333333333333333703, 0.3079598441704289313, 0.3333333333333333703, 0.3079598441704289313, 0.3333333333333333703, 0.3079598441704289313, 0.3333333333333333703, 0.3079598441704289313, 0.3333333333333333703, 0.3079598441704289313, 0.3333333333333333703, 0.3079598441704289313, 0.3333333333333333703, 0.3079598441704289313, 0.3333333333333333703, 0.3079598441704289313, 0.3333333333333333703, 0.3079598441704289313, 0.3333333333333333703, 0.3079598441704289313, 0.3333333333333333703, 0.3079598441704289313, 0.3333333333333333703, 0.3079598441704289313, 0.3333333333333333703, 0.3079598441704289313, 0.3333333333333333703, 0.3079598441704289313, 0.3333333333333333703, 0.3079598441704289313, 0.3333333333333333703, 0.3079598441704289313, 0.3333333333333333703, 0.3079598441704289313, 0.3333333333333333703, 0.3079598441704289313, 0.3333333333333333703, 0.3079598441704289313, 0.3333333333333333703, 0.3251605826665369681, 0.3222526856454325239),
 ( 1.000000000000000000, 0.9238795325112867385, 1.000000000000000000, 0.9238795325112867385, 1.000000000000000000, 0.9238795325112867385, 1.000000000000000000, 0.9238795325112867385, 1.000000000000000000, 0.9238795325112867385, 1.000000000000000000, 0.9238795325112867385, 1.000000000000000000, 0.9238795325112867385, 1.000000000000000000, 0.9238795325112867385, 1.000000000000000000, 0.9238795325112867385, 1.000000000000000000, 0.9238795325112867385, 1.000000000000000000, 0.9238795325112867385, 1.000000000000000000, 0.9238795325112867385, 1.000000000000000000, 0.9238795325112867385, 1.000000000000000000, 0.9238795325112867385, 1.000000000000000000, 0.9238795325112867385, 1.000000000000000000, 0.9238795325112867385, 1.000000000000000000, 0.9238795325112867385, 1.000000000000000000, 0.9238795325112867385, 1.000000000000000000, 0.9238795325112867385, 1.000000000000000000, 0.9238795325112867385, 1.000000000000000000, 0.9238795325112867385, 1.000000000000000000, 0.9238795325112867385, 1.000000000000000000, 0.9238795325112867385, 1.000000000000000000, 0.9238795325112867385, 1.000000000000000000, 0.9238795325112867385, 1.000000000000000000, 0.9238795325112867385, 1.000000000000000000, 0.9238795325112867385, 1.000000000000000000, 0.9238795325112867385, 1.000000000000000000, 0.9238795325112867385, 1.000000000000000000, 0.9238795325112867385, 1.000000000000000000, 0.9238795325112867385, 1.000000000000000000, 0.9238795325112867385, 1.000000000000000000, 0.9238795325112867385, 1.000000000000000000, 0.9238795325112867385, 1.000000000000000000, 0.9238795325112867385, 1.000000000000000000, 0.9238795325112867385, 1.000000000000000000, 0.9238795325112867385, 1.000000000000000000, 0.9238795325112867385, 1.000000000000000000, 0.9238795325112867385, 1.000000000000000000, 0.9238795325112867385, 1.000000000000000000, 0.9238795325112867385, 1.000000000000000000, 0.9238795325112867385, 1.000000000000000000, 0.9238795325112867385, 1.000000000000000000, 0.9238795325112867385, 1.000000000000000000, 0.9238795325112867385, 1.000000000000000000, 0.9238795325112867385, 1.000000000000000000, 0.9754817479996107377, 0.9667580569362973497) ) ) 
 REPRESENTATION_ITEM ( '' )  SURFACE ( )  );
#19801=CARTESIAN_POINT ( 'NONE',  ( 0.9854920305337621089, -9.114917468222230923, 2.372643865078341019 ) ) ;
#19804=CARTESIAN_POINT ( 'NONE',  ( 1.337453470010121714, -9.114917468222230923, 1.622643865078341463 ) ) ;
#19805=CARTESIAN_POINT ( 'NONE',  ( -12.62499999998404299, -19.49999999996810729, 2.793053905886972998 ) ) ;
#19806=CARTESIAN_POINT ( 'NONE',  ( 6.715308582316794173, -23.77099543870833998, 2.825813738724734847 ) ) ;
#19808=CARTESIAN_POINT ( 'NONE',  ( 12.62599079447150885, -20.19996487918709249, 4.820256282269618886 ) ) ;
#19810=CARTESIAN_POINT ( 'NONE',  ( -2.817596665886821672, -11.50588678273290988, 2.986692549455723267 ) ) ;
#19811=CARTESIAN_POINT ( 'NONE',  ( 8.309058582316795949, -22.74294823697954016, 2.828734674606448785 ) ) ;
#19812=CARTESIAN_POINT ( 'NONE',  ( 6.815941417683176518, -20.79840458871654363, 4.773278322869464851 ) ) ;
#19813=CARTESIAN_POINT ( 'NONE',  ( -10.84030858231679240, -22.67418626127525982, 5.270995438708342640 ) ) ;
#19815=CARTESIAN_POINT ( 'NONE',  ( 13.13728495444130751, 4.870390199291127153, 6.548325014280736767 ) ) ;
#19816=CARTESIAN_POINT ( 'NONE',  ( 12.62966097655984754, -19.26462068372267566, 4.756751955311774083 ) ) ;
#19825=CARTESIAN_POINT ( 'NONE',  ( 1.716273078461125090, -9.866787073280026021, 2.373124017006284170 ) ) ;
#19829=CARTESIAN_POINT ( 'NONE',  ( 12.87788743559736027, -20.60791989766740073, 3.516327362592114092 ) ) ;
#19830=CARTESIAN_POINT ( 'NONE',  ( -1.824488249492779879, -9.124319963227819130, 2.375058613629473570 ) ) ;
#19831=CARTESIAN_POINT ( 'NONE',  ( -8.496558582316794173, -22.05068747287764452, 1.749999999999998446 ) ) ;
#19832=CARTESIAN_POINT ( 'NONE',  ( -3.506783328160878010, -9.991161114504492957, 2.040295720924476530 ) ) ;
#19834=CARTESIAN_POINT ( 'NONE',  ( -13.37680511754115287, -19.40884156416817774, 4.692171866446762429 ) ) ;
#19835=CARTESIAN_POINT ( 'NONE',  ( -5.590308582316794173, -21.32581373872472597, 1.729004561291657582 ) ) ;
#19837=CARTESIAN_POINT ( 'NONE',  ( -4.003441417683176518, -22.05068747287765873, 5.250000000000000888 ) ) ;
#19839=CARTESIAN_POINT ( 'NONE',  ( 13.37499999999998224, -20.24999999999998934, 4.166666666666636765 ) ) ;
#19842=ORIENTED_EDGE ( 'NONE', *, *, #12222, .F. ) ;
#19845=CARTESIAN_POINT ( 'NONE',  ( -13.37883250981221472, -20.05645825448334563, 5.102688967256983510 ) ) ;
#19852=CARTESIAN_POINT ( 'NONE',  ( 3.379380450443691952, -10.24275229525297348, 2.854909362179569587 ) ) ;
#19853=CARTESIAN_POINT ( 'NONE',  ( -4.687312169500630787, -21.51559725698340131, 5.182386163300424009 ) ) ;
#19855=CARTESIAN_POINT ( 'NONE',  ( 12.65679946139692902, -19.39412719945235253, 6.251687395662565372 ) ) ;
#19857=CARTESIAN_POINT ( 'NONE',  ( 9.534691417683177406, -20.97900456129164581, 3.136473910504570917 ) ) ;
#19859=CARTESIAN_POINT ( 'NONE',  ( -4.378441417683176518, -22.99999999999999645, 3.449312527122335048 ) ) ;
#19860=CARTESIAN_POINT ( 'NONE',  ( -9.809058582316795949, -23.80360840875935935, 1.768074502826626260 ) ) ;
#19863=CARTESIAN_POINT ( 'NONE',  ( 12.62499999999998401, -19.49999999999998934, 2.439580858552613751 ) ) ;
#19864=CARTESIAN_POINT ( 'NONE',  ( -13.02818618459764188, 0.1109023222084986743, 5.923858176248589125 ) ) ;
#19874=CARTESIAN_POINT ( 'NONE',  ( -1.548630333695928618, -8.364917468222230923, 1.622643865078341907 ) ) ;
#19878=CARTESIAN_POINT ( 'NONE',  ( 13.12529380813666435, 5.014837310896125722, 5.033295791462342628 ) ) ;
#19880=CARTESIAN_POINT ( 'NONE',  ( 5.777808582316795949, -19.52099543870833642, 2.413778621189609286 ) ) ;
#19881=CARTESIAN_POINT ( 'NONE',  ( -12.83635126708105823, -9.576761012430582198, 5.715524842913705328 ) ) ;
#19882=CARTESIAN_POINT ( 'NONE',  ( -4.659691417683177406, -22.98484643305507191, 0.9790045612916508100 ) ) ;
#19886=CARTESIAN_POINT ( 'NONE',  ( -13.56222317325195093, -11.54522975075300728, 6.408692769197242178 ) ) ;
#19887=CARTESIAN_POINT ( 'NONE',  ( 4.840308582316795061, -22.36352608949544418, 4.520995438708343528 ) ) ;
#19891=CARTESIAN_POINT ( 'NONE',  ( 13.87454419214980739, 4.976981703567351367, 5.131312659523921127 ) ) ;
#19898=CARTESIAN_POINT ( 'NONE',  ( 13.39107665282975645, -19.43812903209671461, 5.476542851584349947 ) ) ;
#19900=CARTESIAN_POINT ( 'NONE',  ( 1.743623630681728542, -9.116095536440919744, 2.372946416531167557 ) ) ;
#19904=CARTESIAN_POINT ( 'NONE',  ( -13.12529397354238192, 5.014845663890295846, 4.583333333333296622 ) ) ;
#19907=CARTESIAN_POINT ( 'NONE',  ( 12.24655858231679240, -21.94931252712234482, 5.250000000000000888 ) ) ;
#19908=CARTESIAN_POINT ( 'NONE',  ( -13.40787921250184311, -19.33959976865745389, 6.241060671539915283 ) ) ;
#19911=CARTESIAN_POINT ( 'NONE',  ( 11.40280858231679595, -22.46490103525074034, 2.520995438708341307 ) ) ;
#19912=CARTESIAN_POINT ( 'NONE',  ( 10.28469141768318096, -23.77099543870834353, 4.174186261275252718 ) ) ;
#19913=CARTESIAN_POINT ( 'NONE',  ( -11.49655858231679417, -22.05068747287764452, 1.749999999999998446 ) ) ;
#19915=CARTESIAN_POINT ( 'NONE',  ( 13.11644927503132330, 3.818188389080370282, 6.753616037489316604 ) ) ;
#19916=CARTESIAN_POINT ( 'NONE',  ( 12.62868952012632207, -19.31367923361656480, 4.748088538831167327 ) ) ;
#19922=FACE_OUTER_BOUND ( 'NONE', #2225, .T. ) ;
#19925=CARTESIAN_POINT ( 'NONE',  ( 1.619022621591187150, -9.114917468222230923, 2.372643865078341019 ) ) ;
#19929=CARTESIAN_POINT ( 'NONE',  ( -2.601332995093193379, -9.970398767539743190, 2.592349323443654097 ) ) ;
#19930=CARTESIAN_POINT ( 'NONE',  ( -5.871558582316794173, -20.24999999999999289, 3.449312527122348371 ) ) ;
#19931=CARTESIAN_POINT ( 'NONE',  ( -3.436477319925839602, -9.631595465688135960, 1.947952079262935676 ) ) ;
#19933=CARTESIAN_POINT ( 'NONE',  ( -13.37893135632597819, -19.30146650553847465, 4.738802066438188909 ) ) ;
#19935=CARTESIAN_POINT ( 'NONE',  ( 12.15280858231679950, -20.91377862118960351, 5.979004561291660913 ) ) ;
#19936=CARTESIAN_POINT ( 'NONE',  ( -11.31594141768317741, -21.32873467460645145, 4.242948236979555254 ) ) ;
#19938=CARTESIAN_POINT ( 'NONE',  ( 13.84264281492353987, 3.365962153638767607, 5.979325532956542233 ) ) ;
#19939=CARTESIAN_POINT ( 'NONE',  ( -2.693754455098655409, -10.04853567022903782, 2.237415670251142519 ) ) ;
#19945=CARTESIAN_POINT ( 'NONE',  ( -13.37500015856764435, -20.24999199233421265, 4.532157119432948633 ) ) ;
#19950=CARTESIAN_POINT ( 'NONE',  ( 3.451187703687236041, -10.75258211228477734, 2.985843844067104680 ) ) ;
#19951=CARTESIAN_POINT ( 'NONE',  ( -6.434058582316794173, -23.20159541128345992, 4.773278322869455970 ) ) ;
#19952=CARTESIAN_POINT ( 'NONE',  ( 13.87486364728600208, 4.243114187942282456, 6.725269602253773016 ) ) ;
#19954=CARTESIAN_POINT ( 'NONE',  ( 4.190941417683176518, -23.27327832286946219, 4.701595411283453707 ) ) ;
#19956=CARTESIAN_POINT ( 'NONE',  ( -4.190941417683176518, -22.74294823697955081, 4.171265325393542334 ) ) ;
#19957=CARTESIAN_POINT ( 'NONE',  ( -10.56594141768317741, -23.73192549717336064, 1.696391591240623331 ) ) ;
#19959=CARTESIAN_POINT ( 'NONE',  ( 12.64917329730235096, -18.27924848622803466, 4.778345106674467324 ) ) ;
#19960=CARTESIAN_POINT ( 'NONE',  ( -13.11145189917479392, 4.315820908324673688, 5.961432613039677086 ) ) ;
#19972=CARTESIAN_POINT ( 'NONE',  ( -1.619022621591187150, -9.114917468222230923, 1.622643865078341463 ) ) ;
#19977=CARTESIAN_POINT ( 'NONE',  ( 6.621558582316796837, -24.50000000000000000, 3.550687472877651629 ) ) ;
#19978=CARTESIAN_POINT ( 'NONE',  ( -13.10252221513633941, 3.864871864382954048, 6.004587342915129966 ) ) ;
#19979=CARTESIAN_POINT ( 'NONE',  ( -6.815941417683177406, -20.26807450282663225, 5.303608408759377113 ) ) ;
#19981=CARTESIAN_POINT ( 'NONE',  ( 11.87155858231679417, -20.24999999999999289, 3.449312527122348371 ) ) ;
#19983=CARTESIAN_POINT ( 'NONE',  ( -13.42074492158312715, -18.68988146005270679, 6.255046935864005064 ) ) ;
#19984=CARTESIAN_POINT ( 'NONE',  ( 12.34030858231679240, -22.67418626127525982, 5.270995438708342640 ) ) ;
#19988=CARTESIAN_POINT ( 'NONE',  ( 13.47096266223369376, -15.40388555723029462, 5.575679699623145247 ) ) ;
#19999=CARTESIAN_POINT ( 'NONE',  ( 3.422464802389687311, -10.54865018547243061, 2.933470051312085936 ) ) ;
#20001=CARTESIAN_POINT ( 'NONE',  ( -13.12529418130016445, 5.014856155665242454, 4.958178834604180629 ) ) ;
#20005=CARTESIAN_POINT ( 'NONE',  ( -13.82120031190154208, 1.533115751011936867, 6.689942769197355865 ) ) ;
#20009=CARTESIAN_POINT ( 'NONE',  ( 5.309058582316795949, -22.74294823697954016, 2.828734674606448785 ) ) ;
#20010=CARTESIAN_POINT ( 'NONE',  ( 4.659691417683178294, -22.67418626127524917, 1.729004561291651809 ) ) ;
#20011=CARTESIAN_POINT ( 'NONE',  ( -10.27780858231679417, -20.27099543870833642, 2.724438792969431589 ) ) ;
#20013=CARTESIAN_POINT ( 'NONE',  ( 13.11704875914858270, 3.848462337001107070, 6.754267079155989784 ) ) ;
#20014=CARTESIAN_POINT ( 'NONE',  ( 13.07840392524817474, 3.396898225032857432, 5.244490940007585422 ) ) ;
#20027=CARTESIAN_POINT ( 'NONE',  ( 1.791727654783324741, -9.894249715907907472, 2.380176972254574697 ) ) ;
#20032=CARTESIAN_POINT ( 'NONE',  ( -9.621558582316795949, -24.50000000000000000, 3.550687472877651629 ) ) ;
#20033=CARTESIAN_POINT ( 'NONE',  ( -2.012076196476103362, -9.160103213191565175, 1.634248467062433541 ) ) ;
#20036=CARTESIAN_POINT ( 'NONE',  ( -13.09560260347216953, 4.265431475339161338, 5.020858537328734883 ) ) ;
#20037=CARTESIAN_POINT ( 'NONE',  ( -8.309058582316792396, -23.27327832286945153, 2.298404588716537411 ) ) ;
#20038=CARTESIAN_POINT ( 'NONE',  ( 9.440941417683177406, -20.19639159124061933, 1.768074502826635586 ) ) ;
#20039=CARTESIAN_POINT ( 'NONE',  ( -8.597191417683177406, -22.46490103525075810, 4.479004561291653808 ) ) ;
#20042=CARTESIAN_POINT ( 'NONE',  ( 13.85343352903393388, 3.910893216212274925, 5.991044282956552891 ) ) ;
#20049=CARTESIAN_POINT ( 'NONE',  ( -13.80667376788930056, 1.549525278393783179, 5.940263032956496048 ) ) ;
#20056=CARTESIAN_POINT ( 'NONE',  ( 3.270401025279431995, -9.547343748290430199, 2.676314555138040063 ) ) ;
#20057=CARTESIAN_POINT ( 'NONE',  ( 2.693754455098655409, -10.14181605509423711, 1.874202551270839123 ) ) ;
#20060=CARTESIAN_POINT ( 'NONE',  ( 12.66144083004408571, -19.15973808277258073, 6.259475412489329038 ) ) ;
#20063=CARTESIAN_POINT ( 'NONE',  ( 4.097191417683176518, -22.77556120703057729, 5.229004561291655584 ) ) ;
#20065=CARTESIAN_POINT ( 'NONE',  ( -8.690941417683177406, -22.74294823697955081, 4.171265325393542334 ) ) ;
#20066=CARTESIAN_POINT ( 'NONE',  ( -11.69094141768317741, -23.80360840875937001, 5.231925497173365081 ) ) ;
#20068=CARTESIAN_POINT ( 'NONE',  ( 13.12529397354238192, 5.014845663890295846, 4.333333333333382775 ) ) ;
#20069=CARTESIAN_POINT ( 'NONE',  ( -12.64751377014909828, -19.11305460747000495, 5.510446717915143289 ) ) ;
#20079=CARTESIAN_POINT ( 'NONE',  ( -1.548630333695928396, -9.114917468222230923, 1.622643865078341463 ) ) ;
#20083=CARTESIAN_POINT ( 'NONE',  ( 5.496558582316795949, -22.05068747287764452, 0.9999999999999978906 ) ) ;
#20084=CARTESIAN_POINT ( 'NONE',  ( -12.68288333306630378, -17.32689168014509207, 5.548858176248425700 ) ) ;
#20086=CARTESIAN_POINT ( 'NONE',  ( -8.034691417683175629, -19.47900456129164581, 2.515153566944927199 ) ) ;
#20093=CARTESIAN_POINT ( 'NONE',  ( -13.37499999999998224, -20.99999999999991829, 4.333333333333343695 ) ) ;
#20094=CARTESIAN_POINT ( 'NONE',  ( 5.309058582316795949, -22.74294823697954016, 2.828734674606448785 ) ) ;
#20098=CARTESIAN_POINT ( 'NONE',  ( 13.37499999999998224, -20.99999999999998934, 4.166666666666637653 ) ) ;
#20104=CARTESIAN_POINT ( 'NONE',  ( -10.74655858231679417, -21.94931252712234482, 5.250000000000000888 ) ) ;
#20108=CARTESIAN_POINT ( 'NONE',  ( 1.407845757905374695, -8.364917468222230923, 1.622643865078341907 ) ) ;
#20110=CARTESIAN_POINT ( 'NONE',  ( -13.09543520949579865, 4.256978079540234106, 5.067654010725516578 ) ) ;
#20112=CARTESIAN_POINT ( 'NONE',  ( -13.37923893525309715, -20.78593376972237650, 5.366589449429977954 ) ) ;
#20114=DIRECTION ( 'NONE',  ( 0.000000000000000000, -0.000000000000000000, -1.000000000000000000 ) ) ;
#20115=CARTESIAN_POINT ( 'NONE',  ( 5.121558582316795061, -22.99999999999999645, 3.550687472877652073 ) ) ;
#20117=CARTESIAN_POINT ( 'NONE',  ( 5.315941417683176518, -20.79840458871654363, 4.773278322869464851 ) ) ;
#20118=CARTESIAN_POINT ( 'NONE',  ( -9.152808582316794173, -21.22443879296942626, 5.229004561291659137 ) ) ;
#20121=CARTESIAN_POINT ( 'NONE',  ( 13.08919463935856697, 3.941829287606363863, 5.256209690007596080 ) ) ;
#20129=CARTESIAN_POINT ( 'NONE',  ( -2.702705060698113115, -10.69015907548275379, 2.777197378435510622 ) ) ;
#20130=CARTESIAN_POINT ( 'NONE',  ( -13.43259567872942917, -17.34141822415733714, 5.534013032956523581 ) ) ;
#20133=CARTESIAN_POINT ( 'NONE',  ( 1.837882866761050282, -9.938290523052360825, 2.391487531332776140 ) ) ;
#20136=EDGE_CURVE ( 'NONE', #8942, #13028, #9011, .T. ) ;
#20138=CARTESIAN_POINT ( 'NONE',  ( -12.99655858231679595, -22.05068747287764452, 0.9999999999999978906 ) ) ;
#20139=CARTESIAN_POINT ( 'NONE',  ( -2.768424032093183662, -10.00067216410020166, 1.850123365707658785 ) ) ;
#20141=CARTESIAN_POINT ( 'NONE',  ( -13.37818000216760694, -19.33940989053615311, 4.728953261990445966 ) ) ;
#20143=CARTESIAN_POINT ( 'NONE',  ( 5.027808582316795949, -24.47900456129166358, 4.586221378810390270 ) ) ;
#20144=CARTESIAN_POINT ( 'NONE',  ( -12.44094141768317741, -21.25705176302044208, 2.828734674606458555 ) ) ;
#20146=CARTESIAN_POINT ( 'NONE',  ( 13.37515323800563039, -20.24226148071262799, 4.627790572011877934 ) ) ;
#20153=CARTESIAN_POINT ( 'NONE',  ( -13.84863765609603625, 3.668701632846259830, 5.985835949623216301 ) ) ;
#20154=CARTESIAN_POINT ( 'NONE',  ( 1.904508877737772998, -9.138371295333994837, 2.378667276417936627 ) ) ;
#20159=CARTESIAN_POINT ( 'NONE',  ( 3.365018999794965548, -10.14078633184679923, 2.828722465802024910 ) ) ;
#20163=CARTESIAN_POINT ( 'NONE',  ( 12.66383876651304874, -19.03864229108970463, 6.262079579155994224 ) ) ;
#20168=CARTESIAN_POINT ( 'NONE',  ( 3.974842109207561425, -21.82955800590261575, 5.256404853634145447 ) ) ;
#20170=CARTESIAN_POINT ( 'NONE',  ( -9.527808582316795949, -22.97900456129165647, 3.964901035250747885 ) ) ;
#20171=CARTESIAN_POINT ( 'NONE',  ( -8.878441417683177406, -24.50000000000000000, 3.449312527122335048 ) ) ;
#20173=CARTESIAN_POINT ( 'NONE',  ( 12.62499999999998401, -19.49999999999998934, 3.146526952850934755 ) ) ;
#20174=CARTESIAN_POINT ( 'NONE',  ( -13.12529397354238192, 5.014845663890295846, 4.833333333333344584 ) ) ;
#20180=CARTESIAN_POINT ( 'NONE',  ( 1.857501949683560971, -9.975525523312803955, 2.401050223243493154 ) ) ;
#20187=CARTESIAN_POINT ( 'NONE',  ( 0.000000000000000000, -9.864917468222230923, 1.622643865078341241 ) ) ;
#20189=DIRECTION ( 'NONE',  ( 0.1351665943404306014, -0.9596796555888912339, 0.2464649070825229438 ) ) ;
#20191=CARTESIAN_POINT ( 'NONE',  ( 9.815941417683177406, -20.26807450282663225, 5.303608408759377113 ) ) ;
#20192=CARTESIAN_POINT ( 'NONE',  ( -12.65410809543883985, -18.78004118034163739, 5.517608176248461227 ) ) ;
#20193=CARTESIAN_POINT ( 'NONE',  ( -6.159691417683175629, -22.98484643305507191, 0.9790045612916508100 ) ) ;
#20197=CARTESIAN_POINT ( 'NONE',  ( -13.84517967659089521, 2.744073667841084418, 6.715984435864265301 ) ) ;
#20198=CARTESIAN_POINT ( 'NONE',  ( 11.96530858231679595, -20.22900456129164937, 4.174186261275266929 ) ) ;
#20201=ORIENTED_EDGE ( 'NONE', *, *, #19216, .T. ) ;
#20202=CARTESIAN_POINT ( 'NONE',  ( 13.71569110726703045, -3.795099083046435506, 6.575359435862661250 ) ) ;
#20205=EDGE_CURVE ( 'NONE', #4517, #1847, #7623, .T. ) ;
#20208=CARTESIAN_POINT ( 'NONE',  ( -8.590308582316794173, -21.32581373872472597, 1.729004561291657582 ) ) ;
#20209=CARTESIAN_POINT ( 'NONE',  ( 13.87215786865436762, 4.856472367046606564, 5.506273593909547515 ) ) ;
#20211=CARTESIAN_POINT ( 'NONE',  ( 1.126276606324276619, -8.364917468222230923, 1.622643865078341907 ) ) ;
#20213=CARTESIAN_POINT ( 'NONE',  ( -13.08439876642066935, 3.699637704240349656, 5.251001356674258602 ) ) ;
#20215=CARTESIAN_POINT ( 'NONE',  ( -13.67732412376249052, -5.732631749971324631, 6.533692769198849781 ) ) ;
#20217=CARTESIAN_POINT ( 'NONE',  ( 4.687312169500634340, -21.70215802671379990, 4.455959925339818106 ) ) ;
#20218=CARTESIAN_POINT ( 'NONE',  ( 5.034691417683178294, -20.22900456129164581, 2.825813738724747726 ) ) ;
#20219=CARTESIAN_POINT ( 'NONE',  ( -8.309058582316792396, -23.27327832286945153, 2.298404588716537411 ) ) ;
#20220=ORIENTED_EDGE ( 'NONE', *, *, #20205, .T. ) ;
#20221=CARTESIAN_POINT ( 'NONE',  ( 13.09560269887985307, 4.265436293439658577, 4.973800642626965640 ) ) ;
#20227=CARTESIAN_POINT ( 'NONE',  ( -12.95145221759166354, -3.764163011652346569, 5.840524842913703552 ) ) ;
#20229=CARTESIAN_POINT ( 'NONE',  ( -2.579281110863027582, -9.822567596814183233, 2.554382554832406615 ) ) ;
#20230=CARTESIAN_POINT ( 'NONE',  ( -13.87470623115321899, 4.985164673244912414, 4.958488177337359026 ) ) ;
#20237=CARTESIAN_POINT ( 'NONE',  ( 0.000000000000000000, -9.114917468222230923, 2.372643865078340575 ) ) ;
#20238=CARTESIAN_POINT ( 'NONE',  ( -8.590308582316797725, -21.01515356694490322, 0.9790045612916562501 ) ) ;
#20239=CARTESIAN_POINT ( 'NONE',  ( -0.5631383031621635116, -8.364917468222230923, 1.622643865078341907 ) ) ;
#20241=CARTESIAN_POINT ( 'NONE',  ( -13.84501474873290938, 4.235744811019327649, 4.974109985360144037 ) ) ;
#20243=CARTESIAN_POINT ( 'NONE',  ( 12.15969141768317918, -22.98484643305507191, 0.9790045612916508100 ) ) ;
#20244=CARTESIAN_POINT ( 'NONE',  ( -9.628441417683177406, -20.99999999999999645, 3.550687472877664952 ) ) ;
#20246=CARTESIAN_POINT ( 'NONE',  ( 13.38795836133016870, -20.34560275282643005, 5.879540349057044146 ) ) ;
#20252=CARTESIAN_POINT ( 'NONE',  ( -13.87470602645761986, 4.985154336109792972, 4.333333333333379223 ) ) ;
#20254=CARTESIAN_POINT ( 'NONE',  ( 1.513434189748285696, -9.114917468222230923, 2.372643865078341019 ) ) ;
#20257=CARTESIAN_POINT ( 'NONE',  ( 2.693754455098655409, -10.04853567022903782, 2.237415670251142519 ) ) ;
#20259=CARTESIAN_POINT ( 'NONE',  ( 3.486710468562268961, -9.848741751643258269, 2.003719583429115492 ) ) ;
#20265=CARTESIAN_POINT ( 'NONE',  ( 13.12529397354238192, 5.014845663890295846, 3.000000000000000000 ) ) ;
#20266=CARTESIAN_POINT ( 'NONE',  ( 7.190941417683177406, -22.74294823697955081, 4.171265325393542334 ) ) ;
#20267=CARTESIAN_POINT ( 'NONE',  ( -13.08094078691552831, 2.775009739235173356, 5.981149842915306714 ) ) ;
#20269=CARTESIAN_POINT ( 'NONE',  ( -8.121558582316795949, -22.99999999999999645, 3.550687472877652073 ) ) ;
#20270=CARTESIAN_POINT ( 'NONE',  ( -7.659691417683177406, -22.98484643305507191, 0.9790045612916508100 ) ) ;
#20272=CARTESIAN_POINT ( 'NONE',  ( 12.62499999998404299, -19.49999999996810729, 2.793053905886972998 ) ) ;
#20273=DIRECTION ( 'NONE',  ( -0.000000000000000000, -0.000000000000000000, -1.000000000000000000 ) ) ;
#20278=CARTESIAN_POINT ( 'NONE',  ( 2.875042468481914248, -11.91375063635796039, 3.091440134965714126 ) ) ;
#20284=CARTESIAN_POINT ( 'NONE',  ( -2.088806020750596737, -10.42712783963456857, 1.767030719737609168 ) ) ;
#20288=CARTESIAN_POINT ( 'NONE',  ( 11.50344141768317741, -22.05068747287766229, 6.000000000000001776 ) ) ;
#20289=CARTESIAN_POINT ( 'NONE',  ( -13.10431844137356627, 3.955581289335645234, 6.006545679920360925 ) ) ;
#20291=CARTESIAN_POINT ( 'NONE',  ( -11.87844141768317563, -23.74999999999999645, 3.449312527122335492 ) ) ;
#20293=CARTESIAN_POINT ( 'NONE',  ( 12.71530858231679240, -23.77099543870833998, 2.825813738724734847 ) ) ;
#20295=CARTESIAN_POINT ( 'NONE',  ( -13.37505392270939986, -20.99727690317663686, 4.612442573673130930 ) ) ;
#20296=CARTESIAN_POINT ( 'NONE',  ( 11.59030858231679417, -21.32581373872472597, 1.729004561291657582 ) ) ;
#20298=ORIENTED_EDGE ( 'NONE', *, *, #20136, .T. ) ;
#20300=CARTESIAN_POINT ( 'NONE',  ( 13.40432071140796744, -19.51930407389869515, 6.223619713037471968 ) ) ;
#20305=CARTESIAN_POINT ( 'NONE',  ( -12.90280858231679773, -22.77556120703056308, 1.770995438708339975 ) ) ;
#20307=DIRECTION ( 'NONE',  ( 0.000000000000000000, -0.2487476929738665354, -0.9685683172808094987 ) ) ;
#20308=CARTESIAN_POINT ( 'NONE',  ( 1.948765222931501784, -9.143197003266354983, 1.629906614618163552 ) ) ;
#20309=AXIS2_PLACEMENT_3D ( 'NONE', #7842, #20612, #4804 ) ;
#20311=CARTESIAN_POINT ( 'NONE',  ( -13.37499994994395891, -19.50000252782794519, 4.474109982178703149 ) ) ;
#20312=CARTESIAN_POINT ( 'NONE',  ( 11.12155858231679417, -23.74999999999999645, 3.550687472877651629 ) ) ;
#20313=CARTESIAN_POINT ( 'NONE',  ( -13.41115317570721110, -19.17426462678482579, 6.244630269197427808 ) ) ;
#20316=CARTESIAN_POINT ( 'NONE',  ( 5.027808582316795949, -22.97900456129165647, 3.964901035250747885 ) ) ;
#20318=CARTESIAN_POINT ( 'NONE',  ( 9.815941417683177406, -21.32873467460645145, 4.242948236979555254 ) ) ;
#20319=CARTESIAN_POINT ( 'NONE',  ( -6.809058582316794173, -23.27327832286945153, 2.298404588716537411 ) ) ;
#20321=CARTESIAN_POINT ( 'NONE',  ( 13.09560264576187905, 4.265433610975056133, 4.916666666666649199 ) ) ;
#20322=CARTESIAN_POINT ( 'NONE',  ( -1.948765222931501784, -9.143197003266354983, 1.629906614618163552 ) ) ;
#20328=CARTESIAN_POINT ( 'NONE',  ( -13.10624331898488037, 4.052787608736739600, 6.006964772046813117 ) ) ;
#20329=CARTESIAN_POINT ( 'NONE',  ( -2.203959450683124377, -9.262433282444222371, 2.410528873095051594 ) ) ;
#20330=CARTESIAN_POINT ( 'NONE',  ( -13.87066368810231154, 4.781016249162736820, 5.617237349937618696 ) ) ;
#20335=( BOUNDED_CURVE ( )  B_SPLINE_CURVE ( 2, ( #11264, #14287, #14505, #3319, #17758, #9591, #3427, #4786, #1757, #12622, #8143, #3219, #15867, #15967, #7923, #12930, #183, #14190, #1856, #6671, #8034, #13042, #17542, #1651, #11171, #14402, #11074, #8240, #5098, #85, #6248, #20700, #9700, #19027, #6567, #1545, #19134, #4681, #9805, #19333, #19443, #16191, #14604, #279, #11479, #17859, #9904, #17443, #6363, #16285, #7827, #5405, #803, #2258, #10429, #11671, #15127, #11575, #11777, #393, #3834, #8644, #8338, #18169, #699, #15018, #16386, #10318, #10213, #13346, #13550, #5504, #7186, #8543, #19951, #16687, #19747, #8756, #6872, #590, #13449, #13239, #1956, #14716, #19638, #5295, #5609, #6776, #3624, #16580, #16488, #11981, #10008, #7085, #19853 ),
 .UNSPECIFIED., .F., .F. ) 
 B_SPLINE_CURVE_WITH_KNOTS ( ( 3, 2, 2, 2, 2, 2, 2, 2, 2, 2, 2, 2, 2, 2, 2, 2, 2, 2, 2, 2, 2, 2, 2, 2, 2, 2, 2, 2, 2, 2, 2, 2, 2, 2, 2, 2, 2, 2, 2, 2, 2, 2, 2, 2, 2, 2, 2, 3 ),
 ( 0.000000000000000000, 0.02083333333333333218, 0.04166666666666666435, 0.06250000000000000000, 0.08333333333333332871, 0.1041666666666666713, 0.1250000000000000000, 0.1458333333333333426, 0.1666666666666666574, 0.1875000000000000000, 0.2083333333333333426, 0.2291666666666666574, 0.2500000000000000000, 0.2708333333333333148, 0.2916666666666666852, 0.3124999999999999445, 0.3333333333333333148, 0.3541666666666666852, 0.3750000000000000000, 0.3958333333333333148, 0.4166666666666666852, 0.4375000000000000555, 0.4583333333333333148, 0.4791666666666666852, 0.5000000000000000000, 0.5208333333333333703, 0.5416666666666666297, 0.5625000000000000000, 0.5833333333333333703, 0.6041666666666666297, 0.6249999999999998890, 0.6458333333333333703, 0.6666666666666666297, 0.6875000000000000000, 0.7083333333333333703, 0.7291666666666666297, 0.7500000000000000000, 0.7708333333333333703, 0.7916666666666666297, 0.8125000000000000000, 0.8333333333333333703, 0.8541666666666666297, 0.8750000000000001110, 0.8958333333333333703, 0.9166666666666666297, 0.9375000000000000000, 0.9583333333333333703, 0.9650437087885355147 ),
 .UNSPECIFIED. ) 
 CURVE ( )  GEOMETRIC_REPRESENTATION_ITEM ( )  RATIONAL_B_SPLINE_CURVE ( ( 1.000000000000000000, 0.9238795325112867385, 1.000000000000000000, 0.9238795325112867385, 1.000000000000000000, 0.9238795325112867385, 1.000000000000000000, 0.9238795325112867385, 1.000000000000000000, 0.9238795325112867385, 1.000000000000000000, 0.9238795325112867385, 1.000000000000000000, 0.9238795325112867385, 1.000000000000000000, 0.9238795325112867385, 1.000000000000000000, 0.9238795325112867385, 1.000000000000000000, 0.9238795325112867385, 1.000000000000000000, 0.9238795325112867385, 1.000000000000000000, 0.9238795325112867385, 1.000000000000000000, 0.9238795325112867385, 1.000000000000000000, 0.9238795325112867385, 1.000000000000000000, 0.9238795325112867385, 1.000000000000000000, 0.9238795325112867385, 1.000000000000000000, 0.9238795325112867385, 1.000000000000000000, 0.9238795325112867385, 1.000000000000000000, 0.9238795325112867385, 1.000000000000000000, 0.9238795325112867385, 1.000000000000000000, 0.9238795325112867385, 1.000000000000000000, 0.9238795325112867385, 1.000000000000000000, 0.9238795325112867385, 1.000000000000000000, 0.9238795325112867385, 1.000000000000000000, 0.9238795325112867385, 1.000000000000000000, 0.9238795325112867385, 1.000000000000000000, 0.9238795325112867385, 1.000000000000000000, 0.9238795325112867385, 1.000000000000000000, 0.9238795325112867385, 1.000000000000000000, 0.9238795325112867385, 1.000000000000000000, 0.9238795325112867385, 1.000000000000000000, 0.9238795325112867385, 1.000000000000000000, 0.9238795325112867385, 1.000000000000000000, 0.9238795325112867385, 1.000000000000000000, 0.9238795325112867385, 1.000000000000000000, 0.9238795325112867385, 1.000000000000000000, 0.9238795325112867385, 1.000000000000000000, 0.9238795325112867385, 1.000000000000000000, 0.9238795325112867385, 1.000000000000000000, 0.9238795325112867385, 1.000000000000000000, 0.9238795325112867385, 1.000000000000000000, 0.9238795325112867385, 1.000000000000000000, 0.9238795325112867385, 1.000000000000000000, 0.9238795325112867385, 1.000000000000000000, 0.9238795325112867385, 1.000000000000000000, 0.9238795325112867385, 1.000000000000000000, 0.9754817479996107377, 0.9667580569362973497 ) ) 
 REPRESENTATION_ITEM ( '' )  );
#20337=CARTESIAN_POINT ( 'NONE',  ( -7.934058582316796837, -23.73192549717337130, 5.303608408759367343 ) ) ;
#20338=CARTESIAN_POINT ( 'NONE',  ( 0.000000000000000000, -9.114917468222230923, 1.622643865078341019 ) ) ;
#20340=CARTESIAN_POINT ( 'NONE',  ( -13.84501469867365131, 4.235742283194553259, 3.333333333332063386 ) ) ;
#20342=CARTESIAN_POINT ( 'NONE',  ( 12.25344141768317741, -21.94931252712233061, 0.9999999999999978906 ) ) ;
#20343=CARTESIAN_POINT ( 'NONE',  ( -13.37155858231679595, -20.99999999999999645, 3.449312527122348371 ) ) ;
#20345=CARTESIAN_POINT ( 'NONE',  ( 13.87467358130843387, 4.983515856073828409, 5.065827972856573602 ) ) ;
#20349=ORIENTED_EDGE ( 'NONE', *, *, #7997, .T. ) ;
#20355=EDGE_CURVE ( 'NONE', #8228, #10614, #8537, .T. ) ;
#20357=CARTESIAN_POINT ( 'NONE',  ( 2.436080212393455735, -9.483920418190111334, 2.467411194204634839 ) ) ;
#20363=CARTESIAN_POINT ( 'NONE',  ( 2.012076196476103362, -9.160103213191565175, 1.634248467062433541 ) ) ;
#20366=CARTESIAN_POINT ( 'NONE',  ( 13.10821839766814279, 4.152529082241303904, 5.997503362667785609 ) ) ;
#20371=CARTESIAN_POINT ( 'NONE',  ( 4.940941417683177406, -21.25705176302044208, 2.828734674606458555 ) ) ;
#20372=CARTESIAN_POINT ( 'NONE',  ( -13.12529397354238192, 5.014845663890295846, 4.166666666666765551 ) ) ;
#20373=CARTESIAN_POINT ( 'NONE',  ( -7.840308582316795949, -22.36352608949544418, 4.520995438708343528 ) ) ;
#20375=CARTESIAN_POINT ( 'NONE',  ( -7.472191417683177406, -24.47900456129165292, 2.413778621189595963 ) ) ;
#20377=CARTESIAN_POINT ( 'NONE',  ( 13.37500003877585186, -19.49999804181952712, 4.520055687292853008 ) ) ;
#20382=CARTESIAN_POINT ( 'NONE',  ( 2.602174906157317835, -9.976397331638239052, 2.593889103792902606 ) ) ;
#20392=CARTESIAN_POINT ( 'NONE',  ( -1.797685059409938280, -9.880079706704160358, 1.626537830816663588 ) ) ;
#20396=CARTESIAN_POINT ( 'NONE',  ( 4.472191417683178294, -24.47900456129165292, 2.413778621189595963 ) ) ;
#20398=CARTESIAN_POINT ( 'NONE',  ( -12.34719141768317563, -21.22443879296941915, 1.770995438708345748 ) ) ;
#20401=CARTESIAN_POINT ( 'NONE',  ( 5.121558582316794173, -23.74999999999999645, 3.550687472877651629 ) ) ;
#20403=CARTESIAN_POINT ( 'NONE',  ( -12.62608183053121458, -20.94536755816881168, 4.949360998036265613 ) ) ;
#20404=ORIENTED_EDGE ( 'NONE', *, *, #2791, .T. ) ;
#20406=CARTESIAN_POINT ( 'NONE',  ( 5.309058582316794173, -23.27327832286945153, 2.298404588716537411 ) ) ;
#20410=CARTESIAN_POINT ( 'NONE',  ( 13.37500027835944039, -20.99998594284889464, 4.544258551573043370 ) ) ;
#20417=CARTESIAN_POINT ( 'NONE',  ( -11.30905858231679417, -23.27327832286945153, 2.298404588716537411 ) ) ;
#20419=CARTESIAN_POINT ( 'NONE',  ( -4.687312169500630787, -21.51559725698340131, 5.182386163300424009 ) ) ;
#20421=CARTESIAN_POINT ( 'NONE',  ( 0.9854920305337622199, -8.364917468222230923, 1.622643865078341907 ) ) ;
#20426=CARTESIAN_POINT ( 'NONE',  ( -13.09494140422671471, 4.232040913449062636, 5.131376921800749003 ) ) ;
#20427=CARTESIAN_POINT ( 'NONE',  ( 5.496558582316794173, -22.05068747287764452, 1.749999999999998446 ) ) ;
#20428=CARTESIAN_POINT ( 'NONE',  ( -12.63806878948643231, -20.34002613093225520, 5.891296472647073124 ) ) ;
#20432=CARTESIAN_POINT ( 'NONE',  ( 6.434058582316796837, -22.67126532539354855, 4.242948236979545484 ) ) ;
#20433=CARTESIAN_POINT ( 'NONE',  ( 11.69094141768317741, -22.74294823697955081, 4.171265325393542334 ) ) ;
#20434=CARTESIAN_POINT ( 'NONE',  ( -4.934058582316793284, -23.20159541128345992, 4.773278322869455970 ) ) ;
#20436=CARTESIAN_POINT ( 'NONE',  ( 13.09560264576187905, 4.265433610975056133, 4.166666666666765551 ) ) ;
#20444=CARTESIAN_POINT ( 'NONE',  ( -12.64131715375063258, -19.42598373559290792, 5.491151580003103660 ) ) ;
#20445=CARTESIAN_POINT ( 'NONE',  ( -3.034277558025862298, -9.029550313327863620, 2.543334857076493094 ) ) ;
#20446=CARTESIAN_POINT ( 'NONE',  ( -13.87454419214980739, 4.976981703567351367, 5.131312659523921127 ) ) ;
#20452=CARTESIAN_POINT ( 'NONE',  ( -11.12155858231679595, -24.50000000000000000, 3.550687472877651629 ) ) ;
#20453=CARTESIAN_POINT ( 'NONE',  ( -2.309828811027716977, -9.292785183284841821, 1.668323847571005603 ) ) ;
#20455=CARTESIAN_POINT ( 'NONE',  ( -13.84402619238587206, 4.185822715484293077, 5.150938132831436533 ) ) ;
#20457=CARTESIAN_POINT ( 'NONE',  ( 5.215308582316795949, -24.52099543870834708, 2.515153566944913432 ) ) ;
#20458=CARTESIAN_POINT ( 'NONE',  ( -12.34030858231679773, -22.36352608949544418, 4.520995438708343528 ) ) ;
#20460=CARTESIAN_POINT ( 'NONE',  ( 13.37500000000002132, -21.00000000000274269, 4.083333333315724012 ) ) ;
#20466=CARTESIAN_POINT ( 'NONE',  ( -13.86106797245302147, 4.296432608878145487, 5.947261916831099171 ) ) ;
#20469=CARTESIAN_POINT ( 'NONE',  ( 1.797604806073912709, -9.120796646272857799, 2.374153755450133740 ) ) ;
#20471=CARTESIAN_POINT ( 'NONE',  ( -4.121804964265448845, -21.67354536559615497, 4.877507451124815319 ) ) ;
#20473=( BOUNDED_SURFACE ( )  B_SPLINE_SURFACE ( 3, 3, ( 
 ( #11348, #19422, #6231, #1626, #1737, #14486, #8220, #6449, #19003, #6338, #5079, #12710, #12813, #3200, #17624, #4659, #9572, #15945, #14583, #9785, #1525, #3294, #11150, #6647, #11051, #17740, #19112, #8007, #17424, #16171, #11455, #258, #4765, #16064, #8119, #12910, #3404, #373, #14892, #5485 ),
 ( #7063, #2341, #10093, #8735, #18250, #571, #10293, #1933, #16562, #8429, #5175, #11651, #9883, #17934, #11858, #11554, #16468, #13125, #8625, #475, #2237, #3913, #2141, #18042, #3603, #6849, #6951, #19617, #9983, #16663, #3715, #16365, #19522, #11758, #13322, #15103, #780, #8523, #14796, #2043 ),
 ( #7166, #19722, #13219, #5275, #5383, #18149, #3814, #11959, #6756, #10192, #14994, #19832, #675, #13426, #3504, #13529, #19931, #5588, #16265, #8316, #14691, #4222, #13625, #10821, #4019, #16874, #15512, #10602, #16976, #880, #12170, #1294, #2444, #15412, #13735, #18558, #7673, #20239, #9239, #18772 ),
 ( #15303, #14043, #8932, #2653, #9040, #5897, #10404, #1095, #7475, #2864, #4437, #12070, #13834, #20139, #15611, #16775, #7573, #2544, #5799, #8836, #17186, #20453, #6110, #20033, #18355, #12267, #13935, #7264, #18661, #10712, #15204, #4329, #5695, #18460, #17086, #2764, #4123, #9142, #1194, #20338 ),
 ( #10504, #6002, #982, #7371, #12377, #11023, #9649, #19081, #4738, #15718, #6306, #16142, #17281, #9548, #7880, #12678, #1809, #14350, #3378, #12886, #8094, #12785, #8194, #33, #4942, #6205, #18873, #14560, #14459, #3271, #17392, #4534, #16033, #1597, #11322, #17494, #14240, #9450, #2966, #11124 ),
 ( #19289, #9759, #17707, #7784, #233, #20647, #139, #1402, #3174, #4841, #10919, #15919, #9342, #12480, #7976, #19187, #14147, #6422, #11222, #17598, #12574, #6523, #1710, #20554, #18975, #4629, #3075, #15821, #1499, #648, #3686, #13404, #5052, #19694, #11529, #8291, #14772, #12992, #345, #14968 ),
 ( #6924, #2215, #13097, #449, #19810, #14665, #10070, #14870, #16341, #5358, #7036, #2015, #16445, #11735, #6827, #11836, #2118, #3889, #2315, #8705, #13197, #6729, #19499, #5152, #8500, #5464, #19594, #17910, #8405, #5248, #11626, #546, #15076, #9856, #9958, #16241, #8598, #13294, #18128, #6622 ) ),
 .UNSPECIFIED., .T., .F., .T. ) 
 B_SPLINE_SURFACE_WITH_KNOTS ( ( 4, 3, 4 ),
 ( 4, 2, 2, 2, 2, 2, 2, 2, 2, 2, 2, 2, 2, 2, 2, 2, 2, 2, 2, 4 ),
 ( 0.000000000000000000, 0.5000000000000000000, 1.000000000000000000 ),
 ( 0.000000000000000000, 0.3100443560520446118, 0.4650665340780669177, 0.5425776230910780429, 0.5813331675975836887, 0.6007109398508364562, 0.6200887121040892236, 0.6309950902025724950, 0.6419014683010558775, 0.6637142244980225314, 0.7073397368919559502, 0.7509652492858893691, 0.7727780054828560230, 0.7836843835813394055, 0.7945907616798226769, 0.8074288390748337596, 0.8202669164698448423, 0.8459430712598670077, 0.8972953808399113385, 1.000000000000000000 ),
 .UNSPECIFIED. ) 
 GEOMETRIC_REPRESENTATION_ITEM ( )  RATIONAL_B_SPLINE_SURFACE ( (
 ( 1.000000000000000000, 1.000000000000000000, 1.000000000000000000, 1.000000000000000000, 1.000000000000000000, 1.000000000000000000, 1.000000000000000000, 1.000000000000000000, 1.000000000000000000, 1.000000000000000000, 1.000000000000000000, 1.000000000000000000, 1.000000000000000000, 1.000000000000000000, 1.000000000000000000, 1.000000000000000000, 1.000000000000000000, 1.000000000000000000, 1.000000000000000000, 1.000000000000000000, 1.000000000000000000, 1.000000000000000000, 1.000000000000000000, 1.000000000000000000, 1.000000000000000000, 1.000000000000000000, 1.000000000000000000, 1.000000000000000000, 1.000000000000000000, 1.000000000000000000, 1.000000000000000000, 1.000000000000000000, 1.000000000000000000, 1.000000000000000000, 1.000000000000000000, 1.000000000000000000, 1.000000000000000000, 1.000000000000000000, 1.000000000000000000, 1.000000000000000000),
 ( 0.3333333333333333703, 0.3333333333333333703, 0.3333333333333333703, 0.3333333333333333703, 0.3333333333333333703, 0.3333333333333333703, 0.3333333333333333703, 0.3333333333333333703, 0.3333333333333333703, 0.3333333333333333703, 0.3333333333333333703, 0.3333333333333333703, 0.3333333333333333703, 0.3333333333333333703, 0.3333333333333333703, 0.3333333333333333703, 0.3333333333333333703, 0.3333333333333333703, 0.3333333333333333703, 0.3333333333333333703, 0.3333333333333333703, 0.3333333333333333703, 0.3333333333333333703, 0.3333333333333333703, 0.3333333333333333703, 0.3333333333333333703, 0.3333333333333333703, 0.3333333333333333703, 0.3333333333333333703, 0.3333333333333333703, 0.3333333333333333703, 0.3333333333333333703, 0.3333333333333333703, 0.3333333333333333703, 0.3333333333333333703, 0.3333333333333333703, 0.3333333333333333703, 0.3333333333333333703, 0.3333333333333333703, 0.3333333333333333703),
 ( 0.3333333333333333703, 0.3333333333333333703, 0.3333333333333333703, 0.3333333333333333703, 0.3333333333333333703, 0.3333333333333333703, 0.3333333333333333703, 0.3333333333333333703, 0.3333333333333333703, 0.3333333333333333703, 0.3333333333333333703, 0.3333333333333333703, 0.3333333333333333703, 0.3333333333333333703, 0.3333333333333333703, 0.3333333333333333703, 0.3333333333333333703, 0.3333333333333333703, 0.3333333333333333703, 0.3333333333333333703, 0.3333333333333333703, 0.3333333333333333703, 0.3333333333333333703, 0.3333333333333333703, 0.3333333333333333703, 0.3333333333333333703, 0.3333333333333333703, 0.3333333333333333703, 0.3333333333333333703, 0.3333333333333333703, 0.3333333333333333703, 0.3333333333333333703, 0.3333333333333333703, 0.3333333333333333703, 0.3333333333333333703, 0.3333333333333333703, 0.3333333333333333703, 0.3333333333333333703, 0.3333333333333333703, 0.3333333333333333703),
 ( 1.000000000000000000, 1.000000000000000000, 1.000000000000000000, 1.000000000000000000, 1.000000000000000000, 1.000000000000000000, 1.000000000000000000, 1.000000000000000000, 1.000000000000000000, 1.000000000000000000, 1.000000000000000000, 1.000000000000000000, 1.000000000000000000, 1.000000000000000000, 1.000000000000000000, 1.000000000000000000, 1.000000000000000000, 1.000000000000000000, 1.000000000000000000, 1.000000000000000000, 1.000000000000000000, 1.000000000000000000, 1.000000000000000000, 1.000000000000000000, 1.000000000000000000, 1.000000000000000000, 1.000000000000000000, 1.000000000000000000, 1.000000000000000000, 1.000000000000000000, 1.000000000000000000, 1.000000000000000000, 1.000000000000000000, 1.000000000000000000, 1.000000000000000000, 1.000000000000000000, 1.000000000000000000, 1.000000000000000000, 1.000000000000000000, 1.000000000000000000),
 ( 0.3333333333333333703, 0.3333333333333333703, 0.3333333333333333703, 0.3333333333333333703, 0.3333333333333333703, 0.3333333333333333703, 0.3333333333333333703, 0.3333333333333333703, 0.3333333333333333703, 0.3333333333333333703, 0.3333333333333333703, 0.3333333333333333703, 0.3333333333333333703, 0.3333333333333333703, 0.3333333333333333703, 0.3333333333333333703, 0.3333333333333333703, 0.3333333333333333703, 0.3333333333333333703, 0.3333333333333333703, 0.3333333333333333703, 0.3333333333333333703, 0.3333333333333333703, 0.3333333333333333703, 0.3333333333333333703, 0.3333333333333333703, 0.3333333333333333703, 0.3333333333333333703, 0.3333333333333333703, 0.3333333333333333703, 0.3333333333333333703, 0.3333333333333333703, 0.3333333333333333703, 0.3333333333333333703, 0.3333333333333333703, 0.3333333333333333703, 0.3333333333333333703, 0.3333333333333333703, 0.3333333333333333703, 0.3333333333333333703),
 ( 0.3333333333333333703, 0.3333333333333333703, 0.3333333333333333703, 0.3333333333333333703, 0.3333333333333333703, 0.3333333333333333703, 0.3333333333333333703, 0.3333333333333333703, 0.3333333333333333703, 0.3333333333333333703, 0.3333333333333333703, 0.3333333333333333703, 0.3333333333333333703, 0.3333333333333333703, 0.3333333333333333703, 0.3333333333333333703, 0.3333333333333333703, 0.3333333333333333703, 0.3333333333333333703, 0.3333333333333333703, 0.3333333333333333703, 0.3333333333333333703, 0.3333333333333333703, 0.3333333333333333703, 0.3333333333333333703, 0.3333333333333333703, 0.3333333333333333703, 0.3333333333333333703, 0.3333333333333333703, 0.3333333333333333703, 0.3333333333333333703, 0.3333333333333333703, 0.3333333333333333703, 0.3333333333333333703, 0.3333333333333333703, 0.3333333333333333703, 0.3333333333333333703, 0.3333333333333333703, 0.3333333333333333703, 0.3333333333333333703),
 ( 1.000000000000000000, 1.000000000000000000, 1.000000000000000000, 1.000000000000000000, 1.000000000000000000, 1.000000000000000000, 1.000000000000000000, 1.000000000000000000, 1.000000000000000000, 1.000000000000000000, 1.000000000000000000, 1.000000000000000000, 1.000000000000000000, 1.000000000000000000, 1.000000000000000000, 1.000000000000000000, 1.000000000000000000, 1.000000000000000000, 1.000000000000000000, 1.000000000000000000, 1.000000000000000000, 1.000000000000000000, 1.000000000000000000, 1.000000000000000000, 1.000000000000000000, 1.000000000000000000, 1.000000000000000000, 1.000000000000000000, 1.000000000000000000, 1.000000000000000000, 1.000000000000000000, 1.000000000000000000, 1.000000000000000000, 1.000000000000000000, 1.000000000000000000, 1.000000000000000000, 1.000000000000000000, 1.000000000000000000, 1.000000000000000000, 1.000000000000000000) ) ) 
 REPRESENTATION_ITEM ( '' )  SURFACE ( )  );
#20475=CARTESIAN_POINT ( 'NONE',  ( 2.916276642307554123, -11.05036367517186058, 2.119705115445599475 ) ) ;
#20477=CARTESIAN_POINT ( 'NONE',  ( 13.10372118337080849, 3.925419760224517329, 6.005889426248455010 ) ) ;
#20481=CARTESIAN_POINT ( 'NONE',  ( 5.409691417683178294, -21.63647391050456648, 4.520995438708348857 ) ) ;
#20482=CARTESIAN_POINT ( 'NONE',  ( -12.62499999999998401, -19.49999999999998934, 3.146526952850934755 ) ) ;
#20483=CARTESIAN_POINT ( 'NONE',  ( -10.74655858231679595, -21.94931252712234127, 4.499999999999999112 ) ) ;
#20485=CARTESIAN_POINT ( 'NONE',  ( -6.722191417683176518, -19.52099543870834353, 4.586221378810406257 ) ) ;
#20487=CARTESIAN_POINT ( 'NONE',  ( 13.07840392524817474, 3.396898225032857432, 5.244490940007585422 ) ) ;
#20493=CARTESIAN_POINT ( 'NONE',  ( 3.162271481458107658, -13.95306990448253437, 3.615178062515473911 ) ) ;
#20499=CARTESIAN_POINT ( 'NONE',  ( -2.282685604506861754, -11.80366834561962364, 2.120553820834011116 ) ) ;
#20505=CARTESIAN_POINT ( 'NONE',  ( 3.944195004867014909, -21.42722504787766624, 5.934029185143018914 ) ) ;
#20507=CARTESIAN_POINT ( 'NONE',  ( -7.097191417683177406, -22.77556120703057729, 5.229004561291655584 ) ) ;
#20509=CARTESIAN_POINT ( 'NONE',  ( 6.340308582316793284, -22.67418626127525982, 5.270995438708342640 ) ) ;
#20511=CARTESIAN_POINT ( 'NONE',  ( -12.73577686058281344, -15.40576854059989920, 6.340204579155907183 ) ) ;
#20513=CARTESIAN_POINT ( 'NONE',  ( 8.121558582316792396, -23.74999999999999645, 3.550687472877651629 ) ) ;
#20522=CARTESIAN_POINT ( 'NONE',  ( 12.63943061533661982, -19.52125392549825733, 5.470334935344855154 ) ) ;
#20525=CARTESIAN_POINT ( 'NONE',  ( 0.2815691515810352374, -8.364917468222230923, 1.622643865078524428 ) ) ;
#20527=CARTESIAN_POINT ( 'NONE',  ( -13.37500000000002132, -19.50000000000273559, 4.083333333315724012 ) ) ;
#20528=CARTESIAN_POINT ( 'NONE',  ( 10.18405858231679417, -20.79840458871652942, 2.226721677130544030 ) ) ;
#20529=CARTESIAN_POINT ( 'NONE',  ( -13.87144757537903494, 4.070602556641903291, 6.741633940066556363 ) ) ;
#20531=CARTESIAN_POINT ( 'NONE',  ( 6.621558582316794173, -23.74999999999999645, 3.550687472877651629 ) ) ;
#20533=CARTESIAN_POINT ( 'NONE',  ( 8.784691417683177406, -23.02099543870834353, 3.863526089495429972 ) ) ;
#20534=CARTESIAN_POINT ( 'NONE',  ( -11.97219141768317563, -23.72900456129164937, 2.724438792969417378 ) ) ;
#20536=CARTESIAN_POINT ( 'NONE',  ( 13.38269957179998038, -19.11117162410040038, 4.745921838382382241 ) ) ;
#20537=CARTESIAN_POINT ( 'NONE',  ( -1.337453470010121714, -9.114917468222230923, 1.622643865078341463 ) ) ;
#20539=UNCERTAINTY_MEASURE_WITH_UNIT (LENGTH_MEASURE( 1.000000000000000082E-05 ), #17046, 'distance_accuracy_value', 'NONE');
#20542=CARTESIAN_POINT ( 'NONE',  ( -12.64195242771744709, -19.39390240027112000, 5.496549442168085164 ) ) ;
#20543=EDGE_CURVE ( 'NONE', #14392, #8942, #9799, .T. ) ;
#20545=CARTESIAN_POINT ( 'NONE',  ( -1.655860418491166941, -9.114909740826840689, 2.372641880528837621 ) ) ;
#20546=CARTESIAN_POINT ( 'NONE',  ( -13.41820805991576826, -18.06799297425606454, 5.518388032956592859 ) ) ;
#20552=CARTESIAN_POINT ( 'NONE',  ( 13.15452713448031297, 5.741120291255121799, 5.290164123766007087 ) ) ;
#20553=CARTESIAN_POINT ( 'NONE',  ( -10.65969141768317741, -22.98484643305507191, 0.9790045612916508100 ) ) ;
#20554=CARTESIAN_POINT ( 'NONE',  ( -1.742625132518061504, -9.872369070458363538, 2.374557585393312298 ) ) ;
#20556=CARTESIAN_POINT ( 'NONE',  ( -13.83531008031826026, 3.745659056069631898, 5.237458296715707284 ) ) ;
#20558=CARTESIAN_POINT ( 'NONE',  ( 5.784691417683178294, -24.52099543870834708, 4.484846433055073689 ) ) ;
#20559=CARTESIAN_POINT ( 'NONE',  ( -5.690941417683177406, -22.74294823697955081, 4.171265325393542334 ) ) ;
#20561=CARTESIAN_POINT ( 'NONE',  ( 13.87470602645761986, 4.985154336109792972, 4.791666666666685614 ) ) ;
#20573=CARTESIAN_POINT ( 'NONE',  ( 3.187906586576829682, -9.105473976199601083, 1.812833570429532859 ) ) ;
#20579=CARTESIAN_POINT ( 'NONE',  ( 4.284691417683177406, -23.02099543870834353, 3.863526089495429972 ) ) ;
#20580=CARTESIAN_POINT ( 'NONE',  ( -13.12529397354238192, 5.014845663890295846, 4.791666666666685614 ) ) ;
#20581=CARTESIAN_POINT ( 'NONE',  ( -12.43405858231679595, -22.67126532539354855, 4.242948236979545484 ) ) ;
#20583=CARTESIAN_POINT ( 'NONE',  ( -4.472191417683178294, -24.47900456129165292, 2.413778621189595963 ) ) ;
#20585=CARTESIAN_POINT ( 'NONE',  ( 13.09560264576187905, 4.265433610975056133, 4.166666666666765551 ) ) ;
#20590=CARTESIAN_POINT ( 'NONE',  ( 2.583953725994688533, -9.847075946378776479, 2.560676788604062004 ) ) ;
#20593=CARTESIAN_POINT ( 'NONE',  ( 7.753441417683176518, -21.94931252712233061, 1.749999999999998446 ) ) ;
#20595=CARTESIAN_POINT ( 'NONE',  ( -0.2815691515810352930, -9.114917468222230923, 1.622643865078524206 ) ) ;
#20599=CARTESIAN_POINT ( 'NONE',  ( 7.003441417683177406, -22.05068747287766229, 6.000000000000001776 ) ) ;
#20601=CARTESIAN_POINT ( 'NONE',  ( -10.00344141768317563, -22.05068747287765873, 5.250000000000000888 ) ) ;
#20603=CARTESIAN_POINT ( 'NONE',  ( 8.121558582316792396, -23.74999999999999645, 3.550687472877651629 ) ) ;
#20605=CARTESIAN_POINT ( 'NONE',  ( -13.90439735423812273, 5.734566389025032684, 4.833333333333343695 ) ) ;
#20609=CARTESIAN_POINT ( 'NONE',  ( 7.090308582316794173, -21.32581373872472597, 1.729004561291657582 ) ) ;
#20610=CARTESIAN_POINT ( 'NONE',  ( -13.50000000000000178, 5.000000000000047962, 2.000000000000000000 ) ) ;
#20611=ORIENTED_EDGE ( 'NONE', *, *, #20656, .F. ) ;
#20612=DIRECTION ( 'NONE',  ( -0.1351665943404306014, -0.9596796555888912339, 0.2464649070825229438 ) ) ;
#20615=EDGE_CURVE ( 'NONE', #14392, #2288, #18378, .T. ) ;
#20618=CARTESIAN_POINT ( 'NONE',  ( -8.027808582316792396, -23.72900456129165647, 4.275561207030568411 ) ) ;
#20621=CARTESIAN_POINT ( 'NONE',  ( 1.337453470010121714, -9.864917468222230923, 1.622643865078341907 ) ) ;
#20623=CARTESIAN_POINT ( 'NONE',  ( -13.84090061271218985, 4.027980941966571748, 5.240332426532912535 ) ) ;
#20624=CARTESIAN_POINT ( 'NONE',  ( 4.687312169500632564, -21.51559725698341197, 5.182386163300427562 ) ) ;
#20625=CARTESIAN_POINT ( 'NONE',  ( -12.62527129584495000, -20.98629955982801576, 4.726243163759704657 ) ) ;
#20627=CARTESIAN_POINT ( 'NONE',  ( 5.402808582316794173, -22.77556120703056308, 1.770995438708339975 ) ) ;
#20629=CARTESIAN_POINT ( 'NONE',  ( 8.597191417683177406, -22.46490103525075810, 4.479004561291653808 ) ) ;
#20630=CARTESIAN_POINT ( 'NONE',  ( -11.78469141768317563, -23.77099543870834353, 4.174186261275251830 ) ) ;
#20632=CARTESIAN_POINT ( 'NONE',  ( 13.37939227869017600, -19.27818992614120575, 4.741950614318236390 ) ) ;
#20634=CARTESIAN_POINT ( 'NONE',  ( -2.012076196476103362, -9.160103213191565175, 1.634248467062433541 ) ) ;
#20639=CARTESIAN_POINT ( 'NONE',  ( -3.996922828336520794, -14.62728872172488437, 3.980945906412841850 ) ) ;
#20640=CARTESIAN_POINT ( 'NONE',  ( 1.337453470010121714, -9.114917468222230923, 2.372643865078341019 ) ) ;
#20643=CARTESIAN_POINT ( 'NONE',  ( -12.65650603190776025, -18.65894538865861563, 5.520212342915047365 ) ) ;
#20645=CARTESIAN_POINT ( 'NONE',  ( 13.15498530132288479, 5.764257716805535559, 4.916666666666649199 ) ) ;
#20646=CARTESIAN_POINT ( 'NONE',  ( -10.28469141768317741, -24.52099543870834708, 4.484846433055073689 ) ) ;
#20647=CARTESIAN_POINT ( 'NONE',  ( -2.011668220304084542, -11.03559989230542193, 2.673298498313999794 ) ) ;
#20649=CARTESIAN_POINT ( 'NONE',  ( -13.37499999999998579, -20.24999999999999289, 3.666666666666653640 ) ) ;
#20653=CARTESIAN_POINT ( 'NONE',  ( 7.003441417683177406, -22.05068747287766229, 6.000000000000001776 ) ) ;
#20654=CARTESIAN_POINT ( 'NONE',  ( -7.097191417683176518, -22.46490103525075810, 4.479004561291653808 ) ) ;
#20656=EDGE_CURVE ( 'NONE', #13542, #10698, #12014, .T. ) ;
#20657=CARTESIAN_POINT ( 'NONE',  ( 13.37499999999998401, -20.99999999999998934, 2.439580858552613751 ) ) ;
#20658=CARTESIAN_POINT ( 'NONE',  ( 12.62499999999998579, -20.24999999999999289, 3.666666666666653640 ) ) ;
#20659=CARTESIAN_POINT ( 'NONE',  ( 0.000000000000000000, -9.114917468222230923, 1.997643865078340797 ) ) ;
#20669=CARTESIAN_POINT ( 'NONE',  ( 3.232228556578340850, -13.29361487011126464, 2.695816835751057461 ) ) ;
#20675=CARTESIAN_POINT ( 'NONE',  ( -13.19432713877993812, -20.58564808021783321, 3.473490178816806662 ) ) ;
#20677=CARTESIAN_POINT ( 'NONE',  ( 4.003441417683175629, -22.05068747287766229, 4.499999999999999112 ) ) ;
#20678=CARTESIAN_POINT ( 'NONE',  ( -12.83635126708105823, -9.576761012430582198, 5.715524842913705328 ) ) ;
#20679=CARTESIAN_POINT ( 'NONE',  ( -12.43405858231679417, -23.20159541128345992, 4.773278322869455970 ) ) ;
#20681=CARTESIAN_POINT ( 'NONE',  ( -11.12844141768317741, -20.24999999999999289, 3.550687472877664952 ) ) ;
#20685=CARTESIAN_POINT ( 'NONE',  ( 13.08919463935856697, 3.941829287606363863, 5.256209690007596080 ) ) ;
#20694=CARTESIAN_POINT ( 'NONE',  ( 10.47219141768317741, -23.72900456129164937, 2.724438792969417378 ) ) ;
#20698=CARTESIAN_POINT ( 'NONE',  ( -3.162271481458107658, -13.95306990448253437, 3.615178062515473911 ) ) ;
#20700=CARTESIAN_POINT ( 'NONE',  ( -10.46530858231679417, -20.22900456129164937, 4.174186261275266929 ) ) ;
#20702=CARTESIAN_POINT ( 'NONE',  ( 8.784691417683177406, -24.52099543870834708, 4.484846433055073689 ) ) ;
#20704=CARTESIAN_POINT ( 'NONE',  ( -9.815941417683177406, -20.79840458871654363, 4.773278322869464851 ) ) ;
#20706=CARTESIAN_POINT ( 'NONE',  ( 7.840308582316794173, -22.67418626127525982, 5.270995438708342640 ) ) ;
#20709=CARTESIAN_POINT ( 'NONE',  ( -13.90439735423465351, 5.734566389025032684, 3.333333333332063386 ) ) ;
#20711=CARTESIAN_POINT ( 'NONE',  ( 5.777808582316794173, -20.27099543870833642, 2.724438792969431589 ) ) ;
#20716=( NAMED_UNIT ( * ) PLANE_ANGLE_UNIT ( ) SI_UNIT ( $, .RADIAN. ) );
#20719=CARTESIAN_POINT ( 'NONE',  ( 0.000000000000000000, -9.114917468222230923, 1.622643865078341019 ) ) ;
ENDSEC;
END-ISO-10303-21;
